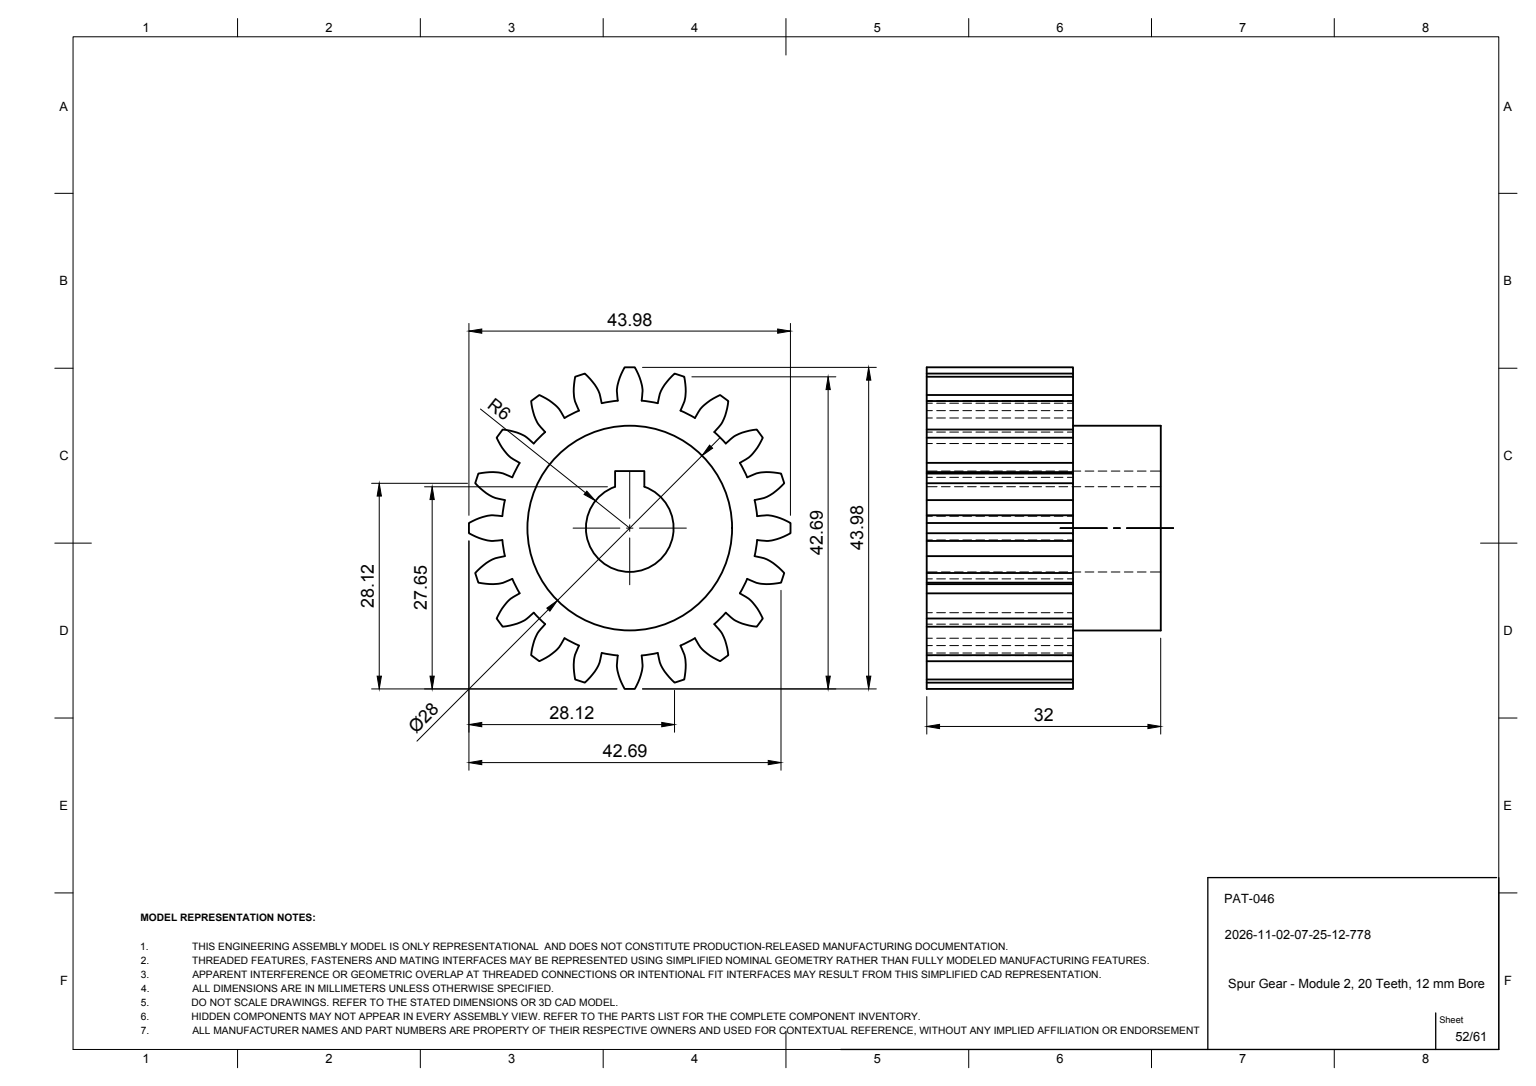
ISO-10303-21;
HEADER;
/* Generated by software containing ST-Developer
 * from STEP Tools, Inc. (www.steptools.com) 
 */

FILE_DESCRIPTION(
/* description */ ('Gear mesh backlash fixture'),
/* implementation_level */ '2;1');

FILE_NAME(
/* name */ 'Spur Gear - Module 2, 20 Teeth, 12 mm Bore.step',
/* time_stamp */ '2026-10-28T03:26:00-07:00',
/* author */ (''),
/* organization */ (''),
/* preprocessor_version */ 'ST-DEVELOPER v20.2',
/* originating_system */ 'Autodesk Translation Framework v15.17.0.0',
/* authorisation */ '');

FILE_SCHEMA (('AUTOMOTIVE_DESIGN { 1 0 10303 214 3 1 1 }'));
ENDSEC;

DATA;
#10=MECHANICAL_DESIGN_GEOMETRIC_PRESENTATION_REPRESENTATION('',(#1071),#57900);
#11=(
BOUNDED_SURFACE()
B_SPLINE_SURFACE(5,1,((#25176,#25177),(#25178,#25179),(#25180,#25181),(#25182,
#25183),(#25184,#25185),(#25186,#25187),(#25188,#25189),(#25190,#25191),
(#25192,#25193),(#25194,#25195),(#25196,#25197),(#25198,#25199),(#25200,
#25201),(#25202,#25203),(#25204,#25205),(#25206,#25207),(#25208,#25209),
(#25210,#25211),(#25212,#25213),(#25214,#25215),(#25216,#25217),(#25218,
#25219),(#25220,#25221),(#25222,#25223),(#25224,#25225),(#25226,#25227),
(#25228,#25229),(#25230,#25231),(#25232,#25233),(#25234,#25235),(#25236,
#25237),(#25238,#25239),(#25240,#25241),(#25242,#25243),(#25244,#25245),
(#25246,#25247),(#25248,#25249),(#25250,#25251),(#25252,#25253),(#25254,
#25255),(#25256,#25257),(#25258,#25259),(#25260,#25261),(#25262,#25263),
(#25264,#25265),(#25266,#25267),(#25268,#25269),(#25270,#25271),(#25272,
#25273),(#25274,#25275),(#25276,#25277),(#25278,#25279),(#25280,#25281),
(#25282,#25283),(#25284,#25285),(#25286,#25287),(#25288,#25289),(#25290,
#25291),(#25292,#25293),(#25294,#25295),(#25296,#25297),(#25298,#25299),
(#25300,#25301),(#25302,#25303),(#25304,#25305),(#25306,#25307),(#25308,
#25309),(#25310,#25311),(#25312,#25313),(#25314,#25315)),.UNSPECIFIED.,
 .F.,.F.,.F.)
B_SPLINE_SURFACE_WITH_KNOTS((6,1,1,1,1,1,1,1,1,1,1,1,1,1,1,1,1,1,1,1,1,
1,1,1,1,1,1,1,1,1,1,1,1,1,1,1,1,1,1,1,1,1,1,1,1,1,1,1,1,1,1,1,1,1,1,1,1,
1,1,1,1,1,1,1,1,6),(2,2),(-1.,-0.984615384615383,-0.969230769230768,-0.953846153846152,
-0.938461538461537,-0.923076923076922,-0.907692307692306,-0.892307692307691,
-0.876923076923076,-0.86153846153846,-0.846153846153845,-0.83076923076923,
-0.815384615384614,-0.799999999999999,-0.784615384615384,-0.769230769230768,
-0.753846153846153,-0.738461538461538,-0.723076923076922,-0.707692307692307,
-0.692307692307692,-0.676923076923076,-0.661538461538461,-0.646153846153846,
-0.63076923076923,-0.615384615384615,-0.6,-0.584615384615384,-0.569230769230769,
-0.553846153846154,-0.538461538461538,-0.523076923076923,-0.507692307692308,
-0.492307692307692,-0.476923076923077,-0.461538461538462,-0.446153846153846,
-0.430769230769231,-0.415384615384615,-0.4,-0.384615384615385,-0.369230769230769,
-0.353846153846154,-0.338461538461538,-0.323076923076923,-0.307692307692308,
-0.292307692307692,-0.276923076923077,-0.261538461538462,-0.246153846153846,
-0.230769230769231,-0.215384615384615,-0.2,-0.184615384615385,-0.169230769230769,
-0.153846153846154,-0.138461538461538,-0.123076923076923,-0.107692307692308,
-0.0923076923076923,-0.0769230769230769,-0.0615384615384615,-0.0461538461538462,
-0.0307692307692308,-0.0153846153846154,0.),(-1.,1.),.UNSPECIFIED.)
GEOMETRIC_REPRESENTATION_ITEM()
RATIONAL_B_SPLINE_SURFACE(((1.,1.),(1.,1.),(1.,1.),(1.,1.),(1.,1.),(1.,
1.),(1.,1.),(1.,1.),(1.,1.),(1.,1.),(1.,1.),(1.,1.),(1.,1.),(1.,1.),(1.,
1.),(1.,1.),(1.,1.),(1.,1.),(1.,1.),(1.,1.),(1.,1.),(1.,1.),(1.,1.),(1.,
1.),(1.,1.),(1.,1.),(1.,1.),(1.,1.),(1.,1.),(1.,1.),(1.,1.),(1.,1.),(1.,
1.),(1.,1.),(1.,1.),(1.,1.),(1.,1.),(1.,1.),(1.,1.),(1.,1.),(1.,1.),(1.,
1.),(1.,1.),(1.,1.),(1.,1.),(1.,1.),(1.,1.),(1.,1.),(1.,1.),(1.,1.),(1.,
1.),(1.,1.),(1.,1.),(1.,1.),(1.,1.),(1.,1.),(1.,1.),(1.,1.),(1.,1.),(1.,
1.),(1.,1.),(1.,1.),(1.,1.),(1.,1.),(1.,1.),(1.,1.),(1.,1.),(1.,1.),(1.,
1.),(1.,1.)))
REPRESENTATION_ITEM('')
SURFACE()
);
#12=(
BOUNDED_SURFACE()
B_SPLINE_SURFACE(5,1,((#25394,#25395),(#25396,#25397),(#25398,#25399),(#25400,
#25401),(#25402,#25403),(#25404,#25405),(#25406,#25407),(#25408,#25409),
(#25410,#25411),(#25412,#25413),(#25414,#25415),(#25416,#25417),(#25418,
#25419),(#25420,#25421),(#25422,#25423),(#25424,#25425),(#25426,#25427),
(#25428,#25429),(#25430,#25431),(#25432,#25433),(#25434,#25435),(#25436,
#25437),(#25438,#25439),(#25440,#25441),(#25442,#25443),(#25444,#25445),
(#25446,#25447),(#25448,#25449),(#25450,#25451),(#25452,#25453),(#25454,
#25455),(#25456,#25457),(#25458,#25459),(#25460,#25461),(#25462,#25463),
(#25464,#25465),(#25466,#25467),(#25468,#25469),(#25470,#25471),(#25472,
#25473),(#25474,#25475),(#25476,#25477),(#25478,#25479),(#25480,#25481),
(#25482,#25483),(#25484,#25485),(#25486,#25487),(#25488,#25489),(#25490,
#25491),(#25492,#25493),(#25494,#25495),(#25496,#25497),(#25498,#25499),
(#25500,#25501),(#25502,#25503),(#25504,#25505),(#25506,#25507),(#25508,
#25509),(#25510,#25511),(#25512,#25513),(#25514,#25515),(#25516,#25517),
(#25518,#25519),(#25520,#25521),(#25522,#25523),(#25524,#25525),(#25526,
#25527),(#25528,#25529),(#25530,#25531),(#25532,#25533)),.UNSPECIFIED.,
 .F.,.F.,.F.)
B_SPLINE_SURFACE_WITH_KNOTS((6,1,1,1,1,1,1,1,1,1,1,1,1,1,1,1,1,1,1,1,1,
1,1,1,1,1,1,1,1,1,1,1,1,1,1,1,1,1,1,1,1,1,1,1,1,1,1,1,1,1,1,1,1,1,1,1,1,
1,1,1,1,1,1,1,1,6),(2,2),(-1.,-0.984615384615383,-0.969230769230768,-0.953846153846152,
-0.938461538461537,-0.923076923076922,-0.907692307692306,-0.892307692307691,
-0.876923076923076,-0.86153846153846,-0.846153846153845,-0.83076923076923,
-0.815384615384614,-0.799999999999999,-0.784615384615384,-0.769230769230768,
-0.753846153846153,-0.738461538461538,-0.723076923076922,-0.707692307692307,
-0.692307692307692,-0.676923076923076,-0.661538461538461,-0.646153846153846,
-0.63076923076923,-0.615384615384615,-0.6,-0.584615384615384,-0.569230769230769,
-0.553846153846154,-0.538461538461538,-0.523076923076923,-0.507692307692308,
-0.492307692307692,-0.476923076923077,-0.461538461538462,-0.446153846153846,
-0.430769230769231,-0.415384615384615,-0.4,-0.384615384615385,-0.369230769230769,
-0.353846153846154,-0.338461538461538,-0.323076923076923,-0.307692307692308,
-0.292307692307692,-0.276923076923077,-0.261538461538462,-0.246153846153846,
-0.230769230769231,-0.215384615384615,-0.2,-0.184615384615385,-0.169230769230769,
-0.153846153846154,-0.138461538461538,-0.123076923076923,-0.107692307692308,
-0.0923076923076923,-0.0769230769230769,-0.0615384615384615,-0.0461538461538462,
-0.0307692307692308,-0.0153846153846154,0.),(-1.,1.),.UNSPECIFIED.)
GEOMETRIC_REPRESENTATION_ITEM()
RATIONAL_B_SPLINE_SURFACE(((1.,1.),(1.,1.),(1.,1.),(1.,1.),(1.,1.),(1.,
1.),(1.,1.),(1.,1.),(1.,1.),(1.,1.),(1.,1.),(1.,1.),(1.,1.),(1.,1.),(1.,
1.),(1.,1.),(1.,1.),(1.,1.),(1.,1.),(1.,1.),(1.,1.),(1.,1.),(1.,1.),(1.,
1.),(1.,1.),(1.,1.),(1.,1.),(1.,1.),(1.,1.),(1.,1.),(1.,1.),(1.,1.),(1.,
1.),(1.,1.),(1.,1.),(1.,1.),(1.,1.),(1.,1.),(1.,1.),(1.,1.),(1.,1.),(1.,
1.),(1.,1.),(1.,1.),(1.,1.),(1.,1.),(1.,1.),(1.,1.),(1.,1.),(1.,1.),(1.,
1.),(1.,1.),(1.,1.),(1.,1.),(1.,1.),(1.,1.),(1.,1.),(1.,1.),(1.,1.),(1.,
1.),(1.,1.),(1.,1.),(1.,1.),(1.,1.),(1.,1.),(1.,1.),(1.,1.),(1.,1.),(1.,
1.),(1.,1.)))
REPRESENTATION_ITEM('')
SURFACE()
);
#13=(
BOUNDED_SURFACE()
B_SPLINE_SURFACE(5,1,((#25610,#25611),(#25612,#25613),(#25614,#25615),(#25616,
#25617),(#25618,#25619),(#25620,#25621),(#25622,#25623),(#25624,#25625),
(#25626,#25627),(#25628,#25629),(#25630,#25631),(#25632,#25633),(#25634,
#25635),(#25636,#25637),(#25638,#25639),(#25640,#25641),(#25642,#25643),
(#25644,#25645),(#25646,#25647),(#25648,#25649),(#25650,#25651),(#25652,
#25653),(#25654,#25655),(#25656,#25657),(#25658,#25659),(#25660,#25661),
(#25662,#25663),(#25664,#25665),(#25666,#25667),(#25668,#25669),(#25670,
#25671),(#25672,#25673),(#25674,#25675),(#25676,#25677),(#25678,#25679),
(#25680,#25681),(#25682,#25683),(#25684,#25685),(#25686,#25687),(#25688,
#25689),(#25690,#25691),(#25692,#25693),(#25694,#25695),(#25696,#25697),
(#25698,#25699),(#25700,#25701),(#25702,#25703),(#25704,#25705),(#25706,
#25707),(#25708,#25709),(#25710,#25711),(#25712,#25713),(#25714,#25715),
(#25716,#25717),(#25718,#25719),(#25720,#25721),(#25722,#25723),(#25724,
#25725),(#25726,#25727),(#25728,#25729),(#25730,#25731),(#25732,#25733),
(#25734,#25735),(#25736,#25737),(#25738,#25739),(#25740,#25741),(#25742,
#25743),(#25744,#25745),(#25746,#25747),(#25748,#25749)),.UNSPECIFIED.,
 .F.,.F.,.F.)
B_SPLINE_SURFACE_WITH_KNOTS((6,1,1,1,1,1,1,1,1,1,1,1,1,1,1,1,1,1,1,1,1,
1,1,1,1,1,1,1,1,1,1,1,1,1,1,1,1,1,1,1,1,1,1,1,1,1,1,1,1,1,1,1,1,1,1,1,1,
1,1,1,1,1,1,1,1,6),(2,2),(-1.,-0.984615384615383,-0.969230769230768,-0.953846153846152,
-0.938461538461537,-0.923076923076922,-0.907692307692306,-0.892307692307691,
-0.876923076923076,-0.86153846153846,-0.846153846153845,-0.83076923076923,
-0.815384615384614,-0.799999999999999,-0.784615384615384,-0.769230769230768,
-0.753846153846153,-0.738461538461538,-0.723076923076922,-0.707692307692307,
-0.692307692307692,-0.676923076923076,-0.661538461538461,-0.646153846153846,
-0.63076923076923,-0.615384615384615,-0.6,-0.584615384615384,-0.569230769230769,
-0.553846153846154,-0.538461538461538,-0.523076923076923,-0.507692307692308,
-0.492307692307692,-0.476923076923077,-0.461538461538462,-0.446153846153846,
-0.430769230769231,-0.415384615384615,-0.4,-0.384615384615385,-0.369230769230769,
-0.353846153846154,-0.338461538461538,-0.323076923076923,-0.307692307692308,
-0.292307692307692,-0.276923076923077,-0.261538461538462,-0.246153846153846,
-0.230769230769231,-0.215384615384615,-0.2,-0.184615384615385,-0.169230769230769,
-0.153846153846154,-0.138461538461538,-0.123076923076923,-0.107692307692308,
-0.0923076923076923,-0.0769230769230769,-0.0615384615384615,-0.0461538461538462,
-0.0307692307692308,-0.0153846153846154,0.),(-1.,1.),.UNSPECIFIED.)
GEOMETRIC_REPRESENTATION_ITEM()
RATIONAL_B_SPLINE_SURFACE(((1.,1.),(1.,1.),(1.,1.),(1.,1.),(1.,1.),(1.,
1.),(1.,1.),(1.,1.),(1.,1.),(1.,1.),(1.,1.),(1.,1.),(1.,1.),(1.,1.),(1.,
1.),(1.,1.),(1.,1.),(1.,1.),(1.,1.),(1.,1.),(1.,1.),(1.,1.),(1.,1.),(1.,
1.),(1.,1.),(1.,1.),(1.,1.),(1.,1.),(1.,1.),(1.,1.),(1.,1.),(1.,1.),(1.,
1.),(1.,1.),(1.,1.),(1.,1.),(1.,1.),(1.,1.),(1.,1.),(1.,1.),(1.,1.),(1.,
1.),(1.,1.),(1.,1.),(1.,1.),(1.,1.),(1.,1.),(1.,1.),(1.,1.),(1.,1.),(1.,
1.),(1.,1.),(1.,1.),(1.,1.),(1.,1.),(1.,1.),(1.,1.),(1.,1.),(1.,1.),(1.,
1.),(1.,1.),(1.,1.),(1.,1.),(1.,1.),(1.,1.),(1.,1.),(1.,1.),(1.,1.),(1.,
1.),(1.,1.)))
REPRESENTATION_ITEM('')
SURFACE()
);
#14=(
BOUNDED_SURFACE()
B_SPLINE_SURFACE(5,1,((#25826,#25827),(#25828,#25829),(#25830,#25831),(#25832,
#25833),(#25834,#25835),(#25836,#25837),(#25838,#25839),(#25840,#25841),
(#25842,#25843),(#25844,#25845),(#25846,#25847),(#25848,#25849),(#25850,
#25851),(#25852,#25853),(#25854,#25855),(#25856,#25857),(#25858,#25859),
(#25860,#25861),(#25862,#25863),(#25864,#25865),(#25866,#25867),(#25868,
#25869),(#25870,#25871),(#25872,#25873),(#25874,#25875),(#25876,#25877),
(#25878,#25879),(#25880,#25881),(#25882,#25883),(#25884,#25885),(#25886,
#25887),(#25888,#25889),(#25890,#25891),(#25892,#25893),(#25894,#25895),
(#25896,#25897),(#25898,#25899),(#25900,#25901),(#25902,#25903),(#25904,
#25905),(#25906,#25907),(#25908,#25909),(#25910,#25911),(#25912,#25913),
(#25914,#25915),(#25916,#25917),(#25918,#25919),(#25920,#25921),(#25922,
#25923),(#25924,#25925),(#25926,#25927),(#25928,#25929),(#25930,#25931),
(#25932,#25933),(#25934,#25935),(#25936,#25937),(#25938,#25939),(#25940,
#25941),(#25942,#25943),(#25944,#25945),(#25946,#25947),(#25948,#25949),
(#25950,#25951),(#25952,#25953),(#25954,#25955),(#25956,#25957),(#25958,
#25959),(#25960,#25961),(#25962,#25963),(#25964,#25965)),.UNSPECIFIED.,
 .F.,.F.,.F.)
B_SPLINE_SURFACE_WITH_KNOTS((6,1,1,1,1,1,1,1,1,1,1,1,1,1,1,1,1,1,1,1,1,
1,1,1,1,1,1,1,1,1,1,1,1,1,1,1,1,1,1,1,1,1,1,1,1,1,1,1,1,1,1,1,1,1,1,1,1,
1,1,1,1,1,1,1,1,6),(2,2),(-1.,-0.984615384615383,-0.969230769230768,-0.953846153846152,
-0.938461538461537,-0.923076923076922,-0.907692307692306,-0.892307692307691,
-0.876923076923076,-0.86153846153846,-0.846153846153845,-0.83076923076923,
-0.815384615384614,-0.799999999999999,-0.784615384615384,-0.769230769230768,
-0.753846153846153,-0.738461538461538,-0.723076923076922,-0.707692307692307,
-0.692307692307692,-0.676923076923076,-0.661538461538461,-0.646153846153846,
-0.63076923076923,-0.615384615384615,-0.6,-0.584615384615384,-0.569230769230769,
-0.553846153846154,-0.538461538461538,-0.523076923076923,-0.507692307692308,
-0.492307692307692,-0.476923076923077,-0.461538461538462,-0.446153846153846,
-0.430769230769231,-0.415384615384615,-0.4,-0.384615384615385,-0.369230769230769,
-0.353846153846154,-0.338461538461538,-0.323076923076923,-0.307692307692308,
-0.292307692307692,-0.276923076923077,-0.261538461538462,-0.246153846153846,
-0.230769230769231,-0.215384615384615,-0.2,-0.184615384615385,-0.169230769230769,
-0.153846153846154,-0.138461538461538,-0.123076923076923,-0.107692307692308,
-0.0923076923076923,-0.0769230769230769,-0.0615384615384615,-0.0461538461538462,
-0.0307692307692308,-0.0153846153846154,0.),(-1.,1.),.UNSPECIFIED.)
GEOMETRIC_REPRESENTATION_ITEM()
RATIONAL_B_SPLINE_SURFACE(((1.,1.),(1.,1.),(1.,1.),(1.,1.),(1.,1.),(1.,
1.),(1.,1.),(1.,1.),(1.,1.),(1.,1.),(1.,1.),(1.,1.),(1.,1.),(1.,1.),(1.,
1.),(1.,1.),(1.,1.),(1.,1.),(1.,1.),(1.,1.),(1.,1.),(1.,1.),(1.,1.),(1.,
1.),(1.,1.),(1.,1.),(1.,1.),(1.,1.),(1.,1.),(1.,1.),(1.,1.),(1.,1.),(1.,
1.),(1.,1.),(1.,1.),(1.,1.),(1.,1.),(1.,1.),(1.,1.),(1.,1.),(1.,1.),(1.,
1.),(1.,1.),(1.,1.),(1.,1.),(1.,1.),(1.,1.),(1.,1.),(1.,1.),(1.,1.),(1.,
1.),(1.,1.),(1.,1.),(1.,1.),(1.,1.),(1.,1.),(1.,1.),(1.,1.),(1.,1.),(1.,
1.),(1.,1.),(1.,1.),(1.,1.),(1.,1.),(1.,1.),(1.,1.),(1.,1.),(1.,1.),(1.,
1.),(1.,1.)))
REPRESENTATION_ITEM('')
SURFACE()
);
#15=(
BOUNDED_SURFACE()
B_SPLINE_SURFACE(5,1,((#26042,#26043),(#26044,#26045),(#26046,#26047),(#26048,
#26049),(#26050,#26051),(#26052,#26053),(#26054,#26055),(#26056,#26057),
(#26058,#26059),(#26060,#26061),(#26062,#26063),(#26064,#26065),(#26066,
#26067),(#26068,#26069),(#26070,#26071),(#26072,#26073),(#26074,#26075),
(#26076,#26077),(#26078,#26079),(#26080,#26081),(#26082,#26083),(#26084,
#26085),(#26086,#26087),(#26088,#26089),(#26090,#26091),(#26092,#26093),
(#26094,#26095),(#26096,#26097),(#26098,#26099),(#26100,#26101),(#26102,
#26103),(#26104,#26105),(#26106,#26107),(#26108,#26109),(#26110,#26111),
(#26112,#26113),(#26114,#26115),(#26116,#26117),(#26118,#26119),(#26120,
#26121),(#26122,#26123),(#26124,#26125),(#26126,#26127),(#26128,#26129),
(#26130,#26131),(#26132,#26133),(#26134,#26135),(#26136,#26137),(#26138,
#26139),(#26140,#26141),(#26142,#26143),(#26144,#26145),(#26146,#26147),
(#26148,#26149),(#26150,#26151),(#26152,#26153),(#26154,#26155),(#26156,
#26157),(#26158,#26159),(#26160,#26161),(#26162,#26163),(#26164,#26165),
(#26166,#26167),(#26168,#26169),(#26170,#26171),(#26172,#26173),(#26174,
#26175),(#26176,#26177),(#26178,#26179),(#26180,#26181)),.UNSPECIFIED.,
 .F.,.F.,.F.)
B_SPLINE_SURFACE_WITH_KNOTS((6,1,1,1,1,1,1,1,1,1,1,1,1,1,1,1,1,1,1,1,1,
1,1,1,1,1,1,1,1,1,1,1,1,1,1,1,1,1,1,1,1,1,1,1,1,1,1,1,1,1,1,1,1,1,1,1,1,
1,1,1,1,1,1,1,1,6),(2,2),(-1.,-0.984615384615383,-0.969230769230768,-0.953846153846152,
-0.938461538461537,-0.923076923076922,-0.907692307692306,-0.892307692307691,
-0.876923076923076,-0.86153846153846,-0.846153846153845,-0.83076923076923,
-0.815384615384614,-0.799999999999999,-0.784615384615384,-0.769230769230768,
-0.753846153846153,-0.738461538461538,-0.723076923076922,-0.707692307692307,
-0.692307692307692,-0.676923076923076,-0.661538461538461,-0.646153846153846,
-0.63076923076923,-0.615384615384615,-0.6,-0.584615384615384,-0.569230769230769,
-0.553846153846154,-0.538461538461538,-0.523076923076923,-0.507692307692308,
-0.492307692307692,-0.476923076923077,-0.461538461538462,-0.446153846153846,
-0.430769230769231,-0.415384615384615,-0.4,-0.384615384615385,-0.369230769230769,
-0.353846153846154,-0.338461538461538,-0.323076923076923,-0.307692307692308,
-0.292307692307692,-0.276923076923077,-0.261538461538462,-0.246153846153846,
-0.230769230769231,-0.215384615384615,-0.2,-0.184615384615385,-0.169230769230769,
-0.153846153846154,-0.138461538461538,-0.123076923076923,-0.107692307692308,
-0.0923076923076923,-0.0769230769230769,-0.0615384615384615,-0.0461538461538462,
-0.0307692307692308,-0.0153846153846154,0.),(-1.,1.),.UNSPECIFIED.)
GEOMETRIC_REPRESENTATION_ITEM()
RATIONAL_B_SPLINE_SURFACE(((1.,1.),(1.,1.),(1.,1.),(1.,1.),(1.,1.),(1.,
1.),(1.,1.),(1.,1.),(1.,1.),(1.,1.),(1.,1.),(1.,1.),(1.,1.),(1.,1.),(1.,
1.),(1.,1.),(1.,1.),(1.,1.),(1.,1.),(1.,1.),(1.,1.),(1.,1.),(1.,1.),(1.,
1.),(1.,1.),(1.,1.),(1.,1.),(1.,1.),(1.,1.),(1.,1.),(1.,1.),(1.,1.),(1.,
1.),(1.,1.),(1.,1.),(1.,1.),(1.,1.),(1.,1.),(1.,1.),(1.,1.),(1.,1.),(1.,
1.),(1.,1.),(1.,1.),(1.,1.),(1.,1.),(1.,1.),(1.,1.),(1.,1.),(1.,1.),(1.,
1.),(1.,1.),(1.,1.),(1.,1.),(1.,1.),(1.,1.),(1.,1.),(1.,1.),(1.,1.),(1.,
1.),(1.,1.),(1.,1.),(1.,1.),(1.,1.),(1.,1.),(1.,1.),(1.,1.),(1.,1.),(1.,
1.),(1.,1.)))
REPRESENTATION_ITEM('')
SURFACE()
);
#16=(
BOUNDED_SURFACE()
B_SPLINE_SURFACE(5,1,((#26258,#26259),(#26260,#26261),(#26262,#26263),(#26264,
#26265),(#26266,#26267),(#26268,#26269),(#26270,#26271),(#26272,#26273),
(#26274,#26275),(#26276,#26277),(#26278,#26279),(#26280,#26281),(#26282,
#26283),(#26284,#26285),(#26286,#26287),(#26288,#26289),(#26290,#26291),
(#26292,#26293),(#26294,#26295),(#26296,#26297),(#26298,#26299),(#26300,
#26301),(#26302,#26303),(#26304,#26305),(#26306,#26307),(#26308,#26309),
(#26310,#26311),(#26312,#26313),(#26314,#26315),(#26316,#26317),(#26318,
#26319),(#26320,#26321),(#26322,#26323),(#26324,#26325),(#26326,#26327),
(#26328,#26329),(#26330,#26331),(#26332,#26333),(#26334,#26335),(#26336,
#26337),(#26338,#26339),(#26340,#26341),(#26342,#26343),(#26344,#26345),
(#26346,#26347),(#26348,#26349),(#26350,#26351),(#26352,#26353),(#26354,
#26355),(#26356,#26357),(#26358,#26359),(#26360,#26361),(#26362,#26363),
(#26364,#26365),(#26366,#26367),(#26368,#26369),(#26370,#26371),(#26372,
#26373),(#26374,#26375),(#26376,#26377),(#26378,#26379),(#26380,#26381),
(#26382,#26383),(#26384,#26385),(#26386,#26387),(#26388,#26389),(#26390,
#26391),(#26392,#26393),(#26394,#26395),(#26396,#26397)),.UNSPECIFIED.,
 .F.,.F.,.F.)
B_SPLINE_SURFACE_WITH_KNOTS((6,1,1,1,1,1,1,1,1,1,1,1,1,1,1,1,1,1,1,1,1,
1,1,1,1,1,1,1,1,1,1,1,1,1,1,1,1,1,1,1,1,1,1,1,1,1,1,1,1,1,1,1,1,1,1,1,1,
1,1,1,1,1,1,1,1,6),(2,2),(-1.,-0.984615384615383,-0.969230769230768,-0.953846153846152,
-0.938461538461537,-0.923076923076922,-0.907692307692306,-0.892307692307691,
-0.876923076923076,-0.86153846153846,-0.846153846153845,-0.83076923076923,
-0.815384615384614,-0.799999999999999,-0.784615384615384,-0.769230769230768,
-0.753846153846153,-0.738461538461538,-0.723076923076922,-0.707692307692307,
-0.692307692307692,-0.676923076923076,-0.661538461538461,-0.646153846153846,
-0.63076923076923,-0.615384615384615,-0.6,-0.584615384615384,-0.569230769230769,
-0.553846153846154,-0.538461538461538,-0.523076923076923,-0.507692307692308,
-0.492307692307692,-0.476923076923077,-0.461538461538462,-0.446153846153846,
-0.430769230769231,-0.415384615384615,-0.4,-0.384615384615385,-0.369230769230769,
-0.353846153846154,-0.338461538461538,-0.323076923076923,-0.307692307692308,
-0.292307692307692,-0.276923076923077,-0.261538461538462,-0.246153846153846,
-0.230769230769231,-0.215384615384615,-0.2,-0.184615384615385,-0.169230769230769,
-0.153846153846154,-0.138461538461538,-0.123076923076923,-0.107692307692308,
-0.0923076923076923,-0.0769230769230769,-0.0615384615384615,-0.0461538461538462,
-0.0307692307692308,-0.0153846153846154,0.),(-1.,1.),.UNSPECIFIED.)
GEOMETRIC_REPRESENTATION_ITEM()
RATIONAL_B_SPLINE_SURFACE(((1.,1.),(1.,1.),(1.,1.),(1.,1.),(1.,1.),(1.,
1.),(1.,1.),(1.,1.),(1.,1.),(1.,1.),(1.,1.),(1.,1.),(1.,1.),(1.,1.),(1.,
1.),(1.,1.),(1.,1.),(1.,1.),(1.,1.),(1.,1.),(1.,1.),(1.,1.),(1.,1.),(1.,
1.),(1.,1.),(1.,1.),(1.,1.),(1.,1.),(1.,1.),(1.,1.),(1.,1.),(1.,1.),(1.,
1.),(1.,1.),(1.,1.),(1.,1.),(1.,1.),(1.,1.),(1.,1.),(1.,1.),(1.,1.),(1.,
1.),(1.,1.),(1.,1.),(1.,1.),(1.,1.),(1.,1.),(1.,1.),(1.,1.),(1.,1.),(1.,
1.),(1.,1.),(1.,1.),(1.,1.),(1.,1.),(1.,1.),(1.,1.),(1.,1.),(1.,1.),(1.,
1.),(1.,1.),(1.,1.),(1.,1.),(1.,1.),(1.,1.),(1.,1.),(1.,1.),(1.,1.),(1.,
1.),(1.,1.)))
REPRESENTATION_ITEM('')
SURFACE()
);
#17=(
BOUNDED_SURFACE()
B_SPLINE_SURFACE(5,1,((#26474,#26475),(#26476,#26477),(#26478,#26479),(#26480,
#26481),(#26482,#26483),(#26484,#26485),(#26486,#26487),(#26488,#26489),
(#26490,#26491),(#26492,#26493),(#26494,#26495),(#26496,#26497),(#26498,
#26499),(#26500,#26501),(#26502,#26503),(#26504,#26505),(#26506,#26507),
(#26508,#26509),(#26510,#26511),(#26512,#26513),(#26514,#26515),(#26516,
#26517),(#26518,#26519),(#26520,#26521),(#26522,#26523),(#26524,#26525),
(#26526,#26527),(#26528,#26529),(#26530,#26531),(#26532,#26533),(#26534,
#26535),(#26536,#26537),(#26538,#26539),(#26540,#26541),(#26542,#26543),
(#26544,#26545),(#26546,#26547),(#26548,#26549),(#26550,#26551),(#26552,
#26553),(#26554,#26555),(#26556,#26557),(#26558,#26559),(#26560,#26561),
(#26562,#26563),(#26564,#26565),(#26566,#26567),(#26568,#26569),(#26570,
#26571),(#26572,#26573),(#26574,#26575),(#26576,#26577),(#26578,#26579),
(#26580,#26581),(#26582,#26583),(#26584,#26585),(#26586,#26587),(#26588,
#26589),(#26590,#26591),(#26592,#26593),(#26594,#26595),(#26596,#26597),
(#26598,#26599),(#26600,#26601),(#26602,#26603),(#26604,#26605),(#26606,
#26607),(#26608,#26609),(#26610,#26611),(#26612,#26613)),.UNSPECIFIED.,
 .F.,.F.,.F.)
B_SPLINE_SURFACE_WITH_KNOTS((6,1,1,1,1,1,1,1,1,1,1,1,1,1,1,1,1,1,1,1,1,
1,1,1,1,1,1,1,1,1,1,1,1,1,1,1,1,1,1,1,1,1,1,1,1,1,1,1,1,1,1,1,1,1,1,1,1,
1,1,1,1,1,1,1,1,6),(2,2),(-1.,-0.984615384615383,-0.969230769230768,-0.953846153846152,
-0.938461538461537,-0.923076923076922,-0.907692307692306,-0.892307692307691,
-0.876923076923076,-0.86153846153846,-0.846153846153845,-0.83076923076923,
-0.815384615384614,-0.799999999999999,-0.784615384615384,-0.769230769230768,
-0.753846153846153,-0.738461538461538,-0.723076923076922,-0.707692307692307,
-0.692307692307692,-0.676923076923076,-0.661538461538461,-0.646153846153846,
-0.63076923076923,-0.615384615384615,-0.6,-0.584615384615384,-0.569230769230769,
-0.553846153846154,-0.538461538461538,-0.523076923076923,-0.507692307692308,
-0.492307692307692,-0.476923076923077,-0.461538461538462,-0.446153846153846,
-0.430769230769231,-0.415384615384615,-0.4,-0.384615384615385,-0.369230769230769,
-0.353846153846154,-0.338461538461538,-0.323076923076923,-0.307692307692308,
-0.292307692307692,-0.276923076923077,-0.261538461538462,-0.246153846153846,
-0.230769230769231,-0.215384615384615,-0.2,-0.184615384615385,-0.169230769230769,
-0.153846153846154,-0.138461538461538,-0.123076923076923,-0.107692307692308,
-0.0923076923076923,-0.0769230769230769,-0.0615384615384615,-0.0461538461538462,
-0.0307692307692308,-0.0153846153846154,0.),(-1.,1.),.UNSPECIFIED.)
GEOMETRIC_REPRESENTATION_ITEM()
RATIONAL_B_SPLINE_SURFACE(((1.,1.),(1.,1.),(1.,1.),(1.,1.),(1.,1.),(1.,
1.),(1.,1.),(1.,1.),(1.,1.),(1.,1.),(1.,1.),(1.,1.),(1.,1.),(1.,1.),(1.,
1.),(1.,1.),(1.,1.),(1.,1.),(1.,1.),(1.,1.),(1.,1.),(1.,1.),(1.,1.),(1.,
1.),(1.,1.),(1.,1.),(1.,1.),(1.,1.),(1.,1.),(1.,1.),(1.,1.),(1.,1.),(1.,
1.),(1.,1.),(1.,1.),(1.,1.),(1.,1.),(1.,1.),(1.,1.),(1.,1.),(1.,1.),(1.,
1.),(1.,1.),(1.,1.),(1.,1.),(1.,1.),(1.,1.),(1.,1.),(1.,1.),(1.,1.),(1.,
1.),(1.,1.),(1.,1.),(1.,1.),(1.,1.),(1.,1.),(1.,1.),(1.,1.),(1.,1.),(1.,
1.),(1.,1.),(1.,1.),(1.,1.),(1.,1.),(1.,1.),(1.,1.),(1.,1.),(1.,1.),(1.,
1.),(1.,1.)))
REPRESENTATION_ITEM('')
SURFACE()
);
#18=(
BOUNDED_SURFACE()
B_SPLINE_SURFACE(5,1,((#26690,#26691),(#26692,#26693),(#26694,#26695),(#26696,
#26697),(#26698,#26699),(#26700,#26701),(#26702,#26703),(#26704,#26705),
(#26706,#26707),(#26708,#26709),(#26710,#26711),(#26712,#26713),(#26714,
#26715),(#26716,#26717),(#26718,#26719),(#26720,#26721),(#26722,#26723),
(#26724,#26725),(#26726,#26727),(#26728,#26729),(#26730,#26731),(#26732,
#26733),(#26734,#26735),(#26736,#26737),(#26738,#26739),(#26740,#26741),
(#26742,#26743),(#26744,#26745),(#26746,#26747),(#26748,#26749),(#26750,
#26751),(#26752,#26753),(#26754,#26755),(#26756,#26757),(#26758,#26759),
(#26760,#26761),(#26762,#26763),(#26764,#26765),(#26766,#26767),(#26768,
#26769),(#26770,#26771),(#26772,#26773),(#26774,#26775),(#26776,#26777),
(#26778,#26779),(#26780,#26781),(#26782,#26783),(#26784,#26785),(#26786,
#26787),(#26788,#26789),(#26790,#26791),(#26792,#26793),(#26794,#26795),
(#26796,#26797),(#26798,#26799),(#26800,#26801),(#26802,#26803),(#26804,
#26805),(#26806,#26807),(#26808,#26809),(#26810,#26811),(#26812,#26813),
(#26814,#26815),(#26816,#26817),(#26818,#26819),(#26820,#26821),(#26822,
#26823),(#26824,#26825),(#26826,#26827),(#26828,#26829)),.UNSPECIFIED.,
 .F.,.F.,.F.)
B_SPLINE_SURFACE_WITH_KNOTS((6,1,1,1,1,1,1,1,1,1,1,1,1,1,1,1,1,1,1,1,1,
1,1,1,1,1,1,1,1,1,1,1,1,1,1,1,1,1,1,1,1,1,1,1,1,1,1,1,1,1,1,1,1,1,1,1,1,
1,1,1,1,1,1,1,1,6),(2,2),(-1.,-0.984615384615383,-0.969230769230768,-0.953846153846152,
-0.938461538461537,-0.923076923076922,-0.907692307692306,-0.892307692307691,
-0.876923076923076,-0.86153846153846,-0.846153846153845,-0.83076923076923,
-0.815384615384614,-0.799999999999999,-0.784615384615384,-0.769230769230768,
-0.753846153846153,-0.738461538461538,-0.723076923076922,-0.707692307692307,
-0.692307692307692,-0.676923076923076,-0.661538461538461,-0.646153846153846,
-0.63076923076923,-0.615384615384615,-0.6,-0.584615384615384,-0.569230769230769,
-0.553846153846154,-0.538461538461538,-0.523076923076923,-0.507692307692308,
-0.492307692307692,-0.476923076923077,-0.461538461538462,-0.446153846153846,
-0.430769230769231,-0.415384615384615,-0.4,-0.384615384615385,-0.369230769230769,
-0.353846153846154,-0.338461538461538,-0.323076923076923,-0.307692307692308,
-0.292307692307692,-0.276923076923077,-0.261538461538462,-0.246153846153846,
-0.230769230769231,-0.215384615384615,-0.2,-0.184615384615385,-0.169230769230769,
-0.153846153846154,-0.138461538461538,-0.123076923076923,-0.107692307692308,
-0.0923076923076923,-0.0769230769230769,-0.0615384615384615,-0.0461538461538462,
-0.0307692307692308,-0.0153846153846154,0.),(-1.,1.),.UNSPECIFIED.)
GEOMETRIC_REPRESENTATION_ITEM()
RATIONAL_B_SPLINE_SURFACE(((1.,1.),(1.,1.),(1.,1.),(1.,1.),(1.,1.),(1.,
1.),(1.,1.),(1.,1.),(1.,1.),(1.,1.),(1.,1.),(1.,1.),(1.,1.),(1.,1.),(1.,
1.),(1.,1.),(1.,1.),(1.,1.),(1.,1.),(1.,1.),(1.,1.),(1.,1.),(1.,1.),(1.,
1.),(1.,1.),(1.,1.),(1.,1.),(1.,1.),(1.,1.),(1.,1.),(1.,1.),(1.,1.),(1.,
1.),(1.,1.),(1.,1.),(1.,1.),(1.,1.),(1.,1.),(1.,1.),(1.,1.),(1.,1.),(1.,
1.),(1.,1.),(1.,1.),(1.,1.),(1.,1.),(1.,1.),(1.,1.),(1.,1.),(1.,1.),(1.,
1.),(1.,1.),(1.,1.),(1.,1.),(1.,1.),(1.,1.),(1.,1.),(1.,1.),(1.,1.),(1.,
1.),(1.,1.),(1.,1.),(1.,1.),(1.,1.),(1.,1.),(1.,1.),(1.,1.),(1.,1.),(1.,
1.),(1.,1.)))
REPRESENTATION_ITEM('')
SURFACE()
);
#19=(
BOUNDED_SURFACE()
B_SPLINE_SURFACE(5,1,((#26906,#26907),(#26908,#26909),(#26910,#26911),(#26912,
#26913),(#26914,#26915),(#26916,#26917),(#26918,#26919),(#26920,#26921),
(#26922,#26923),(#26924,#26925),(#26926,#26927),(#26928,#26929),(#26930,
#26931),(#26932,#26933),(#26934,#26935),(#26936,#26937),(#26938,#26939),
(#26940,#26941),(#26942,#26943),(#26944,#26945),(#26946,#26947),(#26948,
#26949),(#26950,#26951),(#26952,#26953),(#26954,#26955),(#26956,#26957),
(#26958,#26959),(#26960,#26961),(#26962,#26963),(#26964,#26965),(#26966,
#26967),(#26968,#26969),(#26970,#26971),(#26972,#26973),(#26974,#26975),
(#26976,#26977),(#26978,#26979),(#26980,#26981),(#26982,#26983),(#26984,
#26985),(#26986,#26987),(#26988,#26989),(#26990,#26991),(#26992,#26993),
(#26994,#26995),(#26996,#26997),(#26998,#26999),(#27000,#27001),(#27002,
#27003),(#27004,#27005),(#27006,#27007),(#27008,#27009),(#27010,#27011),
(#27012,#27013),(#27014,#27015),(#27016,#27017),(#27018,#27019),(#27020,
#27021),(#27022,#27023),(#27024,#27025),(#27026,#27027),(#27028,#27029),
(#27030,#27031),(#27032,#27033),(#27034,#27035),(#27036,#27037),(#27038,
#27039),(#27040,#27041),(#27042,#27043),(#27044,#27045)),.UNSPECIFIED.,
 .F.,.F.,.F.)
B_SPLINE_SURFACE_WITH_KNOTS((6,1,1,1,1,1,1,1,1,1,1,1,1,1,1,1,1,1,1,1,1,
1,1,1,1,1,1,1,1,1,1,1,1,1,1,1,1,1,1,1,1,1,1,1,1,1,1,1,1,1,1,1,1,1,1,1,1,
1,1,1,1,1,1,1,1,6),(2,2),(-1.,-0.984615384615383,-0.969230769230768,-0.953846153846152,
-0.938461538461537,-0.923076923076922,-0.907692307692306,-0.892307692307691,
-0.876923076923076,-0.86153846153846,-0.846153846153845,-0.83076923076923,
-0.815384615384614,-0.799999999999999,-0.784615384615384,-0.769230769230768,
-0.753846153846153,-0.738461538461538,-0.723076923076922,-0.707692307692307,
-0.692307692307692,-0.676923076923076,-0.661538461538461,-0.646153846153846,
-0.63076923076923,-0.615384615384615,-0.6,-0.584615384615384,-0.569230769230769,
-0.553846153846154,-0.538461538461538,-0.523076923076923,-0.507692307692308,
-0.492307692307692,-0.476923076923077,-0.461538461538462,-0.446153846153846,
-0.430769230769231,-0.415384615384615,-0.4,-0.384615384615385,-0.369230769230769,
-0.353846153846154,-0.338461538461538,-0.323076923076923,-0.307692307692308,
-0.292307692307692,-0.276923076923077,-0.261538461538462,-0.246153846153846,
-0.230769230769231,-0.215384615384615,-0.2,-0.184615384615385,-0.169230769230769,
-0.153846153846154,-0.138461538461538,-0.123076923076923,-0.107692307692308,
-0.0923076923076923,-0.0769230769230769,-0.0615384615384615,-0.0461538461538462,
-0.0307692307692308,-0.0153846153846154,0.),(-1.,1.),.UNSPECIFIED.)
GEOMETRIC_REPRESENTATION_ITEM()
RATIONAL_B_SPLINE_SURFACE(((1.,1.),(1.,1.),(1.,1.),(1.,1.),(1.,1.),(1.,
1.),(1.,1.),(1.,1.),(1.,1.),(1.,1.),(1.,1.),(1.,1.),(1.,1.),(1.,1.),(1.,
1.),(1.,1.),(1.,1.),(1.,1.),(1.,1.),(1.,1.),(1.,1.),(1.,1.),(1.,1.),(1.,
1.),(1.,1.),(1.,1.),(1.,1.),(1.,1.),(1.,1.),(1.,1.),(1.,1.),(1.,1.),(1.,
1.),(1.,1.),(1.,1.),(1.,1.),(1.,1.),(1.,1.),(1.,1.),(1.,1.),(1.,1.),(1.,
1.),(1.,1.),(1.,1.),(1.,1.),(1.,1.),(1.,1.),(1.,1.),(1.,1.),(1.,1.),(1.,
1.),(1.,1.),(1.,1.),(1.,1.),(1.,1.),(1.,1.),(1.,1.),(1.,1.),(1.,1.),(1.,
1.),(1.,1.),(1.,1.),(1.,1.),(1.,1.),(1.,1.),(1.,1.),(1.,1.),(1.,1.),(1.,
1.),(1.,1.)))
REPRESENTATION_ITEM('')
SURFACE()
);
#20=(
BOUNDED_SURFACE()
B_SPLINE_SURFACE(5,1,((#27122,#27123),(#27124,#27125),(#27126,#27127),(#27128,
#27129),(#27130,#27131),(#27132,#27133),(#27134,#27135),(#27136,#27137),
(#27138,#27139),(#27140,#27141),(#27142,#27143),(#27144,#27145),(#27146,
#27147),(#27148,#27149),(#27150,#27151),(#27152,#27153),(#27154,#27155),
(#27156,#27157),(#27158,#27159),(#27160,#27161),(#27162,#27163),(#27164,
#27165),(#27166,#27167),(#27168,#27169),(#27170,#27171),(#27172,#27173),
(#27174,#27175),(#27176,#27177),(#27178,#27179),(#27180,#27181),(#27182,
#27183),(#27184,#27185),(#27186,#27187),(#27188,#27189),(#27190,#27191),
(#27192,#27193),(#27194,#27195),(#27196,#27197),(#27198,#27199),(#27200,
#27201),(#27202,#27203),(#27204,#27205),(#27206,#27207),(#27208,#27209),
(#27210,#27211),(#27212,#27213),(#27214,#27215),(#27216,#27217),(#27218,
#27219),(#27220,#27221),(#27222,#27223),(#27224,#27225),(#27226,#27227),
(#27228,#27229),(#27230,#27231),(#27232,#27233),(#27234,#27235),(#27236,
#27237),(#27238,#27239),(#27240,#27241),(#27242,#27243),(#27244,#27245),
(#27246,#27247),(#27248,#27249),(#27250,#27251),(#27252,#27253),(#27254,
#27255),(#27256,#27257),(#27258,#27259),(#27260,#27261)),.UNSPECIFIED.,
 .F.,.F.,.F.)
B_SPLINE_SURFACE_WITH_KNOTS((6,1,1,1,1,1,1,1,1,1,1,1,1,1,1,1,1,1,1,1,1,
1,1,1,1,1,1,1,1,1,1,1,1,1,1,1,1,1,1,1,1,1,1,1,1,1,1,1,1,1,1,1,1,1,1,1,1,
1,1,1,1,1,1,1,1,6),(2,2),(-1.,-0.984615384615383,-0.969230769230768,-0.953846153846152,
-0.938461538461537,-0.923076923076922,-0.907692307692306,-0.892307692307691,
-0.876923076923076,-0.86153846153846,-0.846153846153845,-0.83076923076923,
-0.815384615384614,-0.799999999999999,-0.784615384615384,-0.769230769230768,
-0.753846153846153,-0.738461538461538,-0.723076923076922,-0.707692307692307,
-0.692307692307692,-0.676923076923076,-0.661538461538461,-0.646153846153846,
-0.63076923076923,-0.615384615384615,-0.6,-0.584615384615384,-0.569230769230769,
-0.553846153846154,-0.538461538461538,-0.523076923076923,-0.507692307692308,
-0.492307692307692,-0.476923076923077,-0.461538461538462,-0.446153846153846,
-0.430769230769231,-0.415384615384615,-0.4,-0.384615384615385,-0.369230769230769,
-0.353846153846154,-0.338461538461538,-0.323076923076923,-0.307692307692308,
-0.292307692307692,-0.276923076923077,-0.261538461538462,-0.246153846153846,
-0.230769230769231,-0.215384615384615,-0.2,-0.184615384615385,-0.169230769230769,
-0.153846153846154,-0.138461538461538,-0.123076923076923,-0.107692307692308,
-0.0923076923076923,-0.0769230769230769,-0.0615384615384615,-0.0461538461538462,
-0.0307692307692308,-0.0153846153846154,0.),(-1.,1.),.UNSPECIFIED.)
GEOMETRIC_REPRESENTATION_ITEM()
RATIONAL_B_SPLINE_SURFACE(((1.,1.),(1.,1.),(1.,1.),(1.,1.),(1.,1.),(1.,
1.),(1.,1.),(1.,1.),(1.,1.),(1.,1.),(1.,1.),(1.,1.),(1.,1.),(1.,1.),(1.,
1.),(1.,1.),(1.,1.),(1.,1.),(1.,1.),(1.,1.),(1.,1.),(1.,1.),(1.,1.),(1.,
1.),(1.,1.),(1.,1.),(1.,1.),(1.,1.),(1.,1.),(1.,1.),(1.,1.),(1.,1.),(1.,
1.),(1.,1.),(1.,1.),(1.,1.),(1.,1.),(1.,1.),(1.,1.),(1.,1.),(1.,1.),(1.,
1.),(1.,1.),(1.,1.),(1.,1.),(1.,1.),(1.,1.),(1.,1.),(1.,1.),(1.,1.),(1.,
1.),(1.,1.),(1.,1.),(1.,1.),(1.,1.),(1.,1.),(1.,1.),(1.,1.),(1.,1.),(1.,
1.),(1.,1.),(1.,1.),(1.,1.),(1.,1.),(1.,1.),(1.,1.),(1.,1.),(1.,1.),(1.,
1.),(1.,1.)))
REPRESENTATION_ITEM('')
SURFACE()
);
#21=(
BOUNDED_SURFACE()
B_SPLINE_SURFACE(5,1,((#27338,#27339),(#27340,#27341),(#27342,#27343),(#27344,
#27345),(#27346,#27347),(#27348,#27349),(#27350,#27351),(#27352,#27353),
(#27354,#27355),(#27356,#27357),(#27358,#27359),(#27360,#27361),(#27362,
#27363),(#27364,#27365),(#27366,#27367),(#27368,#27369),(#27370,#27371),
(#27372,#27373),(#27374,#27375),(#27376,#27377),(#27378,#27379),(#27380,
#27381),(#27382,#27383),(#27384,#27385),(#27386,#27387),(#27388,#27389),
(#27390,#27391),(#27392,#27393),(#27394,#27395),(#27396,#27397),(#27398,
#27399),(#27400,#27401),(#27402,#27403),(#27404,#27405),(#27406,#27407),
(#27408,#27409),(#27410,#27411),(#27412,#27413),(#27414,#27415),(#27416,
#27417),(#27418,#27419),(#27420,#27421),(#27422,#27423),(#27424,#27425),
(#27426,#27427),(#27428,#27429),(#27430,#27431),(#27432,#27433),(#27434,
#27435),(#27436,#27437),(#27438,#27439),(#27440,#27441),(#27442,#27443),
(#27444,#27445),(#27446,#27447),(#27448,#27449),(#27450,#27451),(#27452,
#27453),(#27454,#27455),(#27456,#27457),(#27458,#27459),(#27460,#27461),
(#27462,#27463),(#27464,#27465),(#27466,#27467),(#27468,#27469),(#27470,
#27471),(#27472,#27473),(#27474,#27475),(#27476,#27477)),.UNSPECIFIED.,
 .F.,.F.,.F.)
B_SPLINE_SURFACE_WITH_KNOTS((6,1,1,1,1,1,1,1,1,1,1,1,1,1,1,1,1,1,1,1,1,
1,1,1,1,1,1,1,1,1,1,1,1,1,1,1,1,1,1,1,1,1,1,1,1,1,1,1,1,1,1,1,1,1,1,1,1,
1,1,1,1,1,1,1,1,6),(2,2),(-1.,-0.984615384615383,-0.969230769230768,-0.953846153846152,
-0.938461538461537,-0.923076923076922,-0.907692307692306,-0.892307692307691,
-0.876923076923076,-0.86153846153846,-0.846153846153845,-0.83076923076923,
-0.815384615384614,-0.799999999999999,-0.784615384615384,-0.769230769230768,
-0.753846153846153,-0.738461538461538,-0.723076923076922,-0.707692307692307,
-0.692307692307692,-0.676923076923076,-0.661538461538461,-0.646153846153846,
-0.63076923076923,-0.615384615384615,-0.6,-0.584615384615384,-0.569230769230769,
-0.553846153846154,-0.538461538461538,-0.523076923076923,-0.507692307692308,
-0.492307692307692,-0.476923076923077,-0.461538461538462,-0.446153846153846,
-0.430769230769231,-0.415384615384615,-0.4,-0.384615384615385,-0.369230769230769,
-0.353846153846154,-0.338461538461538,-0.323076923076923,-0.307692307692308,
-0.292307692307692,-0.276923076923077,-0.261538461538462,-0.246153846153846,
-0.230769230769231,-0.215384615384615,-0.2,-0.184615384615385,-0.169230769230769,
-0.153846153846154,-0.138461538461538,-0.123076923076923,-0.107692307692308,
-0.0923076923076923,-0.0769230769230769,-0.0615384615384615,-0.0461538461538462,
-0.0307692307692308,-0.0153846153846154,0.),(-1.,1.),.UNSPECIFIED.)
GEOMETRIC_REPRESENTATION_ITEM()
RATIONAL_B_SPLINE_SURFACE(((1.,1.),(1.,1.),(1.,1.),(1.,1.),(1.,1.),(1.,
1.),(1.,1.),(1.,1.),(1.,1.),(1.,1.),(1.,1.),(1.,1.),(1.,1.),(1.,1.),(1.,
1.),(1.,1.),(1.,1.),(1.,1.),(1.,1.),(1.,1.),(1.,1.),(1.,1.),(1.,1.),(1.,
1.),(1.,1.),(1.,1.),(1.,1.),(1.,1.),(1.,1.),(1.,1.),(1.,1.),(1.,1.),(1.,
1.),(1.,1.),(1.,1.),(1.,1.),(1.,1.),(1.,1.),(1.,1.),(1.,1.),(1.,1.),(1.,
1.),(1.,1.),(1.,1.),(1.,1.),(1.,1.),(1.,1.),(1.,1.),(1.,1.),(1.,1.),(1.,
1.),(1.,1.),(1.,1.),(1.,1.),(1.,1.),(1.,1.),(1.,1.),(1.,1.),(1.,1.),(1.,
1.),(1.,1.),(1.,1.),(1.,1.),(1.,1.),(1.,1.),(1.,1.),(1.,1.),(1.,1.),(1.,
1.),(1.,1.)))
REPRESENTATION_ITEM('')
SURFACE()
);
#22=(
BOUNDED_SURFACE()
B_SPLINE_SURFACE(5,1,((#27554,#27555),(#27556,#27557),(#27558,#27559),(#27560,
#27561),(#27562,#27563),(#27564,#27565),(#27566,#27567),(#27568,#27569),
(#27570,#27571),(#27572,#27573),(#27574,#27575),(#27576,#27577),(#27578,
#27579),(#27580,#27581),(#27582,#27583),(#27584,#27585),(#27586,#27587),
(#27588,#27589),(#27590,#27591),(#27592,#27593),(#27594,#27595),(#27596,
#27597),(#27598,#27599),(#27600,#27601),(#27602,#27603),(#27604,#27605),
(#27606,#27607),(#27608,#27609),(#27610,#27611),(#27612,#27613),(#27614,
#27615),(#27616,#27617),(#27618,#27619),(#27620,#27621),(#27622,#27623),
(#27624,#27625),(#27626,#27627),(#27628,#27629),(#27630,#27631),(#27632,
#27633),(#27634,#27635),(#27636,#27637),(#27638,#27639),(#27640,#27641),
(#27642,#27643),(#27644,#27645),(#27646,#27647),(#27648,#27649),(#27650,
#27651),(#27652,#27653),(#27654,#27655),(#27656,#27657),(#27658,#27659),
(#27660,#27661),(#27662,#27663),(#27664,#27665),(#27666,#27667),(#27668,
#27669),(#27670,#27671),(#27672,#27673),(#27674,#27675),(#27676,#27677),
(#27678,#27679),(#27680,#27681),(#27682,#27683),(#27684,#27685),(#27686,
#27687),(#27688,#27689),(#27690,#27691),(#27692,#27693)),.UNSPECIFIED.,
 .F.,.F.,.F.)
B_SPLINE_SURFACE_WITH_KNOTS((6,1,1,1,1,1,1,1,1,1,1,1,1,1,1,1,1,1,1,1,1,
1,1,1,1,1,1,1,1,1,1,1,1,1,1,1,1,1,1,1,1,1,1,1,1,1,1,1,1,1,1,1,1,1,1,1,1,
1,1,1,1,1,1,1,1,6),(2,2),(-1.,-0.984615384615383,-0.969230769230768,-0.953846153846152,
-0.938461538461537,-0.923076923076922,-0.907692307692306,-0.892307692307691,
-0.876923076923076,-0.86153846153846,-0.846153846153845,-0.83076923076923,
-0.815384615384614,-0.799999999999999,-0.784615384615384,-0.769230769230768,
-0.753846153846153,-0.738461538461538,-0.723076923076922,-0.707692307692307,
-0.692307692307692,-0.676923076923076,-0.661538461538461,-0.646153846153846,
-0.63076923076923,-0.615384615384615,-0.6,-0.584615384615384,-0.569230769230769,
-0.553846153846154,-0.538461538461538,-0.523076923076923,-0.507692307692308,
-0.492307692307692,-0.476923076923077,-0.461538461538462,-0.446153846153846,
-0.430769230769231,-0.415384615384615,-0.4,-0.384615384615385,-0.369230769230769,
-0.353846153846154,-0.338461538461538,-0.323076923076923,-0.307692307692308,
-0.292307692307692,-0.276923076923077,-0.261538461538462,-0.246153846153846,
-0.230769230769231,-0.215384615384615,-0.2,-0.184615384615385,-0.169230769230769,
-0.153846153846154,-0.138461538461538,-0.123076923076923,-0.107692307692308,
-0.0923076923076923,-0.0769230769230769,-0.0615384615384615,-0.0461538461538462,
-0.0307692307692308,-0.0153846153846154,0.),(-1.,1.),.UNSPECIFIED.)
GEOMETRIC_REPRESENTATION_ITEM()
RATIONAL_B_SPLINE_SURFACE(((1.,1.),(1.,1.),(1.,1.),(1.,1.),(1.,1.),(1.,
1.),(1.,1.),(1.,1.),(1.,1.),(1.,1.),(1.,1.),(1.,1.),(1.,1.),(1.,1.),(1.,
1.),(1.,1.),(1.,1.),(1.,1.),(1.,1.),(1.,1.),(1.,1.),(1.,1.),(1.,1.),(1.,
1.),(1.,1.),(1.,1.),(1.,1.),(1.,1.),(1.,1.),(1.,1.),(1.,1.),(1.,1.),(1.,
1.),(1.,1.),(1.,1.),(1.,1.),(1.,1.),(1.,1.),(1.,1.),(1.,1.),(1.,1.),(1.,
1.),(1.,1.),(1.,1.),(1.,1.),(1.,1.),(1.,1.),(1.,1.),(1.,1.),(1.,1.),(1.,
1.),(1.,1.),(1.,1.),(1.,1.),(1.,1.),(1.,1.),(1.,1.),(1.,1.),(1.,1.),(1.,
1.),(1.,1.),(1.,1.),(1.,1.),(1.,1.),(1.,1.),(1.,1.),(1.,1.),(1.,1.),(1.,
1.),(1.,1.)))
REPRESENTATION_ITEM('')
SURFACE()
);
#23=(
BOUNDED_SURFACE()
B_SPLINE_SURFACE(5,1,((#27770,#27771),(#27772,#27773),(#27774,#27775),(#27776,
#27777),(#27778,#27779),(#27780,#27781),(#27782,#27783),(#27784,#27785),
(#27786,#27787),(#27788,#27789),(#27790,#27791),(#27792,#27793),(#27794,
#27795),(#27796,#27797),(#27798,#27799),(#27800,#27801),(#27802,#27803),
(#27804,#27805),(#27806,#27807),(#27808,#27809),(#27810,#27811),(#27812,
#27813),(#27814,#27815),(#27816,#27817),(#27818,#27819),(#27820,#27821),
(#27822,#27823),(#27824,#27825),(#27826,#27827),(#27828,#27829),(#27830,
#27831),(#27832,#27833),(#27834,#27835),(#27836,#27837),(#27838,#27839),
(#27840,#27841),(#27842,#27843),(#27844,#27845),(#27846,#27847),(#27848,
#27849),(#27850,#27851),(#27852,#27853),(#27854,#27855),(#27856,#27857),
(#27858,#27859),(#27860,#27861),(#27862,#27863),(#27864,#27865),(#27866,
#27867),(#27868,#27869),(#27870,#27871),(#27872,#27873),(#27874,#27875),
(#27876,#27877),(#27878,#27879),(#27880,#27881),(#27882,#27883),(#27884,
#27885),(#27886,#27887),(#27888,#27889),(#27890,#27891),(#27892,#27893),
(#27894,#27895),(#27896,#27897),(#27898,#27899),(#27900,#27901),(#27902,
#27903),(#27904,#27905),(#27906,#27907),(#27908,#27909)),.UNSPECIFIED.,
 .F.,.F.,.F.)
B_SPLINE_SURFACE_WITH_KNOTS((6,1,1,1,1,1,1,1,1,1,1,1,1,1,1,1,1,1,1,1,1,
1,1,1,1,1,1,1,1,1,1,1,1,1,1,1,1,1,1,1,1,1,1,1,1,1,1,1,1,1,1,1,1,1,1,1,1,
1,1,1,1,1,1,1,1,6),(2,2),(-1.,-0.984615384615383,-0.969230769230768,-0.953846153846152,
-0.938461538461537,-0.923076923076922,-0.907692307692306,-0.892307692307691,
-0.876923076923076,-0.86153846153846,-0.846153846153845,-0.83076923076923,
-0.815384615384614,-0.799999999999999,-0.784615384615384,-0.769230769230768,
-0.753846153846153,-0.738461538461538,-0.723076923076922,-0.707692307692307,
-0.692307692307692,-0.676923076923076,-0.661538461538461,-0.646153846153846,
-0.63076923076923,-0.615384615384615,-0.6,-0.584615384615384,-0.569230769230769,
-0.553846153846154,-0.538461538461538,-0.523076923076923,-0.507692307692308,
-0.492307692307692,-0.476923076923077,-0.461538461538462,-0.446153846153846,
-0.430769230769231,-0.415384615384615,-0.4,-0.384615384615385,-0.369230769230769,
-0.353846153846154,-0.338461538461538,-0.323076923076923,-0.307692307692308,
-0.292307692307692,-0.276923076923077,-0.261538461538462,-0.246153846153846,
-0.230769230769231,-0.215384615384615,-0.2,-0.184615384615385,-0.169230769230769,
-0.153846153846154,-0.138461538461538,-0.123076923076923,-0.107692307692308,
-0.0923076923076923,-0.0769230769230769,-0.0615384615384615,-0.0461538461538462,
-0.0307692307692308,-0.0153846153846154,0.),(-1.,1.),.UNSPECIFIED.)
GEOMETRIC_REPRESENTATION_ITEM()
RATIONAL_B_SPLINE_SURFACE(((1.,1.),(1.,1.),(1.,1.),(1.,1.),(1.,1.),(1.,
1.),(1.,1.),(1.,1.),(1.,1.),(1.,1.),(1.,1.),(1.,1.),(1.,1.),(1.,1.),(1.,
1.),(1.,1.),(1.,1.),(1.,1.),(1.,1.),(1.,1.),(1.,1.),(1.,1.),(1.,1.),(1.,
1.),(1.,1.),(1.,1.),(1.,1.),(1.,1.),(1.,1.),(1.,1.),(1.,1.),(1.,1.),(1.,
1.),(1.,1.),(1.,1.),(1.,1.),(1.,1.),(1.,1.),(1.,1.),(1.,1.),(1.,1.),(1.,
1.),(1.,1.),(1.,1.),(1.,1.),(1.,1.),(1.,1.),(1.,1.),(1.,1.),(1.,1.),(1.,
1.),(1.,1.),(1.,1.),(1.,1.),(1.,1.),(1.,1.),(1.,1.),(1.,1.),(1.,1.),(1.,
1.),(1.,1.),(1.,1.),(1.,1.),(1.,1.),(1.,1.),(1.,1.),(1.,1.),(1.,1.),(1.,
1.),(1.,1.)))
REPRESENTATION_ITEM('')
SURFACE()
);
#24=(
BOUNDED_SURFACE()
B_SPLINE_SURFACE(5,1,((#27986,#27987),(#27988,#27989),(#27990,#27991),(#27992,
#27993),(#27994,#27995),(#27996,#27997),(#27998,#27999),(#28000,#28001),
(#28002,#28003),(#28004,#28005),(#28006,#28007),(#28008,#28009),(#28010,
#28011),(#28012,#28013),(#28014,#28015),(#28016,#28017),(#28018,#28019),
(#28020,#28021),(#28022,#28023),(#28024,#28025),(#28026,#28027),(#28028,
#28029),(#28030,#28031),(#28032,#28033),(#28034,#28035),(#28036,#28037),
(#28038,#28039),(#28040,#28041),(#28042,#28043),(#28044,#28045),(#28046,
#28047),(#28048,#28049),(#28050,#28051),(#28052,#28053),(#28054,#28055),
(#28056,#28057),(#28058,#28059),(#28060,#28061),(#28062,#28063),(#28064,
#28065),(#28066,#28067),(#28068,#28069),(#28070,#28071),(#28072,#28073),
(#28074,#28075),(#28076,#28077),(#28078,#28079),(#28080,#28081),(#28082,
#28083),(#28084,#28085),(#28086,#28087),(#28088,#28089),(#28090,#28091),
(#28092,#28093),(#28094,#28095),(#28096,#28097),(#28098,#28099),(#28100,
#28101),(#28102,#28103),(#28104,#28105),(#28106,#28107),(#28108,#28109),
(#28110,#28111),(#28112,#28113),(#28114,#28115),(#28116,#28117),(#28118,
#28119),(#28120,#28121),(#28122,#28123),(#28124,#28125)),.UNSPECIFIED.,
 .F.,.F.,.F.)
B_SPLINE_SURFACE_WITH_KNOTS((6,1,1,1,1,1,1,1,1,1,1,1,1,1,1,1,1,1,1,1,1,
1,1,1,1,1,1,1,1,1,1,1,1,1,1,1,1,1,1,1,1,1,1,1,1,1,1,1,1,1,1,1,1,1,1,1,1,
1,1,1,1,1,1,1,1,6),(2,2),(-1.,-0.984615384615383,-0.969230769230768,-0.953846153846152,
-0.938461538461537,-0.923076923076922,-0.907692307692306,-0.892307692307691,
-0.876923076923076,-0.86153846153846,-0.846153846153845,-0.83076923076923,
-0.815384615384614,-0.799999999999999,-0.784615384615384,-0.769230769230768,
-0.753846153846153,-0.738461538461538,-0.723076923076922,-0.707692307692307,
-0.692307692307692,-0.676923076923076,-0.661538461538461,-0.646153846153846,
-0.63076923076923,-0.615384615384615,-0.6,-0.584615384615384,-0.569230769230769,
-0.553846153846154,-0.538461538461538,-0.523076923076923,-0.507692307692308,
-0.492307692307692,-0.476923076923077,-0.461538461538462,-0.446153846153846,
-0.430769230769231,-0.415384615384615,-0.4,-0.384615384615385,-0.369230769230769,
-0.353846153846154,-0.338461538461538,-0.323076923076923,-0.307692307692308,
-0.292307692307692,-0.276923076923077,-0.261538461538462,-0.246153846153846,
-0.230769230769231,-0.215384615384615,-0.2,-0.184615384615385,-0.169230769230769,
-0.153846153846154,-0.138461538461538,-0.123076923076923,-0.107692307692308,
-0.0923076923076923,-0.0769230769230769,-0.0615384615384615,-0.0461538461538462,
-0.0307692307692308,-0.0153846153846154,0.),(-1.,1.),.UNSPECIFIED.)
GEOMETRIC_REPRESENTATION_ITEM()
RATIONAL_B_SPLINE_SURFACE(((1.,1.),(1.,1.),(1.,1.),(1.,1.),(1.,1.),(1.,
1.),(1.,1.),(1.,1.),(1.,1.),(1.,1.),(1.,1.),(1.,1.),(1.,1.),(1.,1.),(1.,
1.),(1.,1.),(1.,1.),(1.,1.),(1.,1.),(1.,1.),(1.,1.),(1.,1.),(1.,1.),(1.,
1.),(1.,1.),(1.,1.),(1.,1.),(1.,1.),(1.,1.),(1.,1.),(1.,1.),(1.,1.),(1.,
1.),(1.,1.),(1.,1.),(1.,1.),(1.,1.),(1.,1.),(1.,1.),(1.,1.),(1.,1.),(1.,
1.),(1.,1.),(1.,1.),(1.,1.),(1.,1.),(1.,1.),(1.,1.),(1.,1.),(1.,1.),(1.,
1.),(1.,1.),(1.,1.),(1.,1.),(1.,1.),(1.,1.),(1.,1.),(1.,1.),(1.,1.),(1.,
1.),(1.,1.),(1.,1.),(1.,1.),(1.,1.),(1.,1.),(1.,1.),(1.,1.),(1.,1.),(1.,
1.),(1.,1.)))
REPRESENTATION_ITEM('')
SURFACE()
);
#25=(
BOUNDED_SURFACE()
B_SPLINE_SURFACE(5,1,((#28202,#28203),(#28204,#28205),(#28206,#28207),(#28208,
#28209),(#28210,#28211),(#28212,#28213),(#28214,#28215),(#28216,#28217),
(#28218,#28219),(#28220,#28221),(#28222,#28223),(#28224,#28225),(#28226,
#28227),(#28228,#28229),(#28230,#28231),(#28232,#28233),(#28234,#28235),
(#28236,#28237),(#28238,#28239),(#28240,#28241),(#28242,#28243),(#28244,
#28245),(#28246,#28247),(#28248,#28249),(#28250,#28251),(#28252,#28253),
(#28254,#28255),(#28256,#28257),(#28258,#28259),(#28260,#28261),(#28262,
#28263),(#28264,#28265),(#28266,#28267),(#28268,#28269),(#28270,#28271),
(#28272,#28273),(#28274,#28275),(#28276,#28277),(#28278,#28279),(#28280,
#28281),(#28282,#28283),(#28284,#28285),(#28286,#28287),(#28288,#28289),
(#28290,#28291),(#28292,#28293),(#28294,#28295),(#28296,#28297),(#28298,
#28299),(#28300,#28301),(#28302,#28303),(#28304,#28305),(#28306,#28307),
(#28308,#28309),(#28310,#28311),(#28312,#28313),(#28314,#28315),(#28316,
#28317),(#28318,#28319),(#28320,#28321),(#28322,#28323),(#28324,#28325),
(#28326,#28327),(#28328,#28329),(#28330,#28331),(#28332,#28333),(#28334,
#28335),(#28336,#28337),(#28338,#28339),(#28340,#28341)),.UNSPECIFIED.,
 .F.,.F.,.F.)
B_SPLINE_SURFACE_WITH_KNOTS((6,1,1,1,1,1,1,1,1,1,1,1,1,1,1,1,1,1,1,1,1,
1,1,1,1,1,1,1,1,1,1,1,1,1,1,1,1,1,1,1,1,1,1,1,1,1,1,1,1,1,1,1,1,1,1,1,1,
1,1,1,1,1,1,1,1,6),(2,2),(-1.,-0.984615384615383,-0.969230769230768,-0.953846153846152,
-0.938461538461537,-0.923076923076922,-0.907692307692306,-0.892307692307691,
-0.876923076923076,-0.86153846153846,-0.846153846153845,-0.83076923076923,
-0.815384615384614,-0.799999999999999,-0.784615384615384,-0.769230769230768,
-0.753846153846153,-0.738461538461538,-0.723076923076922,-0.707692307692307,
-0.692307692307692,-0.676923076923076,-0.661538461538461,-0.646153846153846,
-0.63076923076923,-0.615384615384615,-0.6,-0.584615384615384,-0.569230769230769,
-0.553846153846154,-0.538461538461538,-0.523076923076923,-0.507692307692308,
-0.492307692307692,-0.476923076923077,-0.461538461538462,-0.446153846153846,
-0.430769230769231,-0.415384615384615,-0.4,-0.384615384615385,-0.369230769230769,
-0.353846153846154,-0.338461538461538,-0.323076923076923,-0.307692307692308,
-0.292307692307692,-0.276923076923077,-0.261538461538462,-0.246153846153846,
-0.230769230769231,-0.215384615384615,-0.2,-0.184615384615385,-0.169230769230769,
-0.153846153846154,-0.138461538461538,-0.123076923076923,-0.107692307692308,
-0.0923076923076923,-0.0769230769230769,-0.0615384615384615,-0.0461538461538462,
-0.0307692307692308,-0.0153846153846154,0.),(-1.,1.),.UNSPECIFIED.)
GEOMETRIC_REPRESENTATION_ITEM()
RATIONAL_B_SPLINE_SURFACE(((1.,1.),(1.,1.),(1.,1.),(1.,1.),(1.,1.),(1.,
1.),(1.,1.),(1.,1.),(1.,1.),(1.,1.),(1.,1.),(1.,1.),(1.,1.),(1.,1.),(1.,
1.),(1.,1.),(1.,1.),(1.,1.),(1.,1.),(1.,1.),(1.,1.),(1.,1.),(1.,1.),(1.,
1.),(1.,1.),(1.,1.),(1.,1.),(1.,1.),(1.,1.),(1.,1.),(1.,1.),(1.,1.),(1.,
1.),(1.,1.),(1.,1.),(1.,1.),(1.,1.),(1.,1.),(1.,1.),(1.,1.),(1.,1.),(1.,
1.),(1.,1.),(1.,1.),(1.,1.),(1.,1.),(1.,1.),(1.,1.),(1.,1.),(1.,1.),(1.,
1.),(1.,1.),(1.,1.),(1.,1.),(1.,1.),(1.,1.),(1.,1.),(1.,1.),(1.,1.),(1.,
1.),(1.,1.),(1.,1.),(1.,1.),(1.,1.),(1.,1.),(1.,1.),(1.,1.),(1.,1.),(1.,
1.),(1.,1.)))
REPRESENTATION_ITEM('')
SURFACE()
);
#26=(
BOUNDED_SURFACE()
B_SPLINE_SURFACE(5,1,((#28418,#28419),(#28420,#28421),(#28422,#28423),(#28424,
#28425),(#28426,#28427),(#28428,#28429),(#28430,#28431),(#28432,#28433),
(#28434,#28435),(#28436,#28437),(#28438,#28439),(#28440,#28441),(#28442,
#28443),(#28444,#28445),(#28446,#28447),(#28448,#28449),(#28450,#28451),
(#28452,#28453),(#28454,#28455),(#28456,#28457),(#28458,#28459),(#28460,
#28461),(#28462,#28463),(#28464,#28465),(#28466,#28467),(#28468,#28469),
(#28470,#28471),(#28472,#28473),(#28474,#28475),(#28476,#28477),(#28478,
#28479),(#28480,#28481),(#28482,#28483),(#28484,#28485),(#28486,#28487),
(#28488,#28489),(#28490,#28491),(#28492,#28493),(#28494,#28495),(#28496,
#28497),(#28498,#28499),(#28500,#28501),(#28502,#28503),(#28504,#28505),
(#28506,#28507),(#28508,#28509),(#28510,#28511),(#28512,#28513),(#28514,
#28515),(#28516,#28517),(#28518,#28519),(#28520,#28521),(#28522,#28523),
(#28524,#28525),(#28526,#28527),(#28528,#28529),(#28530,#28531),(#28532,
#28533),(#28534,#28535),(#28536,#28537),(#28538,#28539),(#28540,#28541),
(#28542,#28543),(#28544,#28545),(#28546,#28547),(#28548,#28549),(#28550,
#28551),(#28552,#28553),(#28554,#28555),(#28556,#28557)),.UNSPECIFIED.,
 .F.,.F.,.F.)
B_SPLINE_SURFACE_WITH_KNOTS((6,1,1,1,1,1,1,1,1,1,1,1,1,1,1,1,1,1,1,1,1,
1,1,1,1,1,1,1,1,1,1,1,1,1,1,1,1,1,1,1,1,1,1,1,1,1,1,1,1,1,1,1,1,1,1,1,1,
1,1,1,1,1,1,1,1,6),(2,2),(-1.,-0.984615384615383,-0.969230769230768,-0.953846153846152,
-0.938461538461537,-0.923076923076922,-0.907692307692306,-0.892307692307691,
-0.876923076923076,-0.86153846153846,-0.846153846153845,-0.83076923076923,
-0.815384615384614,-0.799999999999999,-0.784615384615384,-0.769230769230768,
-0.753846153846153,-0.738461538461538,-0.723076923076922,-0.707692307692307,
-0.692307692307692,-0.676923076923076,-0.661538461538461,-0.646153846153846,
-0.63076923076923,-0.615384615384615,-0.6,-0.584615384615384,-0.569230769230769,
-0.553846153846154,-0.538461538461538,-0.523076923076923,-0.507692307692308,
-0.492307692307692,-0.476923076923077,-0.461538461538462,-0.446153846153846,
-0.430769230769231,-0.415384615384615,-0.4,-0.384615384615385,-0.369230769230769,
-0.353846153846154,-0.338461538461538,-0.323076923076923,-0.307692307692308,
-0.292307692307692,-0.276923076923077,-0.261538461538462,-0.246153846153846,
-0.230769230769231,-0.215384615384615,-0.2,-0.184615384615385,-0.169230769230769,
-0.153846153846154,-0.138461538461538,-0.123076923076923,-0.107692307692308,
-0.0923076923076923,-0.0769230769230769,-0.0615384615384615,-0.0461538461538462,
-0.0307692307692308,-0.0153846153846154,0.),(-1.,1.),.UNSPECIFIED.)
GEOMETRIC_REPRESENTATION_ITEM()
RATIONAL_B_SPLINE_SURFACE(((1.,1.),(1.,1.),(1.,1.),(1.,1.),(1.,1.),(1.,
1.),(1.,1.),(1.,1.),(1.,1.),(1.,1.),(1.,1.),(1.,1.),(1.,1.),(1.,1.),(1.,
1.),(1.,1.),(1.,1.),(1.,1.),(1.,1.),(1.,1.),(1.,1.),(1.,1.),(1.,1.),(1.,
1.),(1.,1.),(1.,1.),(1.,1.),(1.,1.),(1.,1.),(1.,1.),(1.,1.),(1.,1.),(1.,
1.),(1.,1.),(1.,1.),(1.,1.),(1.,1.),(1.,1.),(1.,1.),(1.,1.),(1.,1.),(1.,
1.),(1.,1.),(1.,1.),(1.,1.),(1.,1.),(1.,1.),(1.,1.),(1.,1.),(1.,1.),(1.,
1.),(1.,1.),(1.,1.),(1.,1.),(1.,1.),(1.,1.),(1.,1.),(1.,1.),(1.,1.),(1.,
1.),(1.,1.),(1.,1.),(1.,1.),(1.,1.),(1.,1.),(1.,1.),(1.,1.),(1.,1.),(1.,
1.),(1.,1.)))
REPRESENTATION_ITEM('')
SURFACE()
);
#27=(
BOUNDED_SURFACE()
B_SPLINE_SURFACE(5,1,((#28634,#28635),(#28636,#28637),(#28638,#28639),(#28640,
#28641),(#28642,#28643),(#28644,#28645),(#28646,#28647),(#28648,#28649),
(#28650,#28651),(#28652,#28653),(#28654,#28655),(#28656,#28657),(#28658,
#28659),(#28660,#28661),(#28662,#28663),(#28664,#28665),(#28666,#28667),
(#28668,#28669),(#28670,#28671),(#28672,#28673),(#28674,#28675),(#28676,
#28677),(#28678,#28679),(#28680,#28681),(#28682,#28683),(#28684,#28685),
(#28686,#28687),(#28688,#28689),(#28690,#28691),(#28692,#28693),(#28694,
#28695),(#28696,#28697),(#28698,#28699),(#28700,#28701),(#28702,#28703),
(#28704,#28705),(#28706,#28707),(#28708,#28709),(#28710,#28711),(#28712,
#28713),(#28714,#28715),(#28716,#28717),(#28718,#28719),(#28720,#28721),
(#28722,#28723),(#28724,#28725),(#28726,#28727),(#28728,#28729),(#28730,
#28731),(#28732,#28733),(#28734,#28735),(#28736,#28737),(#28738,#28739),
(#28740,#28741),(#28742,#28743),(#28744,#28745),(#28746,#28747),(#28748,
#28749),(#28750,#28751),(#28752,#28753),(#28754,#28755),(#28756,#28757),
(#28758,#28759),(#28760,#28761),(#28762,#28763),(#28764,#28765),(#28766,
#28767),(#28768,#28769),(#28770,#28771),(#28772,#28773)),.UNSPECIFIED.,
 .F.,.F.,.F.)
B_SPLINE_SURFACE_WITH_KNOTS((6,1,1,1,1,1,1,1,1,1,1,1,1,1,1,1,1,1,1,1,1,
1,1,1,1,1,1,1,1,1,1,1,1,1,1,1,1,1,1,1,1,1,1,1,1,1,1,1,1,1,1,1,1,1,1,1,1,
1,1,1,1,1,1,1,1,6),(2,2),(-1.,-0.984615384615383,-0.969230769230768,-0.953846153846152,
-0.938461538461537,-0.923076923076922,-0.907692307692306,-0.892307692307691,
-0.876923076923076,-0.86153846153846,-0.846153846153845,-0.83076923076923,
-0.815384615384614,-0.799999999999999,-0.784615384615384,-0.769230769230768,
-0.753846153846153,-0.738461538461538,-0.723076923076922,-0.707692307692307,
-0.692307692307692,-0.676923076923076,-0.661538461538461,-0.646153846153846,
-0.63076923076923,-0.615384615384615,-0.6,-0.584615384615384,-0.569230769230769,
-0.553846153846154,-0.538461538461538,-0.523076923076923,-0.507692307692308,
-0.492307692307692,-0.476923076923077,-0.461538461538462,-0.446153846153846,
-0.430769230769231,-0.415384615384615,-0.4,-0.384615384615385,-0.369230769230769,
-0.353846153846154,-0.338461538461538,-0.323076923076923,-0.307692307692308,
-0.292307692307692,-0.276923076923077,-0.261538461538462,-0.246153846153846,
-0.230769230769231,-0.215384615384615,-0.2,-0.184615384615385,-0.169230769230769,
-0.153846153846154,-0.138461538461538,-0.123076923076923,-0.107692307692308,
-0.0923076923076923,-0.0769230769230769,-0.0615384615384615,-0.0461538461538462,
-0.0307692307692308,-0.0153846153846154,0.),(-1.,1.),.UNSPECIFIED.)
GEOMETRIC_REPRESENTATION_ITEM()
RATIONAL_B_SPLINE_SURFACE(((1.,1.),(1.,1.),(1.,1.),(1.,1.),(1.,1.),(1.,
1.),(1.,1.),(1.,1.),(1.,1.),(1.,1.),(1.,1.),(1.,1.),(1.,1.),(1.,1.),(1.,
1.),(1.,1.),(1.,1.),(1.,1.),(1.,1.),(1.,1.),(1.,1.),(1.,1.),(1.,1.),(1.,
1.),(1.,1.),(1.,1.),(1.,1.),(1.,1.),(1.,1.),(1.,1.),(1.,1.),(1.,1.),(1.,
1.),(1.,1.),(1.,1.),(1.,1.),(1.,1.),(1.,1.),(1.,1.),(1.,1.),(1.,1.),(1.,
1.),(1.,1.),(1.,1.),(1.,1.),(1.,1.),(1.,1.),(1.,1.),(1.,1.),(1.,1.),(1.,
1.),(1.,1.),(1.,1.),(1.,1.),(1.,1.),(1.,1.),(1.,1.),(1.,1.),(1.,1.),(1.,
1.),(1.,1.),(1.,1.),(1.,1.),(1.,1.),(1.,1.),(1.,1.),(1.,1.),(1.,1.),(1.,
1.),(1.,1.)))
REPRESENTATION_ITEM('')
SURFACE()
);
#28=(
BOUNDED_SURFACE()
B_SPLINE_SURFACE(5,1,((#28850,#28851),(#28852,#28853),(#28854,#28855),(#28856,
#28857),(#28858,#28859),(#28860,#28861),(#28862,#28863),(#28864,#28865),
(#28866,#28867),(#28868,#28869),(#28870,#28871),(#28872,#28873),(#28874,
#28875),(#28876,#28877),(#28878,#28879),(#28880,#28881),(#28882,#28883),
(#28884,#28885),(#28886,#28887),(#28888,#28889),(#28890,#28891),(#28892,
#28893),(#28894,#28895),(#28896,#28897),(#28898,#28899),(#28900,#28901),
(#28902,#28903),(#28904,#28905),(#28906,#28907),(#28908,#28909),(#28910,
#28911),(#28912,#28913),(#28914,#28915),(#28916,#28917),(#28918,#28919),
(#28920,#28921),(#28922,#28923),(#28924,#28925),(#28926,#28927),(#28928,
#28929),(#28930,#28931),(#28932,#28933),(#28934,#28935),(#28936,#28937),
(#28938,#28939),(#28940,#28941),(#28942,#28943),(#28944,#28945),(#28946,
#28947),(#28948,#28949),(#28950,#28951),(#28952,#28953),(#28954,#28955),
(#28956,#28957),(#28958,#28959),(#28960,#28961),(#28962,#28963),(#28964,
#28965),(#28966,#28967),(#28968,#28969),(#28970,#28971),(#28972,#28973),
(#28974,#28975),(#28976,#28977),(#28978,#28979),(#28980,#28981),(#28982,
#28983),(#28984,#28985),(#28986,#28987),(#28988,#28989)),.UNSPECIFIED.,
 .F.,.F.,.F.)
B_SPLINE_SURFACE_WITH_KNOTS((6,1,1,1,1,1,1,1,1,1,1,1,1,1,1,1,1,1,1,1,1,
1,1,1,1,1,1,1,1,1,1,1,1,1,1,1,1,1,1,1,1,1,1,1,1,1,1,1,1,1,1,1,1,1,1,1,1,
1,1,1,1,1,1,1,1,6),(2,2),(-1.,-0.984615384615383,-0.969230769230768,-0.953846153846152,
-0.938461538461537,-0.923076923076922,-0.907692307692306,-0.892307692307691,
-0.876923076923076,-0.86153846153846,-0.846153846153845,-0.83076923076923,
-0.815384615384614,-0.799999999999999,-0.784615384615384,-0.769230769230768,
-0.753846153846153,-0.738461538461538,-0.723076923076922,-0.707692307692307,
-0.692307692307692,-0.676923076923076,-0.661538461538461,-0.646153846153846,
-0.63076923076923,-0.615384615384615,-0.6,-0.584615384615384,-0.569230769230769,
-0.553846153846154,-0.538461538461538,-0.523076923076923,-0.507692307692308,
-0.492307692307692,-0.476923076923077,-0.461538461538462,-0.446153846153846,
-0.430769230769231,-0.415384615384615,-0.4,-0.384615384615385,-0.369230769230769,
-0.353846153846154,-0.338461538461538,-0.323076923076923,-0.307692307692308,
-0.292307692307692,-0.276923076923077,-0.261538461538462,-0.246153846153846,
-0.230769230769231,-0.215384615384615,-0.2,-0.184615384615385,-0.169230769230769,
-0.153846153846154,-0.138461538461538,-0.123076923076923,-0.107692307692308,
-0.0923076923076923,-0.0769230769230769,-0.0615384615384615,-0.0461538461538462,
-0.0307692307692308,-0.0153846153846154,0.),(-1.,1.),.UNSPECIFIED.)
GEOMETRIC_REPRESENTATION_ITEM()
RATIONAL_B_SPLINE_SURFACE(((1.,1.),(1.,1.),(1.,1.),(1.,1.),(1.,1.),(1.,
1.),(1.,1.),(1.,1.),(1.,1.),(1.,1.),(1.,1.),(1.,1.),(1.,1.),(1.,1.),(1.,
1.),(1.,1.),(1.,1.),(1.,1.),(1.,1.),(1.,1.),(1.,1.),(1.,1.),(1.,1.),(1.,
1.),(1.,1.),(1.,1.),(1.,1.),(1.,1.),(1.,1.),(1.,1.),(1.,1.),(1.,1.),(1.,
1.),(1.,1.),(1.,1.),(1.,1.),(1.,1.),(1.,1.),(1.,1.),(1.,1.),(1.,1.),(1.,
1.),(1.,1.),(1.,1.),(1.,1.),(1.,1.),(1.,1.),(1.,1.),(1.,1.),(1.,1.),(1.,
1.),(1.,1.),(1.,1.),(1.,1.),(1.,1.),(1.,1.),(1.,1.),(1.,1.),(1.,1.),(1.,
1.),(1.,1.),(1.,1.),(1.,1.),(1.,1.),(1.,1.),(1.,1.),(1.,1.),(1.,1.),(1.,
1.),(1.,1.)))
REPRESENTATION_ITEM('')
SURFACE()
);
#29=(
BOUNDED_SURFACE()
B_SPLINE_SURFACE(5,1,((#29066,#29067),(#29068,#29069),(#29070,#29071),(#29072,
#29073),(#29074,#29075),(#29076,#29077),(#29078,#29079),(#29080,#29081),
(#29082,#29083),(#29084,#29085),(#29086,#29087),(#29088,#29089),(#29090,
#29091),(#29092,#29093),(#29094,#29095),(#29096,#29097),(#29098,#29099),
(#29100,#29101),(#29102,#29103),(#29104,#29105),(#29106,#29107),(#29108,
#29109),(#29110,#29111),(#29112,#29113),(#29114,#29115),(#29116,#29117),
(#29118,#29119),(#29120,#29121),(#29122,#29123),(#29124,#29125),(#29126,
#29127),(#29128,#29129),(#29130,#29131),(#29132,#29133),(#29134,#29135),
(#29136,#29137),(#29138,#29139),(#29140,#29141),(#29142,#29143),(#29144,
#29145),(#29146,#29147),(#29148,#29149),(#29150,#29151),(#29152,#29153),
(#29154,#29155),(#29156,#29157),(#29158,#29159),(#29160,#29161),(#29162,
#29163),(#29164,#29165),(#29166,#29167),(#29168,#29169),(#29170,#29171),
(#29172,#29173),(#29174,#29175),(#29176,#29177),(#29178,#29179),(#29180,
#29181),(#29182,#29183),(#29184,#29185),(#29186,#29187),(#29188,#29189),
(#29190,#29191),(#29192,#29193),(#29194,#29195),(#29196,#29197),(#29198,
#29199),(#29200,#29201),(#29202,#29203),(#29204,#29205)),.UNSPECIFIED.,
 .F.,.F.,.F.)
B_SPLINE_SURFACE_WITH_KNOTS((6,1,1,1,1,1,1,1,1,1,1,1,1,1,1,1,1,1,1,1,1,
1,1,1,1,1,1,1,1,1,1,1,1,1,1,1,1,1,1,1,1,1,1,1,1,1,1,1,1,1,1,1,1,1,1,1,1,
1,1,1,1,1,1,1,1,6),(2,2),(-1.,-0.984615384615383,-0.969230769230768,-0.953846153846152,
-0.938461538461537,-0.923076923076922,-0.907692307692306,-0.892307692307691,
-0.876923076923076,-0.86153846153846,-0.846153846153845,-0.83076923076923,
-0.815384615384614,-0.799999999999999,-0.784615384615384,-0.769230769230768,
-0.753846153846153,-0.738461538461538,-0.723076923076922,-0.707692307692307,
-0.692307692307692,-0.676923076923076,-0.661538461538461,-0.646153846153846,
-0.63076923076923,-0.615384615384615,-0.6,-0.584615384615384,-0.569230769230769,
-0.553846153846154,-0.538461538461538,-0.523076923076923,-0.507692307692308,
-0.492307692307692,-0.476923076923077,-0.461538461538462,-0.446153846153846,
-0.430769230769231,-0.415384615384615,-0.4,-0.384615384615385,-0.369230769230769,
-0.353846153846154,-0.338461538461538,-0.323076923076923,-0.307692307692308,
-0.292307692307692,-0.276923076923077,-0.261538461538462,-0.246153846153846,
-0.230769230769231,-0.215384615384615,-0.2,-0.184615384615385,-0.169230769230769,
-0.153846153846154,-0.138461538461538,-0.123076923076923,-0.107692307692308,
-0.0923076923076923,-0.0769230769230769,-0.0615384615384615,-0.0461538461538462,
-0.0307692307692308,-0.0153846153846154,0.),(-1.,1.),.UNSPECIFIED.)
GEOMETRIC_REPRESENTATION_ITEM()
RATIONAL_B_SPLINE_SURFACE(((1.,1.),(1.,1.),(1.,1.),(1.,1.),(1.,1.),(1.,
1.),(1.,1.),(1.,1.),(1.,1.),(1.,1.),(1.,1.),(1.,1.),(1.,1.),(1.,1.),(1.,
1.),(1.,1.),(1.,1.),(1.,1.),(1.,1.),(1.,1.),(1.,1.),(1.,1.),(1.,1.),(1.,
1.),(1.,1.),(1.,1.),(1.,1.),(1.,1.),(1.,1.),(1.,1.),(1.,1.),(1.,1.),(1.,
1.),(1.,1.),(1.,1.),(1.,1.),(1.,1.),(1.,1.),(1.,1.),(1.,1.),(1.,1.),(1.,
1.),(1.,1.),(1.,1.),(1.,1.),(1.,1.),(1.,1.),(1.,1.),(1.,1.),(1.,1.),(1.,
1.),(1.,1.),(1.,1.),(1.,1.),(1.,1.),(1.,1.),(1.,1.),(1.,1.),(1.,1.),(1.,
1.),(1.,1.),(1.,1.),(1.,1.),(1.,1.),(1.,1.),(1.,1.),(1.,1.),(1.,1.),(1.,
1.),(1.,1.)))
REPRESENTATION_ITEM('')
SURFACE()
);
#30=(
BOUNDED_SURFACE()
B_SPLINE_SURFACE(5,1,((#29282,#29283),(#29284,#29285),(#29286,#29287),(#29288,
#29289),(#29290,#29291),(#29292,#29293),(#29294,#29295),(#29296,#29297),
(#29298,#29299),(#29300,#29301),(#29302,#29303),(#29304,#29305),(#29306,
#29307),(#29308,#29309),(#29310,#29311),(#29312,#29313),(#29314,#29315),
(#29316,#29317),(#29318,#29319),(#29320,#29321),(#29322,#29323),(#29324,
#29325),(#29326,#29327),(#29328,#29329),(#29330,#29331),(#29332,#29333),
(#29334,#29335),(#29336,#29337),(#29338,#29339),(#29340,#29341),(#29342,
#29343),(#29344,#29345),(#29346,#29347),(#29348,#29349),(#29350,#29351),
(#29352,#29353),(#29354,#29355),(#29356,#29357),(#29358,#29359),(#29360,
#29361),(#29362,#29363),(#29364,#29365),(#29366,#29367),(#29368,#29369),
(#29370,#29371),(#29372,#29373),(#29374,#29375),(#29376,#29377),(#29378,
#29379),(#29380,#29381),(#29382,#29383),(#29384,#29385),(#29386,#29387),
(#29388,#29389),(#29390,#29391),(#29392,#29393),(#29394,#29395),(#29396,
#29397),(#29398,#29399),(#29400,#29401),(#29402,#29403),(#29404,#29405),
(#29406,#29407),(#29408,#29409),(#29410,#29411),(#29412,#29413),(#29414,
#29415),(#29416,#29417),(#29418,#29419),(#29420,#29421)),.UNSPECIFIED.,
 .F.,.F.,.F.)
B_SPLINE_SURFACE_WITH_KNOTS((6,1,1,1,1,1,1,1,1,1,1,1,1,1,1,1,1,1,1,1,1,
1,1,1,1,1,1,1,1,1,1,1,1,1,1,1,1,1,1,1,1,1,1,1,1,1,1,1,1,1,1,1,1,1,1,1,1,
1,1,1,1,1,1,1,1,6),(2,2),(-1.,-0.984615384615383,-0.969230769230768,-0.953846153846152,
-0.938461538461537,-0.923076923076922,-0.907692307692306,-0.892307692307691,
-0.876923076923076,-0.86153846153846,-0.846153846153845,-0.83076923076923,
-0.815384615384614,-0.799999999999999,-0.784615384615384,-0.769230769230768,
-0.753846153846153,-0.738461538461538,-0.723076923076922,-0.707692307692307,
-0.692307692307692,-0.676923076923076,-0.661538461538461,-0.646153846153846,
-0.63076923076923,-0.615384615384615,-0.6,-0.584615384615384,-0.569230769230769,
-0.553846153846154,-0.538461538461538,-0.523076923076923,-0.507692307692308,
-0.492307692307692,-0.476923076923077,-0.461538461538462,-0.446153846153846,
-0.430769230769231,-0.415384615384615,-0.4,-0.384615384615385,-0.369230769230769,
-0.353846153846154,-0.338461538461538,-0.323076923076923,-0.307692307692308,
-0.292307692307692,-0.276923076923077,-0.261538461538462,-0.246153846153846,
-0.230769230769231,-0.215384615384615,-0.2,-0.184615384615385,-0.169230769230769,
-0.153846153846154,-0.138461538461538,-0.123076923076923,-0.107692307692308,
-0.0923076923076923,-0.0769230769230769,-0.0615384615384615,-0.0461538461538462,
-0.0307692307692308,-0.0153846153846154,0.),(-1.,1.),.UNSPECIFIED.)
GEOMETRIC_REPRESENTATION_ITEM()
RATIONAL_B_SPLINE_SURFACE(((1.,1.),(1.,1.),(1.,1.),(1.,1.),(1.,1.),(1.,
1.),(1.,1.),(1.,1.),(1.,1.),(1.,1.),(1.,1.),(1.,1.),(1.,1.),(1.,1.),(1.,
1.),(1.,1.),(1.,1.),(1.,1.),(1.,1.),(1.,1.),(1.,1.),(1.,1.),(1.,1.),(1.,
1.),(1.,1.),(1.,1.),(1.,1.),(1.,1.),(1.,1.),(1.,1.),(1.,1.),(1.,1.),(1.,
1.),(1.,1.),(1.,1.),(1.,1.),(1.,1.),(1.,1.),(1.,1.),(1.,1.),(1.,1.),(1.,
1.),(1.,1.),(1.,1.),(1.,1.),(1.,1.),(1.,1.),(1.,1.),(1.,1.),(1.,1.),(1.,
1.),(1.,1.),(1.,1.),(1.,1.),(1.,1.),(1.,1.),(1.,1.),(1.,1.),(1.,1.),(1.,
1.),(1.,1.),(1.,1.),(1.,1.),(1.,1.),(1.,1.),(1.,1.),(1.,1.),(1.,1.),(1.,
1.),(1.,1.)))
REPRESENTATION_ITEM('')
SURFACE()
);
#31=(
BOUNDED_SURFACE()
B_SPLINE_SURFACE(5,1,((#29498,#29499),(#29500,#29501),(#29502,#29503),(#29504,
#29505),(#29506,#29507),(#29508,#29509),(#29510,#29511),(#29512,#29513),
(#29514,#29515),(#29516,#29517),(#29518,#29519),(#29520,#29521),(#29522,
#29523),(#29524,#29525),(#29526,#29527),(#29528,#29529),(#29530,#29531),
(#29532,#29533),(#29534,#29535),(#29536,#29537),(#29538,#29539),(#29540,
#29541),(#29542,#29543),(#29544,#29545),(#29546,#29547),(#29548,#29549),
(#29550,#29551),(#29552,#29553),(#29554,#29555),(#29556,#29557),(#29558,
#29559),(#29560,#29561),(#29562,#29563),(#29564,#29565),(#29566,#29567),
(#29568,#29569),(#29570,#29571),(#29572,#29573),(#29574,#29575),(#29576,
#29577),(#29578,#29579),(#29580,#29581),(#29582,#29583),(#29584,#29585),
(#29586,#29587),(#29588,#29589),(#29590,#29591),(#29592,#29593),(#29594,
#29595),(#29596,#29597),(#29598,#29599),(#29600,#29601),(#29602,#29603),
(#29604,#29605),(#29606,#29607),(#29608,#29609),(#29610,#29611),(#29612,
#29613),(#29614,#29615),(#29616,#29617),(#29618,#29619),(#29620,#29621),
(#29622,#29623),(#29624,#29625),(#29626,#29627),(#29628,#29629),(#29630,
#29631),(#29632,#29633),(#29634,#29635),(#29636,#29637)),.UNSPECIFIED.,
 .F.,.F.,.F.)
B_SPLINE_SURFACE_WITH_KNOTS((6,1,1,1,1,1,1,1,1,1,1,1,1,1,1,1,1,1,1,1,1,
1,1,1,1,1,1,1,1,1,1,1,1,1,1,1,1,1,1,1,1,1,1,1,1,1,1,1,1,1,1,1,1,1,1,1,1,
1,1,1,1,1,1,1,1,6),(2,2),(-1.,-0.984615384615383,-0.969230769230768,-0.953846153846152,
-0.938461538461537,-0.923076923076922,-0.907692307692306,-0.892307692307691,
-0.876923076923076,-0.86153846153846,-0.846153846153845,-0.83076923076923,
-0.815384615384614,-0.799999999999999,-0.784615384615384,-0.769230769230768,
-0.753846153846153,-0.738461538461538,-0.723076923076922,-0.707692307692307,
-0.692307692307692,-0.676923076923076,-0.661538461538461,-0.646153846153846,
-0.63076923076923,-0.615384615384615,-0.6,-0.584615384615384,-0.569230769230769,
-0.553846153846154,-0.538461538461538,-0.523076923076923,-0.507692307692308,
-0.492307692307692,-0.476923076923077,-0.461538461538462,-0.446153846153846,
-0.430769230769231,-0.415384615384615,-0.4,-0.384615384615385,-0.369230769230769,
-0.353846153846154,-0.338461538461538,-0.323076923076923,-0.307692307692308,
-0.292307692307692,-0.276923076923077,-0.261538461538462,-0.246153846153846,
-0.230769230769231,-0.215384615384615,-0.2,-0.184615384615385,-0.169230769230769,
-0.153846153846154,-0.138461538461538,-0.123076923076923,-0.107692307692308,
-0.0923076923076923,-0.0769230769230769,-0.0615384615384615,-0.0461538461538462,
-0.0307692307692308,-0.0153846153846154,0.),(-1.,1.),.UNSPECIFIED.)
GEOMETRIC_REPRESENTATION_ITEM()
RATIONAL_B_SPLINE_SURFACE(((1.,1.),(1.,1.),(1.,1.),(1.,1.),(1.,1.),(1.,
1.),(1.,1.),(1.,1.),(1.,1.),(1.,1.),(1.,1.),(1.,1.),(1.,1.),(1.,1.),(1.,
1.),(1.,1.),(1.,1.),(1.,1.),(1.,1.),(1.,1.),(1.,1.),(1.,1.),(1.,1.),(1.,
1.),(1.,1.),(1.,1.),(1.,1.),(1.,1.),(1.,1.),(1.,1.),(1.,1.),(1.,1.),(1.,
1.),(1.,1.),(1.,1.),(1.,1.),(1.,1.),(1.,1.),(1.,1.),(1.,1.),(1.,1.),(1.,
1.),(1.,1.),(1.,1.),(1.,1.),(1.,1.),(1.,1.),(1.,1.),(1.,1.),(1.,1.),(1.,
1.),(1.,1.),(1.,1.),(1.,1.),(1.,1.),(1.,1.),(1.,1.),(1.,1.),(1.,1.),(1.,
1.),(1.,1.),(1.,1.),(1.,1.),(1.,1.),(1.,1.),(1.,1.),(1.,1.),(1.,1.),(1.,
1.),(1.,1.)))
REPRESENTATION_ITEM('')
SURFACE()
);
#32=(
BOUNDED_SURFACE()
B_SPLINE_SURFACE(5,1,((#29714,#29715),(#29716,#29717),(#29718,#29719),(#29720,
#29721),(#29722,#29723),(#29724,#29725),(#29726,#29727),(#29728,#29729),
(#29730,#29731),(#29732,#29733),(#29734,#29735),(#29736,#29737),(#29738,
#29739),(#29740,#29741),(#29742,#29743),(#29744,#29745),(#29746,#29747),
(#29748,#29749),(#29750,#29751),(#29752,#29753),(#29754,#29755),(#29756,
#29757),(#29758,#29759),(#29760,#29761),(#29762,#29763),(#29764,#29765),
(#29766,#29767),(#29768,#29769),(#29770,#29771),(#29772,#29773),(#29774,
#29775),(#29776,#29777),(#29778,#29779),(#29780,#29781),(#29782,#29783),
(#29784,#29785),(#29786,#29787),(#29788,#29789),(#29790,#29791),(#29792,
#29793),(#29794,#29795),(#29796,#29797),(#29798,#29799),(#29800,#29801),
(#29802,#29803),(#29804,#29805),(#29806,#29807),(#29808,#29809),(#29810,
#29811),(#29812,#29813),(#29814,#29815),(#29816,#29817),(#29818,#29819),
(#29820,#29821),(#29822,#29823),(#29824,#29825),(#29826,#29827),(#29828,
#29829),(#29830,#29831),(#29832,#29833),(#29834,#29835),(#29836,#29837),
(#29838,#29839),(#29840,#29841),(#29842,#29843),(#29844,#29845),(#29846,
#29847),(#29848,#29849),(#29850,#29851),(#29852,#29853)),.UNSPECIFIED.,
 .F.,.F.,.F.)
B_SPLINE_SURFACE_WITH_KNOTS((6,1,1,1,1,1,1,1,1,1,1,1,1,1,1,1,1,1,1,1,1,
1,1,1,1,1,1,1,1,1,1,1,1,1,1,1,1,1,1,1,1,1,1,1,1,1,1,1,1,1,1,1,1,1,1,1,1,
1,1,1,1,1,1,1,1,6),(2,2),(-1.,-0.984615384615383,-0.969230769230768,-0.953846153846152,
-0.938461538461537,-0.923076923076922,-0.907692307692306,-0.892307692307691,
-0.876923076923076,-0.86153846153846,-0.846153846153845,-0.83076923076923,
-0.815384615384614,-0.799999999999999,-0.784615384615384,-0.769230769230768,
-0.753846153846153,-0.738461538461538,-0.723076923076922,-0.707692307692307,
-0.692307692307692,-0.676923076923076,-0.661538461538461,-0.646153846153846,
-0.63076923076923,-0.615384615384615,-0.6,-0.584615384615384,-0.569230769230769,
-0.553846153846154,-0.538461538461538,-0.523076923076923,-0.507692307692308,
-0.492307692307692,-0.476923076923077,-0.461538461538462,-0.446153846153846,
-0.430769230769231,-0.415384615384615,-0.4,-0.384615384615385,-0.369230769230769,
-0.353846153846154,-0.338461538461538,-0.323076923076923,-0.307692307692308,
-0.292307692307692,-0.276923076923077,-0.261538461538462,-0.246153846153846,
-0.230769230769231,-0.215384615384615,-0.2,-0.184615384615385,-0.169230769230769,
-0.153846153846154,-0.138461538461538,-0.123076923076923,-0.107692307692308,
-0.0923076923076923,-0.0769230769230769,-0.0615384615384615,-0.0461538461538462,
-0.0307692307692308,-0.0153846153846154,0.),(-1.,1.),.UNSPECIFIED.)
GEOMETRIC_REPRESENTATION_ITEM()
RATIONAL_B_SPLINE_SURFACE(((1.,1.),(1.,1.),(1.,1.),(1.,1.),(1.,1.),(1.,
1.),(1.,1.),(1.,1.),(1.,1.),(1.,1.),(1.,1.),(1.,1.),(1.,1.),(1.,1.),(1.,
1.),(1.,1.),(1.,1.),(1.,1.),(1.,1.),(1.,1.),(1.,1.),(1.,1.),(1.,1.),(1.,
1.),(1.,1.),(1.,1.),(1.,1.),(1.,1.),(1.,1.),(1.,1.),(1.,1.),(1.,1.),(1.,
1.),(1.,1.),(1.,1.),(1.,1.),(1.,1.),(1.,1.),(1.,1.),(1.,1.),(1.,1.),(1.,
1.),(1.,1.),(1.,1.),(1.,1.),(1.,1.),(1.,1.),(1.,1.),(1.,1.),(1.,1.),(1.,
1.),(1.,1.),(1.,1.),(1.,1.),(1.,1.),(1.,1.),(1.,1.),(1.,1.),(1.,1.),(1.,
1.),(1.,1.),(1.,1.),(1.,1.),(1.,1.),(1.,1.),(1.,1.),(1.,1.),(1.,1.),(1.,
1.),(1.,1.)))
REPRESENTATION_ITEM('')
SURFACE()
);
#33=(
BOUNDED_SURFACE()
B_SPLINE_SURFACE(5,1,((#29930,#29931),(#29932,#29933),(#29934,#29935),(#29936,
#29937),(#29938,#29939),(#29940,#29941),(#29942,#29943),(#29944,#29945),
(#29946,#29947),(#29948,#29949),(#29950,#29951),(#29952,#29953),(#29954,
#29955),(#29956,#29957),(#29958,#29959),(#29960,#29961),(#29962,#29963),
(#29964,#29965),(#29966,#29967),(#29968,#29969),(#29970,#29971),(#29972,
#29973),(#29974,#29975),(#29976,#29977),(#29978,#29979),(#29980,#29981),
(#29982,#29983),(#29984,#29985),(#29986,#29987),(#29988,#29989),(#29990,
#29991),(#29992,#29993),(#29994,#29995),(#29996,#29997),(#29998,#29999),
(#30000,#30001),(#30002,#30003),(#30004,#30005),(#30006,#30007),(#30008,
#30009),(#30010,#30011),(#30012,#30013),(#30014,#30015),(#30016,#30017),
(#30018,#30019),(#30020,#30021),(#30022,#30023),(#30024,#30025),(#30026,
#30027),(#30028,#30029),(#30030,#30031),(#30032,#30033),(#30034,#30035),
(#30036,#30037),(#30038,#30039),(#30040,#30041),(#30042,#30043),(#30044,
#30045),(#30046,#30047),(#30048,#30049),(#30050,#30051),(#30052,#30053),
(#30054,#30055),(#30056,#30057),(#30058,#30059),(#30060,#30061),(#30062,
#30063),(#30064,#30065),(#30066,#30067),(#30068,#30069)),.UNSPECIFIED.,
 .F.,.F.,.F.)
B_SPLINE_SURFACE_WITH_KNOTS((6,1,1,1,1,1,1,1,1,1,1,1,1,1,1,1,1,1,1,1,1,
1,1,1,1,1,1,1,1,1,1,1,1,1,1,1,1,1,1,1,1,1,1,1,1,1,1,1,1,1,1,1,1,1,1,1,1,
1,1,1,1,1,1,1,1,6),(2,2),(-1.,-0.984615384615383,-0.969230769230768,-0.953846153846152,
-0.938461538461537,-0.923076923076922,-0.907692307692306,-0.892307692307691,
-0.876923076923076,-0.86153846153846,-0.846153846153845,-0.83076923076923,
-0.815384615384614,-0.799999999999999,-0.784615384615384,-0.769230769230768,
-0.753846153846153,-0.738461538461538,-0.723076923076922,-0.707692307692307,
-0.692307692307692,-0.676923076923076,-0.661538461538461,-0.646153846153846,
-0.63076923076923,-0.615384615384615,-0.6,-0.584615384615384,-0.569230769230769,
-0.553846153846154,-0.538461538461538,-0.523076923076923,-0.507692307692308,
-0.492307692307692,-0.476923076923077,-0.461538461538462,-0.446153846153846,
-0.430769230769231,-0.415384615384615,-0.4,-0.384615384615385,-0.369230769230769,
-0.353846153846154,-0.338461538461538,-0.323076923076923,-0.307692307692308,
-0.292307692307692,-0.276923076923077,-0.261538461538462,-0.246153846153846,
-0.230769230769231,-0.215384615384615,-0.2,-0.184615384615385,-0.169230769230769,
-0.153846153846154,-0.138461538461538,-0.123076923076923,-0.107692307692308,
-0.0923076923076923,-0.0769230769230769,-0.0615384615384615,-0.0461538461538462,
-0.0307692307692308,-0.0153846153846154,0.),(-1.,1.),.UNSPECIFIED.)
GEOMETRIC_REPRESENTATION_ITEM()
RATIONAL_B_SPLINE_SURFACE(((1.,1.),(1.,1.),(1.,1.),(1.,1.),(1.,1.),(1.,
1.),(1.,1.),(1.,1.),(1.,1.),(1.,1.),(1.,1.),(1.,1.),(1.,1.),(1.,1.),(1.,
1.),(1.,1.),(1.,1.),(1.,1.),(1.,1.),(1.,1.),(1.,1.),(1.,1.),(1.,1.),(1.,
1.),(1.,1.),(1.,1.),(1.,1.),(1.,1.),(1.,1.),(1.,1.),(1.,1.),(1.,1.),(1.,
1.),(1.,1.),(1.,1.),(1.,1.),(1.,1.),(1.,1.),(1.,1.),(1.,1.),(1.,1.),(1.,
1.),(1.,1.),(1.,1.),(1.,1.),(1.,1.),(1.,1.),(1.,1.),(1.,1.),(1.,1.),(1.,
1.),(1.,1.),(1.,1.),(1.,1.),(1.,1.),(1.,1.),(1.,1.),(1.,1.),(1.,1.),(1.,
1.),(1.,1.),(1.,1.),(1.,1.),(1.,1.),(1.,1.),(1.,1.),(1.,1.),(1.,1.),(1.,
1.),(1.,1.)))
REPRESENTATION_ITEM('')
SURFACE()
);
#34=(
BOUNDED_SURFACE()
B_SPLINE_SURFACE(5,1,((#30146,#30147),(#30148,#30149),(#30150,#30151),(#30152,
#30153),(#30154,#30155),(#30156,#30157),(#30158,#30159),(#30160,#30161),
(#30162,#30163),(#30164,#30165),(#30166,#30167),(#30168,#30169),(#30170,
#30171),(#30172,#30173),(#30174,#30175),(#30176,#30177),(#30178,#30179),
(#30180,#30181),(#30182,#30183),(#30184,#30185),(#30186,#30187),(#30188,
#30189),(#30190,#30191),(#30192,#30193),(#30194,#30195),(#30196,#30197),
(#30198,#30199),(#30200,#30201),(#30202,#30203),(#30204,#30205),(#30206,
#30207),(#30208,#30209),(#30210,#30211),(#30212,#30213),(#30214,#30215),
(#30216,#30217),(#30218,#30219),(#30220,#30221),(#30222,#30223),(#30224,
#30225),(#30226,#30227),(#30228,#30229),(#30230,#30231),(#30232,#30233),
(#30234,#30235),(#30236,#30237),(#30238,#30239),(#30240,#30241),(#30242,
#30243),(#30244,#30245),(#30246,#30247),(#30248,#30249),(#30250,#30251),
(#30252,#30253),(#30254,#30255),(#30256,#30257),(#30258,#30259),(#30260,
#30261),(#30262,#30263),(#30264,#30265),(#30266,#30267),(#30268,#30269),
(#30270,#30271),(#30272,#30273),(#30274,#30275),(#30276,#30277),(#30278,
#30279),(#30280,#30281),(#30282,#30283),(#30284,#30285)),.UNSPECIFIED.,
 .F.,.F.,.F.)
B_SPLINE_SURFACE_WITH_KNOTS((6,1,1,1,1,1,1,1,1,1,1,1,1,1,1,1,1,1,1,1,1,
1,1,1,1,1,1,1,1,1,1,1,1,1,1,1,1,1,1,1,1,1,1,1,1,1,1,1,1,1,1,1,1,1,1,1,1,
1,1,1,1,1,1,1,1,6),(2,2),(-1.,-0.984615384615383,-0.969230769230768,-0.953846153846152,
-0.938461538461537,-0.923076923076922,-0.907692307692306,-0.892307692307691,
-0.876923076923076,-0.86153846153846,-0.846153846153845,-0.83076923076923,
-0.815384615384614,-0.799999999999999,-0.784615384615384,-0.769230769230768,
-0.753846153846153,-0.738461538461538,-0.723076923076922,-0.707692307692307,
-0.692307692307692,-0.676923076923076,-0.661538461538461,-0.646153846153846,
-0.63076923076923,-0.615384615384615,-0.6,-0.584615384615384,-0.569230769230769,
-0.553846153846154,-0.538461538461538,-0.523076923076923,-0.507692307692308,
-0.492307692307692,-0.476923076923077,-0.461538461538462,-0.446153846153846,
-0.430769230769231,-0.415384615384615,-0.4,-0.384615384615385,-0.369230769230769,
-0.353846153846154,-0.338461538461538,-0.323076923076923,-0.307692307692308,
-0.292307692307692,-0.276923076923077,-0.261538461538462,-0.246153846153846,
-0.230769230769231,-0.215384615384615,-0.2,-0.184615384615385,-0.169230769230769,
-0.153846153846154,-0.138461538461538,-0.123076923076923,-0.107692307692308,
-0.0923076923076923,-0.0769230769230769,-0.0615384615384615,-0.0461538461538462,
-0.0307692307692308,-0.0153846153846154,0.),(-1.,1.),.UNSPECIFIED.)
GEOMETRIC_REPRESENTATION_ITEM()
RATIONAL_B_SPLINE_SURFACE(((1.,1.),(1.,1.),(1.,1.),(1.,1.),(1.,1.),(1.,
1.),(1.,1.),(1.,1.),(1.,1.),(1.,1.),(1.,1.),(1.,1.),(1.,1.),(1.,1.),(1.,
1.),(1.,1.),(1.,1.),(1.,1.),(1.,1.),(1.,1.),(1.,1.),(1.,1.),(1.,1.),(1.,
1.),(1.,1.),(1.,1.),(1.,1.),(1.,1.),(1.,1.),(1.,1.),(1.,1.),(1.,1.),(1.,
1.),(1.,1.),(1.,1.),(1.,1.),(1.,1.),(1.,1.),(1.,1.),(1.,1.),(1.,1.),(1.,
1.),(1.,1.),(1.,1.),(1.,1.),(1.,1.),(1.,1.),(1.,1.),(1.,1.),(1.,1.),(1.,
1.),(1.,1.),(1.,1.),(1.,1.),(1.,1.),(1.,1.),(1.,1.),(1.,1.),(1.,1.),(1.,
1.),(1.,1.),(1.,1.),(1.,1.),(1.,1.),(1.,1.),(1.,1.),(1.,1.),(1.,1.),(1.,
1.),(1.,1.)))
REPRESENTATION_ITEM('')
SURFACE()
);
#35=(
BOUNDED_SURFACE()
B_SPLINE_SURFACE(5,1,((#30362,#30363),(#30364,#30365),(#30366,#30367),(#30368,
#30369),(#30370,#30371),(#30372,#30373),(#30374,#30375),(#30376,#30377),
(#30378,#30379),(#30380,#30381),(#30382,#30383),(#30384,#30385),(#30386,
#30387),(#30388,#30389),(#30390,#30391),(#30392,#30393),(#30394,#30395),
(#30396,#30397),(#30398,#30399),(#30400,#30401),(#30402,#30403),(#30404,
#30405),(#30406,#30407),(#30408,#30409),(#30410,#30411),(#30412,#30413),
(#30414,#30415),(#30416,#30417),(#30418,#30419),(#30420,#30421),(#30422,
#30423),(#30424,#30425),(#30426,#30427),(#30428,#30429),(#30430,#30431),
(#30432,#30433),(#30434,#30435),(#30436,#30437),(#30438,#30439),(#30440,
#30441),(#30442,#30443),(#30444,#30445),(#30446,#30447),(#30448,#30449),
(#30450,#30451),(#30452,#30453),(#30454,#30455),(#30456,#30457),(#30458,
#30459),(#30460,#30461),(#30462,#30463),(#30464,#30465),(#30466,#30467),
(#30468,#30469),(#30470,#30471),(#30472,#30473),(#30474,#30475),(#30476,
#30477),(#30478,#30479),(#30480,#30481),(#30482,#30483),(#30484,#30485),
(#30486,#30487),(#30488,#30489),(#30490,#30491),(#30492,#30493),(#30494,
#30495),(#30496,#30497),(#30498,#30499),(#30500,#30501)),.UNSPECIFIED.,
 .F.,.F.,.F.)
B_SPLINE_SURFACE_WITH_KNOTS((6,1,1,1,1,1,1,1,1,1,1,1,1,1,1,1,1,1,1,1,1,
1,1,1,1,1,1,1,1,1,1,1,1,1,1,1,1,1,1,1,1,1,1,1,1,1,1,1,1,1,1,1,1,1,1,1,1,
1,1,1,1,1,1,1,1,6),(2,2),(-1.,-0.984615384615383,-0.969230769230768,-0.953846153846152,
-0.938461538461537,-0.923076923076922,-0.907692307692306,-0.892307692307691,
-0.876923076923076,-0.86153846153846,-0.846153846153845,-0.83076923076923,
-0.815384615384614,-0.799999999999999,-0.784615384615384,-0.769230769230768,
-0.753846153846153,-0.738461538461538,-0.723076923076922,-0.707692307692307,
-0.692307692307692,-0.676923076923076,-0.661538461538461,-0.646153846153846,
-0.63076923076923,-0.615384615384615,-0.6,-0.584615384615384,-0.569230769230769,
-0.553846153846154,-0.538461538461538,-0.523076923076923,-0.507692307692308,
-0.492307692307692,-0.476923076923077,-0.461538461538462,-0.446153846153846,
-0.430769230769231,-0.415384615384615,-0.4,-0.384615384615385,-0.369230769230769,
-0.353846153846154,-0.338461538461538,-0.323076923076923,-0.307692307692308,
-0.292307692307692,-0.276923076923077,-0.261538461538462,-0.246153846153846,
-0.230769230769231,-0.215384615384615,-0.2,-0.184615384615385,-0.169230769230769,
-0.153846153846154,-0.138461538461538,-0.123076923076923,-0.107692307692308,
-0.0923076923076923,-0.0769230769230769,-0.0615384615384615,-0.0461538461538462,
-0.0307692307692308,-0.0153846153846154,0.),(-1.,1.),.UNSPECIFIED.)
GEOMETRIC_REPRESENTATION_ITEM()
RATIONAL_B_SPLINE_SURFACE(((1.,1.),(1.,1.),(1.,1.),(1.,1.),(1.,1.),(1.,
1.),(1.,1.),(1.,1.),(1.,1.),(1.,1.),(1.,1.),(1.,1.),(1.,1.),(1.,1.),(1.,
1.),(1.,1.),(1.,1.),(1.,1.),(1.,1.),(1.,1.),(1.,1.),(1.,1.),(1.,1.),(1.,
1.),(1.,1.),(1.,1.),(1.,1.),(1.,1.),(1.,1.),(1.,1.),(1.,1.),(1.,1.),(1.,
1.),(1.,1.),(1.,1.),(1.,1.),(1.,1.),(1.,1.),(1.,1.),(1.,1.),(1.,1.),(1.,
1.),(1.,1.),(1.,1.),(1.,1.),(1.,1.),(1.,1.),(1.,1.),(1.,1.),(1.,1.),(1.,
1.),(1.,1.),(1.,1.),(1.,1.),(1.,1.),(1.,1.),(1.,1.),(1.,1.),(1.,1.),(1.,
1.),(1.,1.),(1.,1.),(1.,1.),(1.,1.),(1.,1.),(1.,1.),(1.,1.),(1.,1.),(1.,
1.),(1.,1.)))
REPRESENTATION_ITEM('')
SURFACE()
);
#36=(
BOUNDED_SURFACE()
B_SPLINE_SURFACE(5,1,((#30578,#30579),(#30580,#30581),(#30582,#30583),(#30584,
#30585),(#30586,#30587),(#30588,#30589),(#30590,#30591),(#30592,#30593),
(#30594,#30595),(#30596,#30597),(#30598,#30599),(#30600,#30601),(#30602,
#30603),(#30604,#30605),(#30606,#30607),(#30608,#30609),(#30610,#30611),
(#30612,#30613),(#30614,#30615),(#30616,#30617),(#30618,#30619),(#30620,
#30621),(#30622,#30623),(#30624,#30625),(#30626,#30627),(#30628,#30629),
(#30630,#30631),(#30632,#30633),(#30634,#30635),(#30636,#30637),(#30638,
#30639),(#30640,#30641),(#30642,#30643),(#30644,#30645),(#30646,#30647),
(#30648,#30649),(#30650,#30651),(#30652,#30653),(#30654,#30655),(#30656,
#30657),(#30658,#30659),(#30660,#30661),(#30662,#30663),(#30664,#30665),
(#30666,#30667),(#30668,#30669),(#30670,#30671),(#30672,#30673),(#30674,
#30675),(#30676,#30677),(#30678,#30679),(#30680,#30681),(#30682,#30683),
(#30684,#30685),(#30686,#30687),(#30688,#30689),(#30690,#30691),(#30692,
#30693),(#30694,#30695),(#30696,#30697),(#30698,#30699),(#30700,#30701),
(#30702,#30703),(#30704,#30705),(#30706,#30707),(#30708,#30709),(#30710,
#30711),(#30712,#30713),(#30714,#30715),(#30716,#30717)),.UNSPECIFIED.,
 .F.,.F.,.F.)
B_SPLINE_SURFACE_WITH_KNOTS((6,1,1,1,1,1,1,1,1,1,1,1,1,1,1,1,1,1,1,1,1,
1,1,1,1,1,1,1,1,1,1,1,1,1,1,1,1,1,1,1,1,1,1,1,1,1,1,1,1,1,1,1,1,1,1,1,1,
1,1,1,1,1,1,1,1,6),(2,2),(-1.,-0.984615384615383,-0.969230769230768,-0.953846153846152,
-0.938461538461537,-0.923076923076922,-0.907692307692306,-0.892307692307691,
-0.876923076923076,-0.86153846153846,-0.846153846153845,-0.83076923076923,
-0.815384615384614,-0.799999999999999,-0.784615384615384,-0.769230769230768,
-0.753846153846153,-0.738461538461538,-0.723076923076922,-0.707692307692307,
-0.692307692307692,-0.676923076923076,-0.661538461538461,-0.646153846153846,
-0.63076923076923,-0.615384615384615,-0.6,-0.584615384615384,-0.569230769230769,
-0.553846153846154,-0.538461538461538,-0.523076923076923,-0.507692307692308,
-0.492307692307692,-0.476923076923077,-0.461538461538462,-0.446153846153846,
-0.430769230769231,-0.415384615384615,-0.4,-0.384615384615385,-0.369230769230769,
-0.353846153846154,-0.338461538461538,-0.323076923076923,-0.307692307692308,
-0.292307692307692,-0.276923076923077,-0.261538461538462,-0.246153846153846,
-0.230769230769231,-0.215384615384615,-0.2,-0.184615384615385,-0.169230769230769,
-0.153846153846154,-0.138461538461538,-0.123076923076923,-0.107692307692308,
-0.0923076923076923,-0.0769230769230769,-0.0615384615384615,-0.0461538461538462,
-0.0307692307692308,-0.0153846153846154,0.),(-1.,1.),.UNSPECIFIED.)
GEOMETRIC_REPRESENTATION_ITEM()
RATIONAL_B_SPLINE_SURFACE(((1.,1.),(1.,1.),(1.,1.),(1.,1.),(1.,1.),(1.,
1.),(1.,1.),(1.,1.),(1.,1.),(1.,1.),(1.,1.),(1.,1.),(1.,1.),(1.,1.),(1.,
1.),(1.,1.),(1.,1.),(1.,1.),(1.,1.),(1.,1.),(1.,1.),(1.,1.),(1.,1.),(1.,
1.),(1.,1.),(1.,1.),(1.,1.),(1.,1.),(1.,1.),(1.,1.),(1.,1.),(1.,1.),(1.,
1.),(1.,1.),(1.,1.),(1.,1.),(1.,1.),(1.,1.),(1.,1.),(1.,1.),(1.,1.),(1.,
1.),(1.,1.),(1.,1.),(1.,1.),(1.,1.),(1.,1.),(1.,1.),(1.,1.),(1.,1.),(1.,
1.),(1.,1.),(1.,1.),(1.,1.),(1.,1.),(1.,1.),(1.,1.),(1.,1.),(1.,1.),(1.,
1.),(1.,1.),(1.,1.),(1.,1.),(1.,1.),(1.,1.),(1.,1.),(1.,1.),(1.,1.),(1.,
1.),(1.,1.)))
REPRESENTATION_ITEM('')
SURFACE()
);
#37=(
BOUNDED_SURFACE()
B_SPLINE_SURFACE(5,1,((#30794,#30795),(#30796,#30797),(#30798,#30799),(#30800,
#30801),(#30802,#30803),(#30804,#30805),(#30806,#30807),(#30808,#30809),
(#30810,#30811),(#30812,#30813),(#30814,#30815),(#30816,#30817),(#30818,
#30819),(#30820,#30821),(#30822,#30823),(#30824,#30825),(#30826,#30827),
(#30828,#30829),(#30830,#30831),(#30832,#30833),(#30834,#30835),(#30836,
#30837),(#30838,#30839),(#30840,#30841),(#30842,#30843),(#30844,#30845),
(#30846,#30847),(#30848,#30849),(#30850,#30851),(#30852,#30853),(#30854,
#30855),(#30856,#30857),(#30858,#30859),(#30860,#30861),(#30862,#30863),
(#30864,#30865),(#30866,#30867),(#30868,#30869),(#30870,#30871),(#30872,
#30873),(#30874,#30875),(#30876,#30877),(#30878,#30879),(#30880,#30881),
(#30882,#30883),(#30884,#30885),(#30886,#30887),(#30888,#30889),(#30890,
#30891),(#30892,#30893),(#30894,#30895),(#30896,#30897),(#30898,#30899),
(#30900,#30901),(#30902,#30903),(#30904,#30905),(#30906,#30907),(#30908,
#30909),(#30910,#30911),(#30912,#30913),(#30914,#30915),(#30916,#30917),
(#30918,#30919),(#30920,#30921),(#30922,#30923),(#30924,#30925),(#30926,
#30927),(#30928,#30929),(#30930,#30931),(#30932,#30933)),.UNSPECIFIED.,
 .F.,.F.,.F.)
B_SPLINE_SURFACE_WITH_KNOTS((6,1,1,1,1,1,1,1,1,1,1,1,1,1,1,1,1,1,1,1,1,
1,1,1,1,1,1,1,1,1,1,1,1,1,1,1,1,1,1,1,1,1,1,1,1,1,1,1,1,1,1,1,1,1,1,1,1,
1,1,1,1,1,1,1,1,6),(2,2),(-1.,-0.984615384615383,-0.969230769230768,-0.953846153846152,
-0.938461538461537,-0.923076923076922,-0.907692307692306,-0.892307692307691,
-0.876923076923076,-0.86153846153846,-0.846153846153845,-0.83076923076923,
-0.815384615384614,-0.799999999999999,-0.784615384615384,-0.769230769230768,
-0.753846153846153,-0.738461538461538,-0.723076923076922,-0.707692307692307,
-0.692307692307692,-0.676923076923076,-0.661538461538461,-0.646153846153846,
-0.63076923076923,-0.615384615384615,-0.6,-0.584615384615384,-0.569230769230769,
-0.553846153846154,-0.538461538461538,-0.523076923076923,-0.507692307692308,
-0.492307692307692,-0.476923076923077,-0.461538461538462,-0.446153846153846,
-0.430769230769231,-0.415384615384615,-0.4,-0.384615384615385,-0.369230769230769,
-0.353846153846154,-0.338461538461538,-0.323076923076923,-0.307692307692308,
-0.292307692307692,-0.276923076923077,-0.261538461538462,-0.246153846153846,
-0.230769230769231,-0.215384615384615,-0.2,-0.184615384615385,-0.169230769230769,
-0.153846153846154,-0.138461538461538,-0.123076923076923,-0.107692307692308,
-0.0923076923076923,-0.0769230769230769,-0.0615384615384615,-0.0461538461538462,
-0.0307692307692308,-0.0153846153846154,0.),(-1.,1.),.UNSPECIFIED.)
GEOMETRIC_REPRESENTATION_ITEM()
RATIONAL_B_SPLINE_SURFACE(((1.,1.),(1.,1.),(1.,1.),(1.,1.),(1.,1.),(1.,
1.),(1.,1.),(1.,1.),(1.,1.),(1.,1.),(1.,1.),(1.,1.),(1.,1.),(1.,1.),(1.,
1.),(1.,1.),(1.,1.),(1.,1.),(1.,1.),(1.,1.),(1.,1.),(1.,1.),(1.,1.),(1.,
1.),(1.,1.),(1.,1.),(1.,1.),(1.,1.),(1.,1.),(1.,1.),(1.,1.),(1.,1.),(1.,
1.),(1.,1.),(1.,1.),(1.,1.),(1.,1.),(1.,1.),(1.,1.),(1.,1.),(1.,1.),(1.,
1.),(1.,1.),(1.,1.),(1.,1.),(1.,1.),(1.,1.),(1.,1.),(1.,1.),(1.,1.),(1.,
1.),(1.,1.),(1.,1.),(1.,1.),(1.,1.),(1.,1.),(1.,1.),(1.,1.),(1.,1.),(1.,
1.),(1.,1.),(1.,1.),(1.,1.),(1.,1.),(1.,1.),(1.,1.),(1.,1.),(1.,1.),(1.,
1.),(1.,1.)))
REPRESENTATION_ITEM('')
SURFACE()
);
#38=(
BOUNDED_SURFACE()
B_SPLINE_SURFACE(5,1,((#31010,#31011),(#31012,#31013),(#31014,#31015),(#31016,
#31017),(#31018,#31019),(#31020,#31021),(#31022,#31023),(#31024,#31025),
(#31026,#31027),(#31028,#31029),(#31030,#31031),(#31032,#31033),(#31034,
#31035),(#31036,#31037),(#31038,#31039),(#31040,#31041),(#31042,#31043),
(#31044,#31045),(#31046,#31047),(#31048,#31049),(#31050,#31051),(#31052,
#31053),(#31054,#31055),(#31056,#31057),(#31058,#31059),(#31060,#31061),
(#31062,#31063),(#31064,#31065),(#31066,#31067),(#31068,#31069),(#31070,
#31071),(#31072,#31073),(#31074,#31075),(#31076,#31077),(#31078,#31079),
(#31080,#31081),(#31082,#31083),(#31084,#31085),(#31086,#31087),(#31088,
#31089),(#31090,#31091),(#31092,#31093),(#31094,#31095),(#31096,#31097),
(#31098,#31099),(#31100,#31101),(#31102,#31103),(#31104,#31105),(#31106,
#31107),(#31108,#31109),(#31110,#31111),(#31112,#31113),(#31114,#31115),
(#31116,#31117),(#31118,#31119),(#31120,#31121),(#31122,#31123),(#31124,
#31125),(#31126,#31127),(#31128,#31129),(#31130,#31131),(#31132,#31133),
(#31134,#31135),(#31136,#31137),(#31138,#31139),(#31140,#31141),(#31142,
#31143),(#31144,#31145),(#31146,#31147),(#31148,#31149)),.UNSPECIFIED.,
 .F.,.F.,.F.)
B_SPLINE_SURFACE_WITH_KNOTS((6,1,1,1,1,1,1,1,1,1,1,1,1,1,1,1,1,1,1,1,1,
1,1,1,1,1,1,1,1,1,1,1,1,1,1,1,1,1,1,1,1,1,1,1,1,1,1,1,1,1,1,1,1,1,1,1,1,
1,1,1,1,1,1,1,1,6),(2,2),(-1.,-0.984615384615383,-0.969230769230768,-0.953846153846152,
-0.938461538461537,-0.923076923076922,-0.907692307692306,-0.892307692307691,
-0.876923076923076,-0.86153846153846,-0.846153846153845,-0.83076923076923,
-0.815384615384614,-0.799999999999999,-0.784615384615384,-0.769230769230768,
-0.753846153846153,-0.738461538461538,-0.723076923076922,-0.707692307692307,
-0.692307692307692,-0.676923076923076,-0.661538461538461,-0.646153846153846,
-0.63076923076923,-0.615384615384615,-0.6,-0.584615384615384,-0.569230769230769,
-0.553846153846154,-0.538461538461538,-0.523076923076923,-0.507692307692308,
-0.492307692307692,-0.476923076923077,-0.461538461538462,-0.446153846153846,
-0.430769230769231,-0.415384615384615,-0.4,-0.384615384615385,-0.369230769230769,
-0.353846153846154,-0.338461538461538,-0.323076923076923,-0.307692307692308,
-0.292307692307692,-0.276923076923077,-0.261538461538462,-0.246153846153846,
-0.230769230769231,-0.215384615384615,-0.2,-0.184615384615385,-0.169230769230769,
-0.153846153846154,-0.138461538461538,-0.123076923076923,-0.107692307692308,
-0.0923076923076923,-0.0769230769230769,-0.0615384615384615,-0.0461538461538462,
-0.0307692307692308,-0.0153846153846154,0.),(-1.,1.),.UNSPECIFIED.)
GEOMETRIC_REPRESENTATION_ITEM()
RATIONAL_B_SPLINE_SURFACE(((1.,1.),(1.,1.),(1.,1.),(1.,1.),(1.,1.),(1.,
1.),(1.,1.),(1.,1.),(1.,1.),(1.,1.),(1.,1.),(1.,1.),(1.,1.),(1.,1.),(1.,
1.),(1.,1.),(1.,1.),(1.,1.),(1.,1.),(1.,1.),(1.,1.),(1.,1.),(1.,1.),(1.,
1.),(1.,1.),(1.,1.),(1.,1.),(1.,1.),(1.,1.),(1.,1.),(1.,1.),(1.,1.),(1.,
1.),(1.,1.),(1.,1.),(1.,1.),(1.,1.),(1.,1.),(1.,1.),(1.,1.),(1.,1.),(1.,
1.),(1.,1.),(1.,1.),(1.,1.),(1.,1.),(1.,1.),(1.,1.),(1.,1.),(1.,1.),(1.,
1.),(1.,1.),(1.,1.),(1.,1.),(1.,1.),(1.,1.),(1.,1.),(1.,1.),(1.,1.),(1.,
1.),(1.,1.),(1.,1.),(1.,1.),(1.,1.),(1.,1.),(1.,1.),(1.,1.),(1.,1.),(1.,
1.),(1.,1.)))
REPRESENTATION_ITEM('')
SURFACE()
);
#39=(
BOUNDED_SURFACE()
B_SPLINE_SURFACE(5,1,((#31226,#31227),(#31228,#31229),(#31230,#31231),(#31232,
#31233),(#31234,#31235),(#31236,#31237),(#31238,#31239),(#31240,#31241),
(#31242,#31243),(#31244,#31245),(#31246,#31247),(#31248,#31249),(#31250,
#31251),(#31252,#31253),(#31254,#31255),(#31256,#31257),(#31258,#31259),
(#31260,#31261),(#31262,#31263),(#31264,#31265),(#31266,#31267),(#31268,
#31269),(#31270,#31271),(#31272,#31273),(#31274,#31275),(#31276,#31277),
(#31278,#31279),(#31280,#31281),(#31282,#31283),(#31284,#31285),(#31286,
#31287),(#31288,#31289),(#31290,#31291),(#31292,#31293),(#31294,#31295),
(#31296,#31297),(#31298,#31299),(#31300,#31301),(#31302,#31303),(#31304,
#31305),(#31306,#31307),(#31308,#31309),(#31310,#31311),(#31312,#31313),
(#31314,#31315),(#31316,#31317),(#31318,#31319),(#31320,#31321),(#31322,
#31323),(#31324,#31325),(#31326,#31327),(#31328,#31329),(#31330,#31331),
(#31332,#31333),(#31334,#31335),(#31336,#31337),(#31338,#31339),(#31340,
#31341),(#31342,#31343),(#31344,#31345),(#31346,#31347),(#31348,#31349),
(#31350,#31351),(#31352,#31353),(#31354,#31355),(#31356,#31357),(#31358,
#31359),(#31360,#31361),(#31362,#31363),(#31364,#31365)),.UNSPECIFIED.,
 .F.,.F.,.F.)
B_SPLINE_SURFACE_WITH_KNOTS((6,1,1,1,1,1,1,1,1,1,1,1,1,1,1,1,1,1,1,1,1,
1,1,1,1,1,1,1,1,1,1,1,1,1,1,1,1,1,1,1,1,1,1,1,1,1,1,1,1,1,1,1,1,1,1,1,1,
1,1,1,1,1,1,1,1,6),(2,2),(-1.,-0.984615384615383,-0.969230769230768,-0.953846153846152,
-0.938461538461537,-0.923076923076922,-0.907692307692306,-0.892307692307691,
-0.876923076923076,-0.86153846153846,-0.846153846153845,-0.83076923076923,
-0.815384615384614,-0.799999999999999,-0.784615384615384,-0.769230769230768,
-0.753846153846153,-0.738461538461538,-0.723076923076922,-0.707692307692307,
-0.692307692307692,-0.676923076923076,-0.661538461538461,-0.646153846153846,
-0.63076923076923,-0.615384615384615,-0.6,-0.584615384615384,-0.569230769230769,
-0.553846153846154,-0.538461538461538,-0.523076923076923,-0.507692307692308,
-0.492307692307692,-0.476923076923077,-0.461538461538462,-0.446153846153846,
-0.430769230769231,-0.415384615384615,-0.4,-0.384615384615385,-0.369230769230769,
-0.353846153846154,-0.338461538461538,-0.323076923076923,-0.307692307692308,
-0.292307692307692,-0.276923076923077,-0.261538461538462,-0.246153846153846,
-0.230769230769231,-0.215384615384615,-0.2,-0.184615384615385,-0.169230769230769,
-0.153846153846154,-0.138461538461538,-0.123076923076923,-0.107692307692308,
-0.0923076923076923,-0.0769230769230769,-0.0615384615384615,-0.0461538461538462,
-0.0307692307692308,-0.0153846153846154,0.),(-1.,1.),.UNSPECIFIED.)
GEOMETRIC_REPRESENTATION_ITEM()
RATIONAL_B_SPLINE_SURFACE(((1.,1.),(1.,1.),(1.,1.),(1.,1.),(1.,1.),(1.,
1.),(1.,1.),(1.,1.),(1.,1.),(1.,1.),(1.,1.),(1.,1.),(1.,1.),(1.,1.),(1.,
1.),(1.,1.),(1.,1.),(1.,1.),(1.,1.),(1.,1.),(1.,1.),(1.,1.),(1.,1.),(1.,
1.),(1.,1.),(1.,1.),(1.,1.),(1.,1.),(1.,1.),(1.,1.),(1.,1.),(1.,1.),(1.,
1.),(1.,1.),(1.,1.),(1.,1.),(1.,1.),(1.,1.),(1.,1.),(1.,1.),(1.,1.),(1.,
1.),(1.,1.),(1.,1.),(1.,1.),(1.,1.),(1.,1.),(1.,1.),(1.,1.),(1.,1.),(1.,
1.),(1.,1.),(1.,1.),(1.,1.),(1.,1.),(1.,1.),(1.,1.),(1.,1.),(1.,1.),(1.,
1.),(1.,1.),(1.,1.),(1.,1.),(1.,1.),(1.,1.),(1.,1.),(1.,1.),(1.,1.),(1.,
1.),(1.,1.)))
REPRESENTATION_ITEM('')
SURFACE()
);
#40=(
BOUNDED_SURFACE()
B_SPLINE_SURFACE(5,1,((#31442,#31443),(#31444,#31445),(#31446,#31447),(#31448,
#31449),(#31450,#31451),(#31452,#31453),(#31454,#31455),(#31456,#31457),
(#31458,#31459),(#31460,#31461),(#31462,#31463),(#31464,#31465),(#31466,
#31467),(#31468,#31469),(#31470,#31471),(#31472,#31473),(#31474,#31475),
(#31476,#31477),(#31478,#31479),(#31480,#31481),(#31482,#31483),(#31484,
#31485),(#31486,#31487),(#31488,#31489),(#31490,#31491),(#31492,#31493),
(#31494,#31495),(#31496,#31497),(#31498,#31499),(#31500,#31501),(#31502,
#31503),(#31504,#31505),(#31506,#31507),(#31508,#31509),(#31510,#31511),
(#31512,#31513),(#31514,#31515),(#31516,#31517),(#31518,#31519),(#31520,
#31521),(#31522,#31523),(#31524,#31525),(#31526,#31527),(#31528,#31529),
(#31530,#31531),(#31532,#31533),(#31534,#31535),(#31536,#31537),(#31538,
#31539),(#31540,#31541),(#31542,#31543),(#31544,#31545),(#31546,#31547),
(#31548,#31549),(#31550,#31551),(#31552,#31553),(#31554,#31555),(#31556,
#31557),(#31558,#31559),(#31560,#31561),(#31562,#31563),(#31564,#31565),
(#31566,#31567),(#31568,#31569),(#31570,#31571),(#31572,#31573),(#31574,
#31575),(#31576,#31577),(#31578,#31579),(#31580,#31581)),.UNSPECIFIED.,
 .F.,.F.,.F.)
B_SPLINE_SURFACE_WITH_KNOTS((6,1,1,1,1,1,1,1,1,1,1,1,1,1,1,1,1,1,1,1,1,
1,1,1,1,1,1,1,1,1,1,1,1,1,1,1,1,1,1,1,1,1,1,1,1,1,1,1,1,1,1,1,1,1,1,1,1,
1,1,1,1,1,1,1,1,6),(2,2),(-1.,-0.984615384615383,-0.969230769230768,-0.953846153846152,
-0.938461538461537,-0.923076923076922,-0.907692307692306,-0.892307692307691,
-0.876923076923076,-0.86153846153846,-0.846153846153845,-0.83076923076923,
-0.815384615384614,-0.799999999999999,-0.784615384615384,-0.769230769230768,
-0.753846153846153,-0.738461538461538,-0.723076923076922,-0.707692307692307,
-0.692307692307692,-0.676923076923076,-0.661538461538461,-0.646153846153846,
-0.63076923076923,-0.615384615384615,-0.6,-0.584615384615384,-0.569230769230769,
-0.553846153846154,-0.538461538461538,-0.523076923076923,-0.507692307692308,
-0.492307692307692,-0.476923076923077,-0.461538461538462,-0.446153846153846,
-0.430769230769231,-0.415384615384615,-0.4,-0.384615384615385,-0.369230769230769,
-0.353846153846154,-0.338461538461538,-0.323076923076923,-0.307692307692308,
-0.292307692307692,-0.276923076923077,-0.261538461538462,-0.246153846153846,
-0.230769230769231,-0.215384615384615,-0.2,-0.184615384615385,-0.169230769230769,
-0.153846153846154,-0.138461538461538,-0.123076923076923,-0.107692307692308,
-0.0923076923076923,-0.0769230769230769,-0.0615384615384615,-0.0461538461538462,
-0.0307692307692308,-0.0153846153846154,0.),(-1.,1.),.UNSPECIFIED.)
GEOMETRIC_REPRESENTATION_ITEM()
RATIONAL_B_SPLINE_SURFACE(((1.,1.),(1.,1.),(1.,1.),(1.,1.),(1.,1.),(1.,
1.),(1.,1.),(1.,1.),(1.,1.),(1.,1.),(1.,1.),(1.,1.),(1.,1.),(1.,1.),(1.,
1.),(1.,1.),(1.,1.),(1.,1.),(1.,1.),(1.,1.),(1.,1.),(1.,1.),(1.,1.),(1.,
1.),(1.,1.),(1.,1.),(1.,1.),(1.,1.),(1.,1.),(1.,1.),(1.,1.),(1.,1.),(1.,
1.),(1.,1.),(1.,1.),(1.,1.),(1.,1.),(1.,1.),(1.,1.),(1.,1.),(1.,1.),(1.,
1.),(1.,1.),(1.,1.),(1.,1.),(1.,1.),(1.,1.),(1.,1.),(1.,1.),(1.,1.),(1.,
1.),(1.,1.),(1.,1.),(1.,1.),(1.,1.),(1.,1.),(1.,1.),(1.,1.),(1.,1.),(1.,
1.),(1.,1.),(1.,1.),(1.,1.),(1.,1.),(1.,1.),(1.,1.),(1.,1.),(1.,1.),(1.,
1.),(1.,1.)))
REPRESENTATION_ITEM('')
SURFACE()
);
#41=(
BOUNDED_SURFACE()
B_SPLINE_SURFACE(5,1,((#31658,#31659),(#31660,#31661),(#31662,#31663),(#31664,
#31665),(#31666,#31667),(#31668,#31669),(#31670,#31671),(#31672,#31673),
(#31674,#31675),(#31676,#31677),(#31678,#31679),(#31680,#31681),(#31682,
#31683),(#31684,#31685),(#31686,#31687),(#31688,#31689),(#31690,#31691),
(#31692,#31693),(#31694,#31695),(#31696,#31697),(#31698,#31699),(#31700,
#31701),(#31702,#31703),(#31704,#31705),(#31706,#31707),(#31708,#31709),
(#31710,#31711),(#31712,#31713),(#31714,#31715),(#31716,#31717),(#31718,
#31719),(#31720,#31721),(#31722,#31723),(#31724,#31725),(#31726,#31727),
(#31728,#31729),(#31730,#31731),(#31732,#31733),(#31734,#31735),(#31736,
#31737),(#31738,#31739),(#31740,#31741),(#31742,#31743),(#31744,#31745),
(#31746,#31747),(#31748,#31749),(#31750,#31751),(#31752,#31753),(#31754,
#31755),(#31756,#31757),(#31758,#31759),(#31760,#31761),(#31762,#31763),
(#31764,#31765),(#31766,#31767),(#31768,#31769),(#31770,#31771),(#31772,
#31773),(#31774,#31775),(#31776,#31777),(#31778,#31779),(#31780,#31781),
(#31782,#31783),(#31784,#31785),(#31786,#31787),(#31788,#31789),(#31790,
#31791),(#31792,#31793),(#31794,#31795),(#31796,#31797)),.UNSPECIFIED.,
 .F.,.F.,.F.)
B_SPLINE_SURFACE_WITH_KNOTS((6,1,1,1,1,1,1,1,1,1,1,1,1,1,1,1,1,1,1,1,1,
1,1,1,1,1,1,1,1,1,1,1,1,1,1,1,1,1,1,1,1,1,1,1,1,1,1,1,1,1,1,1,1,1,1,1,1,
1,1,1,1,1,1,1,1,6),(2,2),(-1.,-0.984615384615383,-0.969230769230768,-0.953846153846152,
-0.938461538461537,-0.923076923076922,-0.907692307692306,-0.892307692307691,
-0.876923076923076,-0.86153846153846,-0.846153846153845,-0.83076923076923,
-0.815384615384614,-0.799999999999999,-0.784615384615384,-0.769230769230768,
-0.753846153846153,-0.738461538461538,-0.723076923076922,-0.707692307692307,
-0.692307692307692,-0.676923076923076,-0.661538461538461,-0.646153846153846,
-0.63076923076923,-0.615384615384615,-0.6,-0.584615384615384,-0.569230769230769,
-0.553846153846154,-0.538461538461538,-0.523076923076923,-0.507692307692308,
-0.492307692307692,-0.476923076923077,-0.461538461538462,-0.446153846153846,
-0.430769230769231,-0.415384615384615,-0.4,-0.384615384615385,-0.369230769230769,
-0.353846153846154,-0.338461538461538,-0.323076923076923,-0.307692307692308,
-0.292307692307692,-0.276923076923077,-0.261538461538462,-0.246153846153846,
-0.230769230769231,-0.215384615384615,-0.2,-0.184615384615385,-0.169230769230769,
-0.153846153846154,-0.138461538461538,-0.123076923076923,-0.107692307692308,
-0.0923076923076923,-0.0769230769230769,-0.0615384615384615,-0.0461538461538462,
-0.0307692307692308,-0.0153846153846154,0.),(-1.,1.),.UNSPECIFIED.)
GEOMETRIC_REPRESENTATION_ITEM()
RATIONAL_B_SPLINE_SURFACE(((1.,1.),(1.,1.),(1.,1.),(1.,1.),(1.,1.),(1.,
1.),(1.,1.),(1.,1.),(1.,1.),(1.,1.),(1.,1.),(1.,1.),(1.,1.),(1.,1.),(1.,
1.),(1.,1.),(1.,1.),(1.,1.),(1.,1.),(1.,1.),(1.,1.),(1.,1.),(1.,1.),(1.,
1.),(1.,1.),(1.,1.),(1.,1.),(1.,1.),(1.,1.),(1.,1.),(1.,1.),(1.,1.),(1.,
1.),(1.,1.),(1.,1.),(1.,1.),(1.,1.),(1.,1.),(1.,1.),(1.,1.),(1.,1.),(1.,
1.),(1.,1.),(1.,1.),(1.,1.),(1.,1.),(1.,1.),(1.,1.),(1.,1.),(1.,1.),(1.,
1.),(1.,1.),(1.,1.),(1.,1.),(1.,1.),(1.,1.),(1.,1.),(1.,1.),(1.,1.),(1.,
1.),(1.,1.),(1.,1.),(1.,1.),(1.,1.),(1.,1.),(1.,1.),(1.,1.),(1.,1.),(1.,
1.),(1.,1.)))
REPRESENTATION_ITEM('')
SURFACE()
);
#42=(
BOUNDED_SURFACE()
B_SPLINE_SURFACE(5,1,((#31874,#31875),(#31876,#31877),(#31878,#31879),(#31880,
#31881),(#31882,#31883),(#31884,#31885),(#31886,#31887),(#31888,#31889),
(#31890,#31891),(#31892,#31893),(#31894,#31895),(#31896,#31897),(#31898,
#31899),(#31900,#31901),(#31902,#31903),(#31904,#31905),(#31906,#31907),
(#31908,#31909),(#31910,#31911),(#31912,#31913),(#31914,#31915),(#31916,
#31917),(#31918,#31919),(#31920,#31921),(#31922,#31923),(#31924,#31925),
(#31926,#31927),(#31928,#31929),(#31930,#31931),(#31932,#31933),(#31934,
#31935),(#31936,#31937),(#31938,#31939),(#31940,#31941),(#31942,#31943),
(#31944,#31945),(#31946,#31947),(#31948,#31949),(#31950,#31951),(#31952,
#31953),(#31954,#31955),(#31956,#31957),(#31958,#31959),(#31960,#31961),
(#31962,#31963),(#31964,#31965),(#31966,#31967),(#31968,#31969),(#31970,
#31971),(#31972,#31973),(#31974,#31975),(#31976,#31977),(#31978,#31979),
(#31980,#31981),(#31982,#31983),(#31984,#31985),(#31986,#31987),(#31988,
#31989),(#31990,#31991),(#31992,#31993),(#31994,#31995),(#31996,#31997),
(#31998,#31999),(#32000,#32001),(#32002,#32003),(#32004,#32005),(#32006,
#32007),(#32008,#32009),(#32010,#32011),(#32012,#32013)),.UNSPECIFIED.,
 .F.,.F.,.F.)
B_SPLINE_SURFACE_WITH_KNOTS((6,1,1,1,1,1,1,1,1,1,1,1,1,1,1,1,1,1,1,1,1,
1,1,1,1,1,1,1,1,1,1,1,1,1,1,1,1,1,1,1,1,1,1,1,1,1,1,1,1,1,1,1,1,1,1,1,1,
1,1,1,1,1,1,1,1,6),(2,2),(-1.,-0.984615384615383,-0.969230769230768,-0.953846153846152,
-0.938461538461537,-0.923076923076922,-0.907692307692306,-0.892307692307691,
-0.876923076923076,-0.86153846153846,-0.846153846153845,-0.83076923076923,
-0.815384615384614,-0.799999999999999,-0.784615384615384,-0.769230769230768,
-0.753846153846153,-0.738461538461538,-0.723076923076922,-0.707692307692307,
-0.692307692307692,-0.676923076923076,-0.661538461538461,-0.646153846153846,
-0.63076923076923,-0.615384615384615,-0.6,-0.584615384615384,-0.569230769230769,
-0.553846153846154,-0.538461538461538,-0.523076923076923,-0.507692307692308,
-0.492307692307692,-0.476923076923077,-0.461538461538462,-0.446153846153846,
-0.430769230769231,-0.415384615384615,-0.4,-0.384615384615385,-0.369230769230769,
-0.353846153846154,-0.338461538461538,-0.323076923076923,-0.307692307692308,
-0.292307692307692,-0.276923076923077,-0.261538461538462,-0.246153846153846,
-0.230769230769231,-0.215384615384615,-0.2,-0.184615384615385,-0.169230769230769,
-0.153846153846154,-0.138461538461538,-0.123076923076923,-0.107692307692308,
-0.0923076923076923,-0.0769230769230769,-0.0615384615384615,-0.0461538461538462,
-0.0307692307692308,-0.0153846153846154,0.),(-1.,1.),.UNSPECIFIED.)
GEOMETRIC_REPRESENTATION_ITEM()
RATIONAL_B_SPLINE_SURFACE(((1.,1.),(1.,1.),(1.,1.),(1.,1.),(1.,1.),(1.,
1.),(1.,1.),(1.,1.),(1.,1.),(1.,1.),(1.,1.),(1.,1.),(1.,1.),(1.,1.),(1.,
1.),(1.,1.),(1.,1.),(1.,1.),(1.,1.),(1.,1.),(1.,1.),(1.,1.),(1.,1.),(1.,
1.),(1.,1.),(1.,1.),(1.,1.),(1.,1.),(1.,1.),(1.,1.),(1.,1.),(1.,1.),(1.,
1.),(1.,1.),(1.,1.),(1.,1.),(1.,1.),(1.,1.),(1.,1.),(1.,1.),(1.,1.),(1.,
1.),(1.,1.),(1.,1.),(1.,1.),(1.,1.),(1.,1.),(1.,1.),(1.,1.),(1.,1.),(1.,
1.),(1.,1.),(1.,1.),(1.,1.),(1.,1.),(1.,1.),(1.,1.),(1.,1.),(1.,1.),(1.,
1.),(1.,1.),(1.,1.),(1.,1.),(1.,1.),(1.,1.),(1.,1.),(1.,1.),(1.,1.),(1.,
1.),(1.,1.)))
REPRESENTATION_ITEM('')
SURFACE()
);
#43=(
BOUNDED_SURFACE()
B_SPLINE_SURFACE(5,1,((#32090,#32091),(#32092,#32093),(#32094,#32095),(#32096,
#32097),(#32098,#32099),(#32100,#32101),(#32102,#32103),(#32104,#32105),
(#32106,#32107),(#32108,#32109),(#32110,#32111),(#32112,#32113),(#32114,
#32115),(#32116,#32117),(#32118,#32119),(#32120,#32121),(#32122,#32123),
(#32124,#32125),(#32126,#32127),(#32128,#32129),(#32130,#32131),(#32132,
#32133),(#32134,#32135),(#32136,#32137),(#32138,#32139),(#32140,#32141),
(#32142,#32143),(#32144,#32145),(#32146,#32147),(#32148,#32149),(#32150,
#32151),(#32152,#32153),(#32154,#32155),(#32156,#32157),(#32158,#32159),
(#32160,#32161),(#32162,#32163),(#32164,#32165),(#32166,#32167),(#32168,
#32169),(#32170,#32171),(#32172,#32173),(#32174,#32175),(#32176,#32177),
(#32178,#32179),(#32180,#32181),(#32182,#32183),(#32184,#32185),(#32186,
#32187),(#32188,#32189),(#32190,#32191),(#32192,#32193),(#32194,#32195),
(#32196,#32197),(#32198,#32199),(#32200,#32201),(#32202,#32203),(#32204,
#32205),(#32206,#32207),(#32208,#32209),(#32210,#32211),(#32212,#32213),
(#32214,#32215),(#32216,#32217),(#32218,#32219),(#32220,#32221),(#32222,
#32223),(#32224,#32225),(#32226,#32227),(#32228,#32229)),.UNSPECIFIED.,
 .F.,.F.,.F.)
B_SPLINE_SURFACE_WITH_KNOTS((6,1,1,1,1,1,1,1,1,1,1,1,1,1,1,1,1,1,1,1,1,
1,1,1,1,1,1,1,1,1,1,1,1,1,1,1,1,1,1,1,1,1,1,1,1,1,1,1,1,1,1,1,1,1,1,1,1,
1,1,1,1,1,1,1,1,6),(2,2),(-1.,-0.984615384615383,-0.969230769230768,-0.953846153846152,
-0.938461538461537,-0.923076923076922,-0.907692307692306,-0.892307692307691,
-0.876923076923076,-0.86153846153846,-0.846153846153845,-0.83076923076923,
-0.815384615384614,-0.799999999999999,-0.784615384615384,-0.769230769230768,
-0.753846153846153,-0.738461538461538,-0.723076923076922,-0.707692307692307,
-0.692307692307692,-0.676923076923076,-0.661538461538461,-0.646153846153846,
-0.63076923076923,-0.615384615384615,-0.6,-0.584615384615384,-0.569230769230769,
-0.553846153846154,-0.538461538461538,-0.523076923076923,-0.507692307692308,
-0.492307692307692,-0.476923076923077,-0.461538461538462,-0.446153846153846,
-0.430769230769231,-0.415384615384615,-0.4,-0.384615384615385,-0.369230769230769,
-0.353846153846154,-0.338461538461538,-0.323076923076923,-0.307692307692308,
-0.292307692307692,-0.276923076923077,-0.261538461538462,-0.246153846153846,
-0.230769230769231,-0.215384615384615,-0.2,-0.184615384615385,-0.169230769230769,
-0.153846153846154,-0.138461538461538,-0.123076923076923,-0.107692307692308,
-0.0923076923076923,-0.0769230769230769,-0.0615384615384615,-0.0461538461538462,
-0.0307692307692308,-0.0153846153846154,0.),(-1.,1.),.UNSPECIFIED.)
GEOMETRIC_REPRESENTATION_ITEM()
RATIONAL_B_SPLINE_SURFACE(((1.,1.),(1.,1.),(1.,1.),(1.,1.),(1.,1.),(1.,
1.),(1.,1.),(1.,1.),(1.,1.),(1.,1.),(1.,1.),(1.,1.),(1.,1.),(1.,1.),(1.,
1.),(1.,1.),(1.,1.),(1.,1.),(1.,1.),(1.,1.),(1.,1.),(1.,1.),(1.,1.),(1.,
1.),(1.,1.),(1.,1.),(1.,1.),(1.,1.),(1.,1.),(1.,1.),(1.,1.),(1.,1.),(1.,
1.),(1.,1.),(1.,1.),(1.,1.),(1.,1.),(1.,1.),(1.,1.),(1.,1.),(1.,1.),(1.,
1.),(1.,1.),(1.,1.),(1.,1.),(1.,1.),(1.,1.),(1.,1.),(1.,1.),(1.,1.),(1.,
1.),(1.,1.),(1.,1.),(1.,1.),(1.,1.),(1.,1.),(1.,1.),(1.,1.),(1.,1.),(1.,
1.),(1.,1.),(1.,1.),(1.,1.),(1.,1.),(1.,1.),(1.,1.),(1.,1.),(1.,1.),(1.,
1.),(1.,1.)))
REPRESENTATION_ITEM('')
SURFACE()
);
#44=(
BOUNDED_SURFACE()
B_SPLINE_SURFACE(5,1,((#32306,#32307),(#32308,#32309),(#32310,#32311),(#32312,
#32313),(#32314,#32315),(#32316,#32317),(#32318,#32319),(#32320,#32321),
(#32322,#32323),(#32324,#32325),(#32326,#32327),(#32328,#32329),(#32330,
#32331),(#32332,#32333),(#32334,#32335),(#32336,#32337),(#32338,#32339),
(#32340,#32341),(#32342,#32343),(#32344,#32345),(#32346,#32347),(#32348,
#32349),(#32350,#32351),(#32352,#32353),(#32354,#32355),(#32356,#32357),
(#32358,#32359),(#32360,#32361),(#32362,#32363),(#32364,#32365),(#32366,
#32367),(#32368,#32369),(#32370,#32371),(#32372,#32373),(#32374,#32375),
(#32376,#32377),(#32378,#32379),(#32380,#32381),(#32382,#32383),(#32384,
#32385),(#32386,#32387),(#32388,#32389),(#32390,#32391),(#32392,#32393),
(#32394,#32395),(#32396,#32397),(#32398,#32399),(#32400,#32401),(#32402,
#32403),(#32404,#32405),(#32406,#32407),(#32408,#32409),(#32410,#32411),
(#32412,#32413),(#32414,#32415),(#32416,#32417),(#32418,#32419),(#32420,
#32421),(#32422,#32423),(#32424,#32425),(#32426,#32427),(#32428,#32429),
(#32430,#32431),(#32432,#32433),(#32434,#32435),(#32436,#32437),(#32438,
#32439),(#32440,#32441),(#32442,#32443),(#32444,#32445)),.UNSPECIFIED.,
 .F.,.F.,.F.)
B_SPLINE_SURFACE_WITH_KNOTS((6,1,1,1,1,1,1,1,1,1,1,1,1,1,1,1,1,1,1,1,1,
1,1,1,1,1,1,1,1,1,1,1,1,1,1,1,1,1,1,1,1,1,1,1,1,1,1,1,1,1,1,1,1,1,1,1,1,
1,1,1,1,1,1,1,1,6),(2,2),(-1.,-0.984615384615383,-0.969230769230768,-0.953846153846152,
-0.938461538461537,-0.923076923076922,-0.907692307692306,-0.892307692307691,
-0.876923076923076,-0.86153846153846,-0.846153846153845,-0.83076923076923,
-0.815384615384614,-0.799999999999999,-0.784615384615384,-0.769230769230768,
-0.753846153846153,-0.738461538461538,-0.723076923076922,-0.707692307692307,
-0.692307692307692,-0.676923076923076,-0.661538461538461,-0.646153846153846,
-0.63076923076923,-0.615384615384615,-0.6,-0.584615384615384,-0.569230769230769,
-0.553846153846154,-0.538461538461538,-0.523076923076923,-0.507692307692308,
-0.492307692307692,-0.476923076923077,-0.461538461538462,-0.446153846153846,
-0.430769230769231,-0.415384615384615,-0.4,-0.384615384615385,-0.369230769230769,
-0.353846153846154,-0.338461538461538,-0.323076923076923,-0.307692307692308,
-0.292307692307692,-0.276923076923077,-0.261538461538462,-0.246153846153846,
-0.230769230769231,-0.215384615384615,-0.2,-0.184615384615385,-0.169230769230769,
-0.153846153846154,-0.138461538461538,-0.123076923076923,-0.107692307692308,
-0.0923076923076923,-0.0769230769230769,-0.0615384615384615,-0.0461538461538462,
-0.0307692307692308,-0.0153846153846154,0.),(-1.,1.),.UNSPECIFIED.)
GEOMETRIC_REPRESENTATION_ITEM()
RATIONAL_B_SPLINE_SURFACE(((1.,1.),(1.,1.),(1.,1.),(1.,1.),(1.,1.),(1.,
1.),(1.,1.),(1.,1.),(1.,1.),(1.,1.),(1.,1.),(1.,1.),(1.,1.),(1.,1.),(1.,
1.),(1.,1.),(1.,1.),(1.,1.),(1.,1.),(1.,1.),(1.,1.),(1.,1.),(1.,1.),(1.,
1.),(1.,1.),(1.,1.),(1.,1.),(1.,1.),(1.,1.),(1.,1.),(1.,1.),(1.,1.),(1.,
1.),(1.,1.),(1.,1.),(1.,1.),(1.,1.),(1.,1.),(1.,1.),(1.,1.),(1.,1.),(1.,
1.),(1.,1.),(1.,1.),(1.,1.),(1.,1.),(1.,1.),(1.,1.),(1.,1.),(1.,1.),(1.,
1.),(1.,1.),(1.,1.),(1.,1.),(1.,1.),(1.,1.),(1.,1.),(1.,1.),(1.,1.),(1.,
1.),(1.,1.),(1.,1.),(1.,1.),(1.,1.),(1.,1.),(1.,1.),(1.,1.),(1.,1.),(1.,
1.),(1.,1.)))
REPRESENTATION_ITEM('')
SURFACE()
);
#45=(
BOUNDED_SURFACE()
B_SPLINE_SURFACE(5,1,((#32522,#32523),(#32524,#32525),(#32526,#32527),(#32528,
#32529),(#32530,#32531),(#32532,#32533),(#32534,#32535),(#32536,#32537),
(#32538,#32539),(#32540,#32541),(#32542,#32543),(#32544,#32545),(#32546,
#32547),(#32548,#32549),(#32550,#32551),(#32552,#32553),(#32554,#32555),
(#32556,#32557),(#32558,#32559),(#32560,#32561),(#32562,#32563),(#32564,
#32565),(#32566,#32567),(#32568,#32569),(#32570,#32571),(#32572,#32573),
(#32574,#32575),(#32576,#32577),(#32578,#32579),(#32580,#32581),(#32582,
#32583),(#32584,#32585),(#32586,#32587),(#32588,#32589),(#32590,#32591),
(#32592,#32593),(#32594,#32595),(#32596,#32597),(#32598,#32599),(#32600,
#32601),(#32602,#32603),(#32604,#32605),(#32606,#32607),(#32608,#32609),
(#32610,#32611),(#32612,#32613),(#32614,#32615),(#32616,#32617),(#32618,
#32619),(#32620,#32621),(#32622,#32623),(#32624,#32625),(#32626,#32627),
(#32628,#32629),(#32630,#32631),(#32632,#32633),(#32634,#32635),(#32636,
#32637),(#32638,#32639),(#32640,#32641),(#32642,#32643),(#32644,#32645),
(#32646,#32647),(#32648,#32649),(#32650,#32651),(#32652,#32653),(#32654,
#32655),(#32656,#32657),(#32658,#32659),(#32660,#32661)),.UNSPECIFIED.,
 .F.,.F.,.F.)
B_SPLINE_SURFACE_WITH_KNOTS((6,1,1,1,1,1,1,1,1,1,1,1,1,1,1,1,1,1,1,1,1,
1,1,1,1,1,1,1,1,1,1,1,1,1,1,1,1,1,1,1,1,1,1,1,1,1,1,1,1,1,1,1,1,1,1,1,1,
1,1,1,1,1,1,1,1,6),(2,2),(-1.,-0.984615384615383,-0.969230769230768,-0.953846153846152,
-0.938461538461537,-0.923076923076922,-0.907692307692306,-0.892307692307691,
-0.876923076923076,-0.86153846153846,-0.846153846153845,-0.83076923076923,
-0.815384615384614,-0.799999999999999,-0.784615384615384,-0.769230769230768,
-0.753846153846153,-0.738461538461538,-0.723076923076922,-0.707692307692307,
-0.692307692307692,-0.676923076923076,-0.661538461538461,-0.646153846153846,
-0.63076923076923,-0.615384615384615,-0.6,-0.584615384615384,-0.569230769230769,
-0.553846153846154,-0.538461538461538,-0.523076923076923,-0.507692307692308,
-0.492307692307692,-0.476923076923077,-0.461538461538462,-0.446153846153846,
-0.430769230769231,-0.415384615384615,-0.4,-0.384615384615385,-0.369230769230769,
-0.353846153846154,-0.338461538461538,-0.323076923076923,-0.307692307692308,
-0.292307692307692,-0.276923076923077,-0.261538461538462,-0.246153846153846,
-0.230769230769231,-0.215384615384615,-0.2,-0.184615384615385,-0.169230769230769,
-0.153846153846154,-0.138461538461538,-0.123076923076923,-0.107692307692308,
-0.0923076923076923,-0.0769230769230769,-0.0615384615384615,-0.0461538461538462,
-0.0307692307692308,-0.0153846153846154,0.),(-1.,1.),.UNSPECIFIED.)
GEOMETRIC_REPRESENTATION_ITEM()
RATIONAL_B_SPLINE_SURFACE(((1.,1.),(1.,1.),(1.,1.),(1.,1.),(1.,1.),(1.,
1.),(1.,1.),(1.,1.),(1.,1.),(1.,1.),(1.,1.),(1.,1.),(1.,1.),(1.,1.),(1.,
1.),(1.,1.),(1.,1.),(1.,1.),(1.,1.),(1.,1.),(1.,1.),(1.,1.),(1.,1.),(1.,
1.),(1.,1.),(1.,1.),(1.,1.),(1.,1.),(1.,1.),(1.,1.),(1.,1.),(1.,1.),(1.,
1.),(1.,1.),(1.,1.),(1.,1.),(1.,1.),(1.,1.),(1.,1.),(1.,1.),(1.,1.),(1.,
1.),(1.,1.),(1.,1.),(1.,1.),(1.,1.),(1.,1.),(1.,1.),(1.,1.),(1.,1.),(1.,
1.),(1.,1.),(1.,1.),(1.,1.),(1.,1.),(1.,1.),(1.,1.),(1.,1.),(1.,1.),(1.,
1.),(1.,1.),(1.,1.),(1.,1.),(1.,1.),(1.,1.),(1.,1.),(1.,1.),(1.,1.),(1.,
1.),(1.,1.)))
REPRESENTATION_ITEM('')
SURFACE()
);
#46=(
BOUNDED_SURFACE()
B_SPLINE_SURFACE(5,1,((#32738,#32739),(#32740,#32741),(#32742,#32743),(#32744,
#32745),(#32746,#32747),(#32748,#32749),(#32750,#32751),(#32752,#32753),
(#32754,#32755),(#32756,#32757),(#32758,#32759),(#32760,#32761),(#32762,
#32763),(#32764,#32765),(#32766,#32767),(#32768,#32769),(#32770,#32771),
(#32772,#32773),(#32774,#32775),(#32776,#32777),(#32778,#32779),(#32780,
#32781),(#32782,#32783),(#32784,#32785),(#32786,#32787),(#32788,#32789),
(#32790,#32791),(#32792,#32793),(#32794,#32795),(#32796,#32797),(#32798,
#32799),(#32800,#32801),(#32802,#32803),(#32804,#32805),(#32806,#32807),
(#32808,#32809),(#32810,#32811),(#32812,#32813),(#32814,#32815),(#32816,
#32817),(#32818,#32819),(#32820,#32821),(#32822,#32823),(#32824,#32825),
(#32826,#32827),(#32828,#32829),(#32830,#32831),(#32832,#32833),(#32834,
#32835),(#32836,#32837),(#32838,#32839),(#32840,#32841),(#32842,#32843),
(#32844,#32845),(#32846,#32847),(#32848,#32849),(#32850,#32851),(#32852,
#32853),(#32854,#32855),(#32856,#32857),(#32858,#32859),(#32860,#32861),
(#32862,#32863),(#32864,#32865),(#32866,#32867),(#32868,#32869),(#32870,
#32871),(#32872,#32873),(#32874,#32875),(#32876,#32877)),.UNSPECIFIED.,
 .F.,.F.,.F.)
B_SPLINE_SURFACE_WITH_KNOTS((6,1,1,1,1,1,1,1,1,1,1,1,1,1,1,1,1,1,1,1,1,
1,1,1,1,1,1,1,1,1,1,1,1,1,1,1,1,1,1,1,1,1,1,1,1,1,1,1,1,1,1,1,1,1,1,1,1,
1,1,1,1,1,1,1,1,6),(2,2),(-1.,-0.984615384615383,-0.969230769230768,-0.953846153846152,
-0.938461538461537,-0.923076923076922,-0.907692307692306,-0.892307692307691,
-0.876923076923076,-0.86153846153846,-0.846153846153845,-0.83076923076923,
-0.815384615384614,-0.799999999999999,-0.784615384615384,-0.769230769230768,
-0.753846153846153,-0.738461538461538,-0.723076923076922,-0.707692307692307,
-0.692307692307692,-0.676923076923076,-0.661538461538461,-0.646153846153846,
-0.63076923076923,-0.615384615384615,-0.6,-0.584615384615384,-0.569230769230769,
-0.553846153846154,-0.538461538461538,-0.523076923076923,-0.507692307692308,
-0.492307692307692,-0.476923076923077,-0.461538461538462,-0.446153846153846,
-0.430769230769231,-0.415384615384615,-0.4,-0.384615384615385,-0.369230769230769,
-0.353846153846154,-0.338461538461538,-0.323076923076923,-0.307692307692308,
-0.292307692307692,-0.276923076923077,-0.261538461538462,-0.246153846153846,
-0.230769230769231,-0.215384615384615,-0.2,-0.184615384615385,-0.169230769230769,
-0.153846153846154,-0.138461538461538,-0.123076923076923,-0.107692307692308,
-0.0923076923076923,-0.0769230769230769,-0.0615384615384615,-0.0461538461538462,
-0.0307692307692308,-0.0153846153846154,0.),(-1.,1.),.UNSPECIFIED.)
GEOMETRIC_REPRESENTATION_ITEM()
RATIONAL_B_SPLINE_SURFACE(((1.,1.),(1.,1.),(1.,1.),(1.,1.),(1.,1.),(1.,
1.),(1.,1.),(1.,1.),(1.,1.),(1.,1.),(1.,1.),(1.,1.),(1.,1.),(1.,1.),(1.,
1.),(1.,1.),(1.,1.),(1.,1.),(1.,1.),(1.,1.),(1.,1.),(1.,1.),(1.,1.),(1.,
1.),(1.,1.),(1.,1.),(1.,1.),(1.,1.),(1.,1.),(1.,1.),(1.,1.),(1.,1.),(1.,
1.),(1.,1.),(1.,1.),(1.,1.),(1.,1.),(1.,1.),(1.,1.),(1.,1.),(1.,1.),(1.,
1.),(1.,1.),(1.,1.),(1.,1.),(1.,1.),(1.,1.),(1.,1.),(1.,1.),(1.,1.),(1.,
1.),(1.,1.),(1.,1.),(1.,1.),(1.,1.),(1.,1.),(1.,1.),(1.,1.),(1.,1.),(1.,
1.),(1.,1.),(1.,1.),(1.,1.),(1.,1.),(1.,1.),(1.,1.),(1.,1.),(1.,1.),(1.,
1.),(1.,1.)))
REPRESENTATION_ITEM('')
SURFACE()
);
#47=(
BOUNDED_SURFACE()
B_SPLINE_SURFACE(5,1,((#32954,#32955),(#32956,#32957),(#32958,#32959),(#32960,
#32961),(#32962,#32963),(#32964,#32965),(#32966,#32967),(#32968,#32969),
(#32970,#32971),(#32972,#32973),(#32974,#32975),(#32976,#32977),(#32978,
#32979),(#32980,#32981),(#32982,#32983),(#32984,#32985),(#32986,#32987),
(#32988,#32989),(#32990,#32991),(#32992,#32993),(#32994,#32995),(#32996,
#32997),(#32998,#32999),(#33000,#33001),(#33002,#33003),(#33004,#33005),
(#33006,#33007),(#33008,#33009),(#33010,#33011),(#33012,#33013),(#33014,
#33015),(#33016,#33017),(#33018,#33019),(#33020,#33021),(#33022,#33023),
(#33024,#33025),(#33026,#33027),(#33028,#33029),(#33030,#33031),(#33032,
#33033),(#33034,#33035),(#33036,#33037),(#33038,#33039),(#33040,#33041),
(#33042,#33043),(#33044,#33045),(#33046,#33047),(#33048,#33049),(#33050,
#33051),(#33052,#33053),(#33054,#33055),(#33056,#33057),(#33058,#33059),
(#33060,#33061),(#33062,#33063),(#33064,#33065),(#33066,#33067),(#33068,
#33069),(#33070,#33071),(#33072,#33073),(#33074,#33075),(#33076,#33077),
(#33078,#33079),(#33080,#33081),(#33082,#33083),(#33084,#33085),(#33086,
#33087),(#33088,#33089),(#33090,#33091),(#33092,#33093)),.UNSPECIFIED.,
 .F.,.F.,.F.)
B_SPLINE_SURFACE_WITH_KNOTS((6,1,1,1,1,1,1,1,1,1,1,1,1,1,1,1,1,1,1,1,1,
1,1,1,1,1,1,1,1,1,1,1,1,1,1,1,1,1,1,1,1,1,1,1,1,1,1,1,1,1,1,1,1,1,1,1,1,
1,1,1,1,1,1,1,1,6),(2,2),(-1.,-0.984615384615383,-0.969230769230768,-0.953846153846152,
-0.938461538461537,-0.923076923076922,-0.907692307692306,-0.892307692307691,
-0.876923076923076,-0.86153846153846,-0.846153846153845,-0.83076923076923,
-0.815384615384614,-0.799999999999999,-0.784615384615384,-0.769230769230768,
-0.753846153846153,-0.738461538461538,-0.723076923076922,-0.707692307692307,
-0.692307692307692,-0.676923076923076,-0.661538461538461,-0.646153846153846,
-0.63076923076923,-0.615384615384615,-0.6,-0.584615384615384,-0.569230769230769,
-0.553846153846154,-0.538461538461538,-0.523076923076923,-0.507692307692308,
-0.492307692307692,-0.476923076923077,-0.461538461538462,-0.446153846153846,
-0.430769230769231,-0.415384615384615,-0.4,-0.384615384615385,-0.369230769230769,
-0.353846153846154,-0.338461538461538,-0.323076923076923,-0.307692307692308,
-0.292307692307692,-0.276923076923077,-0.261538461538462,-0.246153846153846,
-0.230769230769231,-0.215384615384615,-0.2,-0.184615384615385,-0.169230769230769,
-0.153846153846154,-0.138461538461538,-0.123076923076923,-0.107692307692308,
-0.0923076923076923,-0.0769230769230769,-0.0615384615384615,-0.0461538461538462,
-0.0307692307692308,-0.0153846153846154,0.),(-1.,1.),.UNSPECIFIED.)
GEOMETRIC_REPRESENTATION_ITEM()
RATIONAL_B_SPLINE_SURFACE(((1.,1.),(1.,1.),(1.,1.),(1.,1.),(1.,1.),(1.,
1.),(1.,1.),(1.,1.),(1.,1.),(1.,1.),(1.,1.),(1.,1.),(1.,1.),(1.,1.),(1.,
1.),(1.,1.),(1.,1.),(1.,1.),(1.,1.),(1.,1.),(1.,1.),(1.,1.),(1.,1.),(1.,
1.),(1.,1.),(1.,1.),(1.,1.),(1.,1.),(1.,1.),(1.,1.),(1.,1.),(1.,1.),(1.,
1.),(1.,1.),(1.,1.),(1.,1.),(1.,1.),(1.,1.),(1.,1.),(1.,1.),(1.,1.),(1.,
1.),(1.,1.),(1.,1.),(1.,1.),(1.,1.),(1.,1.),(1.,1.),(1.,1.),(1.,1.),(1.,
1.),(1.,1.),(1.,1.),(1.,1.),(1.,1.),(1.,1.),(1.,1.),(1.,1.),(1.,1.),(1.,
1.),(1.,1.),(1.,1.),(1.,1.),(1.,1.),(1.,1.),(1.,1.),(1.,1.),(1.,1.),(1.,
1.),(1.,1.)))
REPRESENTATION_ITEM('')
SURFACE()
);
#48=(
BOUNDED_SURFACE()
B_SPLINE_SURFACE(5,1,((#33170,#33171),(#33172,#33173),(#33174,#33175),(#33176,
#33177),(#33178,#33179),(#33180,#33181),(#33182,#33183),(#33184,#33185),
(#33186,#33187),(#33188,#33189),(#33190,#33191),(#33192,#33193),(#33194,
#33195),(#33196,#33197),(#33198,#33199),(#33200,#33201),(#33202,#33203),
(#33204,#33205),(#33206,#33207),(#33208,#33209),(#33210,#33211),(#33212,
#33213),(#33214,#33215),(#33216,#33217),(#33218,#33219),(#33220,#33221),
(#33222,#33223),(#33224,#33225),(#33226,#33227),(#33228,#33229),(#33230,
#33231),(#33232,#33233),(#33234,#33235),(#33236,#33237),(#33238,#33239),
(#33240,#33241),(#33242,#33243),(#33244,#33245),(#33246,#33247),(#33248,
#33249),(#33250,#33251),(#33252,#33253),(#33254,#33255),(#33256,#33257),
(#33258,#33259),(#33260,#33261),(#33262,#33263),(#33264,#33265),(#33266,
#33267),(#33268,#33269),(#33270,#33271),(#33272,#33273),(#33274,#33275),
(#33276,#33277),(#33278,#33279),(#33280,#33281),(#33282,#33283),(#33284,
#33285),(#33286,#33287),(#33288,#33289),(#33290,#33291),(#33292,#33293),
(#33294,#33295),(#33296,#33297),(#33298,#33299),(#33300,#33301),(#33302,
#33303),(#33304,#33305),(#33306,#33307),(#33308,#33309)),.UNSPECIFIED.,
 .F.,.F.,.F.)
B_SPLINE_SURFACE_WITH_KNOTS((6,1,1,1,1,1,1,1,1,1,1,1,1,1,1,1,1,1,1,1,1,
1,1,1,1,1,1,1,1,1,1,1,1,1,1,1,1,1,1,1,1,1,1,1,1,1,1,1,1,1,1,1,1,1,1,1,1,
1,1,1,1,1,1,1,1,6),(2,2),(-1.,-0.984615384615383,-0.969230769230768,-0.953846153846152,
-0.938461538461537,-0.923076923076922,-0.907692307692306,-0.892307692307691,
-0.876923076923076,-0.86153846153846,-0.846153846153845,-0.83076923076923,
-0.815384615384614,-0.799999999999999,-0.784615384615384,-0.769230769230768,
-0.753846153846153,-0.738461538461538,-0.723076923076922,-0.707692307692307,
-0.692307692307692,-0.676923076923076,-0.661538461538461,-0.646153846153846,
-0.63076923076923,-0.615384615384615,-0.6,-0.584615384615384,-0.569230769230769,
-0.553846153846154,-0.538461538461538,-0.523076923076923,-0.507692307692308,
-0.492307692307692,-0.476923076923077,-0.461538461538462,-0.446153846153846,
-0.430769230769231,-0.415384615384615,-0.4,-0.384615384615385,-0.369230769230769,
-0.353846153846154,-0.338461538461538,-0.323076923076923,-0.307692307692308,
-0.292307692307692,-0.276923076923077,-0.261538461538462,-0.246153846153846,
-0.230769230769231,-0.215384615384615,-0.2,-0.184615384615385,-0.169230769230769,
-0.153846153846154,-0.138461538461538,-0.123076923076923,-0.107692307692308,
-0.0923076923076923,-0.0769230769230769,-0.0615384615384615,-0.0461538461538462,
-0.0307692307692308,-0.0153846153846154,0.),(-1.,1.),.UNSPECIFIED.)
GEOMETRIC_REPRESENTATION_ITEM()
RATIONAL_B_SPLINE_SURFACE(((1.,1.),(1.,1.),(1.,1.),(1.,1.),(1.,1.),(1.,
1.),(1.,1.),(1.,1.),(1.,1.),(1.,1.),(1.,1.),(1.,1.),(1.,1.),(1.,1.),(1.,
1.),(1.,1.),(1.,1.),(1.,1.),(1.,1.),(1.,1.),(1.,1.),(1.,1.),(1.,1.),(1.,
1.),(1.,1.),(1.,1.),(1.,1.),(1.,1.),(1.,1.),(1.,1.),(1.,1.),(1.,1.),(1.,
1.),(1.,1.),(1.,1.),(1.,1.),(1.,1.),(1.,1.),(1.,1.),(1.,1.),(1.,1.),(1.,
1.),(1.,1.),(1.,1.),(1.,1.),(1.,1.),(1.,1.),(1.,1.),(1.,1.),(1.,1.),(1.,
1.),(1.,1.),(1.,1.),(1.,1.),(1.,1.),(1.,1.),(1.,1.),(1.,1.),(1.,1.),(1.,
1.),(1.,1.),(1.,1.),(1.,1.),(1.,1.),(1.,1.),(1.,1.),(1.,1.),(1.,1.),(1.,
1.),(1.,1.)))
REPRESENTATION_ITEM('')
SURFACE()
);
#49=(
BOUNDED_SURFACE()
B_SPLINE_SURFACE(5,1,((#33386,#33387),(#33388,#33389),(#33390,#33391),(#33392,
#33393),(#33394,#33395),(#33396,#33397),(#33398,#33399),(#33400,#33401),
(#33402,#33403),(#33404,#33405),(#33406,#33407),(#33408,#33409),(#33410,
#33411),(#33412,#33413),(#33414,#33415),(#33416,#33417),(#33418,#33419),
(#33420,#33421),(#33422,#33423),(#33424,#33425),(#33426,#33427),(#33428,
#33429),(#33430,#33431),(#33432,#33433),(#33434,#33435),(#33436,#33437),
(#33438,#33439),(#33440,#33441),(#33442,#33443),(#33444,#33445),(#33446,
#33447),(#33448,#33449),(#33450,#33451),(#33452,#33453),(#33454,#33455),
(#33456,#33457),(#33458,#33459),(#33460,#33461),(#33462,#33463),(#33464,
#33465),(#33466,#33467),(#33468,#33469),(#33470,#33471),(#33472,#33473),
(#33474,#33475),(#33476,#33477),(#33478,#33479),(#33480,#33481),(#33482,
#33483),(#33484,#33485),(#33486,#33487),(#33488,#33489),(#33490,#33491),
(#33492,#33493),(#33494,#33495),(#33496,#33497),(#33498,#33499),(#33500,
#33501),(#33502,#33503),(#33504,#33505),(#33506,#33507),(#33508,#33509),
(#33510,#33511),(#33512,#33513),(#33514,#33515),(#33516,#33517),(#33518,
#33519),(#33520,#33521),(#33522,#33523),(#33524,#33525)),.UNSPECIFIED.,
 .F.,.F.,.F.)
B_SPLINE_SURFACE_WITH_KNOTS((6,1,1,1,1,1,1,1,1,1,1,1,1,1,1,1,1,1,1,1,1,
1,1,1,1,1,1,1,1,1,1,1,1,1,1,1,1,1,1,1,1,1,1,1,1,1,1,1,1,1,1,1,1,1,1,1,1,
1,1,1,1,1,1,1,1,6),(2,2),(-1.,-0.984615384615383,-0.969230769230768,-0.953846153846152,
-0.938461538461537,-0.923076923076922,-0.907692307692306,-0.892307692307691,
-0.876923076923076,-0.86153846153846,-0.846153846153845,-0.83076923076923,
-0.815384615384614,-0.799999999999999,-0.784615384615384,-0.769230769230768,
-0.753846153846153,-0.738461538461538,-0.723076923076922,-0.707692307692307,
-0.692307692307692,-0.676923076923076,-0.661538461538461,-0.646153846153846,
-0.63076923076923,-0.615384615384615,-0.6,-0.584615384615384,-0.569230769230769,
-0.553846153846154,-0.538461538461538,-0.523076923076923,-0.507692307692308,
-0.492307692307692,-0.476923076923077,-0.461538461538462,-0.446153846153846,
-0.430769230769231,-0.415384615384615,-0.4,-0.384615384615385,-0.369230769230769,
-0.353846153846154,-0.338461538461538,-0.323076923076923,-0.307692307692308,
-0.292307692307692,-0.276923076923077,-0.261538461538462,-0.246153846153846,
-0.230769230769231,-0.215384615384615,-0.2,-0.184615384615385,-0.169230769230769,
-0.153846153846154,-0.138461538461538,-0.123076923076923,-0.107692307692308,
-0.0923076923076923,-0.0769230769230769,-0.0615384615384615,-0.0461538461538462,
-0.0307692307692308,-0.0153846153846154,0.),(-1.,1.),.UNSPECIFIED.)
GEOMETRIC_REPRESENTATION_ITEM()
RATIONAL_B_SPLINE_SURFACE(((1.,1.),(1.,1.),(1.,1.),(1.,1.),(1.,1.),(1.,
1.),(1.,1.),(1.,1.),(1.,1.),(1.,1.),(1.,1.),(1.,1.),(1.,1.),(1.,1.),(1.,
1.),(1.,1.),(1.,1.),(1.,1.),(1.,1.),(1.,1.),(1.,1.),(1.,1.),(1.,1.),(1.,
1.),(1.,1.),(1.,1.),(1.,1.),(1.,1.),(1.,1.),(1.,1.),(1.,1.),(1.,1.),(1.,
1.),(1.,1.),(1.,1.),(1.,1.),(1.,1.),(1.,1.),(1.,1.),(1.,1.),(1.,1.),(1.,
1.),(1.,1.),(1.,1.),(1.,1.),(1.,1.),(1.,1.),(1.,1.),(1.,1.),(1.,1.),(1.,
1.),(1.,1.),(1.,1.),(1.,1.),(1.,1.),(1.,1.),(1.,1.),(1.,1.),(1.,1.),(1.,
1.),(1.,1.),(1.,1.),(1.,1.),(1.,1.),(1.,1.),(1.,1.),(1.,1.),(1.,1.),(1.,
1.),(1.,1.)))
REPRESENTATION_ITEM('')
SURFACE()
);
#50=(
BOUNDED_SURFACE()
B_SPLINE_SURFACE(5,1,((#33602,#33603),(#33604,#33605),(#33606,#33607),(#33608,
#33609),(#33610,#33611),(#33612,#33613),(#33614,#33615),(#33616,#33617),
(#33618,#33619),(#33620,#33621),(#33622,#33623),(#33624,#33625),(#33626,
#33627),(#33628,#33629),(#33630,#33631),(#33632,#33633),(#33634,#33635),
(#33636,#33637),(#33638,#33639),(#33640,#33641),(#33642,#33643),(#33644,
#33645),(#33646,#33647),(#33648,#33649),(#33650,#33651),(#33652,#33653),
(#33654,#33655),(#33656,#33657),(#33658,#33659),(#33660,#33661),(#33662,
#33663),(#33664,#33665),(#33666,#33667),(#33668,#33669),(#33670,#33671),
(#33672,#33673),(#33674,#33675),(#33676,#33677),(#33678,#33679),(#33680,
#33681),(#33682,#33683),(#33684,#33685),(#33686,#33687),(#33688,#33689),
(#33690,#33691),(#33692,#33693),(#33694,#33695),(#33696,#33697),(#33698,
#33699),(#33700,#33701),(#33702,#33703),(#33704,#33705),(#33706,#33707),
(#33708,#33709),(#33710,#33711),(#33712,#33713),(#33714,#33715),(#33716,
#33717),(#33718,#33719),(#33720,#33721),(#33722,#33723),(#33724,#33725),
(#33726,#33727),(#33728,#33729),(#33730,#33731),(#33732,#33733),(#33734,
#33735),(#33736,#33737),(#33738,#33739),(#33740,#33741)),.UNSPECIFIED.,
 .F.,.F.,.F.)
B_SPLINE_SURFACE_WITH_KNOTS((6,1,1,1,1,1,1,1,1,1,1,1,1,1,1,1,1,1,1,1,1,
1,1,1,1,1,1,1,1,1,1,1,1,1,1,1,1,1,1,1,1,1,1,1,1,1,1,1,1,1,1,1,1,1,1,1,1,
1,1,1,1,1,1,1,1,6),(2,2),(-1.,-0.984615384615383,-0.969230769230768,-0.953846153846152,
-0.938461538461537,-0.923076923076922,-0.907692307692306,-0.892307692307691,
-0.876923076923076,-0.86153846153846,-0.846153846153845,-0.83076923076923,
-0.815384615384614,-0.799999999999999,-0.784615384615384,-0.769230769230768,
-0.753846153846153,-0.738461538461538,-0.723076923076922,-0.707692307692307,
-0.692307692307692,-0.676923076923076,-0.661538461538461,-0.646153846153846,
-0.63076923076923,-0.615384615384615,-0.6,-0.584615384615384,-0.569230769230769,
-0.553846153846154,-0.538461538461538,-0.523076923076923,-0.507692307692308,
-0.492307692307692,-0.476923076923077,-0.461538461538462,-0.446153846153846,
-0.430769230769231,-0.415384615384615,-0.4,-0.384615384615385,-0.369230769230769,
-0.353846153846154,-0.338461538461538,-0.323076923076923,-0.307692307692308,
-0.292307692307692,-0.276923076923077,-0.261538461538462,-0.246153846153846,
-0.230769230769231,-0.215384615384615,-0.2,-0.184615384615385,-0.169230769230769,
-0.153846153846154,-0.138461538461538,-0.123076923076923,-0.107692307692308,
-0.0923076923076923,-0.0769230769230769,-0.0615384615384615,-0.0461538461538462,
-0.0307692307692308,-0.0153846153846154,0.),(-1.,1.),.UNSPECIFIED.)
GEOMETRIC_REPRESENTATION_ITEM()
RATIONAL_B_SPLINE_SURFACE(((1.,1.),(1.,1.),(1.,1.),(1.,1.),(1.,1.),(1.,
1.),(1.,1.),(1.,1.),(1.,1.),(1.,1.),(1.,1.),(1.,1.),(1.,1.),(1.,1.),(1.,
1.),(1.,1.),(1.,1.),(1.,1.),(1.,1.),(1.,1.),(1.,1.),(1.,1.),(1.,1.),(1.,
1.),(1.,1.),(1.,1.),(1.,1.),(1.,1.),(1.,1.),(1.,1.),(1.,1.),(1.,1.),(1.,
1.),(1.,1.),(1.,1.),(1.,1.),(1.,1.),(1.,1.),(1.,1.),(1.,1.),(1.,1.),(1.,
1.),(1.,1.),(1.,1.),(1.,1.),(1.,1.),(1.,1.),(1.,1.),(1.,1.),(1.,1.),(1.,
1.),(1.,1.),(1.,1.),(1.,1.),(1.,1.),(1.,1.),(1.,1.),(1.,1.),(1.,1.),(1.,
1.),(1.,1.),(1.,1.),(1.,1.),(1.,1.),(1.,1.),(1.,1.),(1.,1.),(1.,1.),(1.,
1.),(1.,1.)))
REPRESENTATION_ITEM('')
SURFACE()
);
#131=(
BOUNDED_CURVE()
B_SPLINE_CURVE(5,(#22250,#22251,#22252,#22253,#22254,#22255,#22256,#22257,
#22258,#22259,#22260,#22261,#22262,#22263,#22264,#22265,#22266,#22267,#22268,
#22269,#22270,#22271,#22272,#22273,#22274,#22275,#22276,#22277,#22278,#22279,
#22280,#22281,#22282,#22283,#22284,#22285,#22286,#22287,#22288,#22289,#22290,
#22291,#22292,#22293,#22294,#22295,#22296,#22297,#22298,#22299,#22300,#22301,
#22302,#22303,#22304,#22305,#22306,#22307,#22308,#22309,#22310,#22311,#22312,
#22313,#22314,#22315,#22316,#22317,#22318,#22319),.UNSPECIFIED.,.F.,.F.)
B_SPLINE_CURVE_WITH_KNOTS((6,1,1,1,1,1,1,1,1,1,1,1,1,1,1,1,1,1,1,1,1,1,
1,1,1,1,1,1,1,1,1,1,1,1,1,1,1,1,1,1,1,1,1,1,1,1,1,1,1,1,1,1,1,1,1,1,1,1,
1,1,1,1,1,1,1,6),(0.,0.0153846153846154,0.0307692307692308,0.0461538461538462,
0.0615384615384615,0.0769230769230769,0.0923076923076923,0.107692307692308,
0.123076923076923,0.138461538461538,0.153846153846154,0.169230769230769,
0.184615384615385,0.2,0.215384615384615,0.230769230769231,0.246153846153846,
0.261538461538462,0.276923076923077,0.292307692307692,0.307692307692308,
0.323076923076923,0.338461538461538,0.353846153846154,0.369230769230769,
0.384615384615385,0.4,0.415384615384615,0.430769230769231,0.446153846153846,
0.461538461538462,0.476923076923077,0.492307692307692,0.507692307692308,
0.523076923076923,0.538461538461538,0.553846153846154,0.569230769230769,
0.584615384615384,0.6,0.615384615384615,0.63076923076923,0.646153846153846,
0.661538461538461,0.676923076923076,0.692307692307692,0.707692307692307,
0.723076923076922,0.738461538461538,0.753846153846153,0.769230769230768,
0.784615384615384,0.799999999999999,0.815384615384614,0.83076923076923,
0.846153846153845,0.86153846153846,0.876923076923076,0.892307692307691,
0.907692307692306,0.923076923076922,0.938461538461537,0.953846153846152,
0.969230769230768,0.984615384615383,1.),.UNSPECIFIED.)
CURVE()
GEOMETRIC_REPRESENTATION_ITEM()
RATIONAL_B_SPLINE_CURVE((1.,1.,1.,1.,1.,1.,1.,1.,1.,1.,1.,1.,1.,1.,1.,1.,
1.,1.,1.,1.,1.,1.,1.,1.,1.,1.,1.,1.,1.,1.,1.,1.,1.,1.,1.,1.,1.,1.,1.,1.,
1.,1.,1.,1.,1.,1.,1.,1.,1.,1.,1.,1.,1.,1.,1.,1.,1.,1.,1.,1.,1.,1.,1.,1.,
1.,1.,1.,1.,1.,1.))
REPRESENTATION_ITEM('')
);
#132=(
BOUNDED_CURVE()
B_SPLINE_CURVE(5,(#22323,#22324,#22325,#22326,#22327,#22328,#22329,#22330,
#22331,#22332,#22333,#22334,#22335,#22336,#22337,#22338,#22339,#22340,#22341,
#22342,#22343,#22344,#22345,#22346,#22347,#22348,#22349,#22350,#22351,#22352,
#22353,#22354,#22355,#22356,#22357,#22358,#22359,#22360,#22361,#22362,#22363,
#22364,#22365,#22366,#22367,#22368,#22369,#22370,#22371,#22372,#22373,#22374,
#22375,#22376,#22377,#22378,#22379,#22380,#22381,#22382,#22383,#22384,#22385,
#22386,#22387,#22388,#22389,#22390,#22391,#22392),.UNSPECIFIED.,.F.,.F.)
B_SPLINE_CURVE_WITH_KNOTS((6,1,1,1,1,1,1,1,1,1,1,1,1,1,1,1,1,1,1,1,1,1,
1,1,1,1,1,1,1,1,1,1,1,1,1,1,1,1,1,1,1,1,1,1,1,1,1,1,1,1,1,1,1,1,1,1,1,1,
1,1,1,1,1,1,1,6),(0.,0.0153846153846154,0.0307692307692308,0.0461538461538462,
0.0615384615384615,0.0769230769230769,0.0923076923076923,0.107692307692308,
0.123076923076923,0.138461538461538,0.153846153846154,0.169230769230769,
0.184615384615385,0.2,0.215384615384615,0.230769230769231,0.246153846153846,
0.261538461538462,0.276923076923077,0.292307692307692,0.307692307692308,
0.323076923076923,0.338461538461538,0.353846153846154,0.369230769230769,
0.384615384615385,0.4,0.415384615384615,0.430769230769231,0.446153846153846,
0.461538461538462,0.476923076923077,0.492307692307692,0.507692307692308,
0.523076923076923,0.538461538461538,0.553846153846154,0.569230769230769,
0.584615384615384,0.6,0.615384615384615,0.63076923076923,0.646153846153846,
0.661538461538461,0.676923076923076,0.692307692307692,0.707692307692307,
0.723076923076922,0.738461538461538,0.753846153846153,0.769230769230768,
0.784615384615384,0.799999999999999,0.815384615384614,0.83076923076923,
0.846153846153845,0.86153846153846,0.876923076923076,0.892307692307691,
0.907692307692306,0.923076923076922,0.938461538461537,0.953846153846152,
0.969230769230768,0.984615384615383,1.),.UNSPECIFIED.)
CURVE()
GEOMETRIC_REPRESENTATION_ITEM()
RATIONAL_B_SPLINE_CURVE((1.,1.,1.,1.,1.,1.,1.,1.,1.,1.,1.,1.,1.,1.,1.,1.,
1.,1.,1.,1.,1.,1.,1.,1.,1.,1.,1.,1.,1.,1.,1.,1.,1.,1.,1.,1.,1.,1.,1.,1.,
1.,1.,1.,1.,1.,1.,1.,1.,1.,1.,1.,1.,1.,1.,1.,1.,1.,1.,1.,1.,1.,1.,1.,1.,
1.,1.,1.,1.,1.,1.))
REPRESENTATION_ITEM('')
);
#133=(
BOUNDED_CURVE()
B_SPLINE_CURVE(5,(#22396,#22397,#22398,#22399,#22400,#22401,#22402,#22403,
#22404,#22405,#22406,#22407,#22408,#22409,#22410,#22411,#22412,#22413,#22414,
#22415,#22416,#22417,#22418,#22419,#22420,#22421,#22422,#22423,#22424,#22425,
#22426,#22427,#22428,#22429,#22430,#22431,#22432,#22433,#22434,#22435,#22436,
#22437,#22438,#22439,#22440,#22441,#22442,#22443,#22444,#22445,#22446,#22447,
#22448,#22449,#22450,#22451,#22452,#22453,#22454,#22455,#22456,#22457,#22458,
#22459,#22460,#22461,#22462,#22463,#22464,#22465),.UNSPECIFIED.,.F.,.F.)
B_SPLINE_CURVE_WITH_KNOTS((6,1,1,1,1,1,1,1,1,1,1,1,1,1,1,1,1,1,1,1,1,1,
1,1,1,1,1,1,1,1,1,1,1,1,1,1,1,1,1,1,1,1,1,1,1,1,1,1,1,1,1,1,1,1,1,1,1,1,
1,1,1,1,1,1,1,6),(0.,0.0153846153846154,0.0307692307692308,0.0461538461538462,
0.0615384615384615,0.0769230769230769,0.0923076923076923,0.107692307692308,
0.123076923076923,0.138461538461538,0.153846153846154,0.169230769230769,
0.184615384615385,0.2,0.215384615384615,0.230769230769231,0.246153846153846,
0.261538461538462,0.276923076923077,0.292307692307692,0.307692307692308,
0.323076923076923,0.338461538461538,0.353846153846154,0.369230769230769,
0.384615384615385,0.4,0.415384615384615,0.430769230769231,0.446153846153846,
0.461538461538462,0.476923076923077,0.492307692307692,0.507692307692308,
0.523076923076923,0.538461538461538,0.553846153846154,0.569230769230769,
0.584615384615384,0.6,0.615384615384615,0.63076923076923,0.646153846153846,
0.661538461538461,0.676923076923076,0.692307692307692,0.707692307692307,
0.723076923076922,0.738461538461538,0.753846153846153,0.769230769230768,
0.784615384615384,0.799999999999999,0.815384615384614,0.83076923076923,
0.846153846153845,0.86153846153846,0.876923076923076,0.892307692307691,
0.907692307692306,0.923076923076922,0.938461538461537,0.953846153846152,
0.969230769230768,0.984615384615383,1.),.UNSPECIFIED.)
CURVE()
GEOMETRIC_REPRESENTATION_ITEM()
RATIONAL_B_SPLINE_CURVE((1.,1.,1.,1.,1.,1.,1.,1.,1.,1.,1.,1.,1.,1.,1.,1.,
1.,1.,1.,1.,1.,1.,1.,1.,1.,1.,1.,1.,1.,1.,1.,1.,1.,1.,1.,1.,1.,1.,1.,1.,
1.,1.,1.,1.,1.,1.,1.,1.,1.,1.,1.,1.,1.,1.,1.,1.,1.,1.,1.,1.,1.,1.,1.,1.,
1.,1.,1.,1.,1.,1.))
REPRESENTATION_ITEM('')
);
#134=(
BOUNDED_CURVE()
B_SPLINE_CURVE(5,(#22469,#22470,#22471,#22472,#22473,#22474,#22475,#22476,
#22477,#22478,#22479,#22480,#22481,#22482,#22483,#22484,#22485,#22486,#22487,
#22488,#22489,#22490,#22491,#22492,#22493,#22494,#22495,#22496,#22497,#22498,
#22499,#22500,#22501,#22502,#22503,#22504,#22505,#22506,#22507,#22508,#22509,
#22510,#22511,#22512,#22513,#22514,#22515,#22516,#22517,#22518,#22519,#22520,
#22521,#22522,#22523,#22524,#22525,#22526,#22527,#22528,#22529,#22530,#22531,
#22532,#22533,#22534,#22535,#22536,#22537,#22538),.UNSPECIFIED.,.F.,.F.)
B_SPLINE_CURVE_WITH_KNOTS((6,1,1,1,1,1,1,1,1,1,1,1,1,1,1,1,1,1,1,1,1,1,
1,1,1,1,1,1,1,1,1,1,1,1,1,1,1,1,1,1,1,1,1,1,1,1,1,1,1,1,1,1,1,1,1,1,1,1,
1,1,1,1,1,1,1,6),(0.,0.0153846153846154,0.0307692307692308,0.0461538461538462,
0.0615384615384615,0.0769230769230769,0.0923076923076923,0.107692307692308,
0.123076923076923,0.138461538461538,0.153846153846154,0.169230769230769,
0.184615384615385,0.2,0.215384615384615,0.230769230769231,0.246153846153846,
0.261538461538462,0.276923076923077,0.292307692307692,0.307692307692308,
0.323076923076923,0.338461538461538,0.353846153846154,0.369230769230769,
0.384615384615385,0.4,0.415384615384615,0.430769230769231,0.446153846153846,
0.461538461538462,0.476923076923077,0.492307692307692,0.507692307692308,
0.523076923076923,0.538461538461538,0.553846153846154,0.569230769230769,
0.584615384615384,0.6,0.615384615384615,0.63076923076923,0.646153846153846,
0.661538461538461,0.676923076923076,0.692307692307692,0.707692307692307,
0.723076923076922,0.738461538461538,0.753846153846153,0.769230769230768,
0.784615384615384,0.799999999999999,0.815384615384614,0.83076923076923,
0.846153846153845,0.86153846153846,0.876923076923076,0.892307692307691,
0.907692307692306,0.923076923076922,0.938461538461537,0.953846153846152,
0.969230769230768,0.984615384615383,1.),.UNSPECIFIED.)
CURVE()
GEOMETRIC_REPRESENTATION_ITEM()
RATIONAL_B_SPLINE_CURVE((1.,1.,1.,1.,1.,1.,1.,1.,1.,1.,1.,1.,1.,1.,1.,1.,
1.,1.,1.,1.,1.,1.,1.,1.,1.,1.,1.,1.,1.,1.,1.,1.,1.,1.,1.,1.,1.,1.,1.,1.,
1.,1.,1.,1.,1.,1.,1.,1.,1.,1.,1.,1.,1.,1.,1.,1.,1.,1.,1.,1.,1.,1.,1.,1.,
1.,1.,1.,1.,1.,1.))
REPRESENTATION_ITEM('')
);
#135=(
BOUNDED_CURVE()
B_SPLINE_CURVE(5,(#22542,#22543,#22544,#22545,#22546,#22547,#22548,#22549,
#22550,#22551,#22552,#22553,#22554,#22555,#22556,#22557,#22558,#22559,#22560,
#22561,#22562,#22563,#22564,#22565,#22566,#22567,#22568,#22569,#22570,#22571,
#22572,#22573,#22574,#22575,#22576,#22577,#22578,#22579,#22580,#22581,#22582,
#22583,#22584,#22585,#22586,#22587,#22588,#22589,#22590,#22591,#22592,#22593,
#22594,#22595,#22596,#22597,#22598,#22599,#22600,#22601,#22602,#22603,#22604,
#22605,#22606,#22607,#22608,#22609,#22610,#22611),.UNSPECIFIED.,.F.,.F.)
B_SPLINE_CURVE_WITH_KNOTS((6,1,1,1,1,1,1,1,1,1,1,1,1,1,1,1,1,1,1,1,1,1,
1,1,1,1,1,1,1,1,1,1,1,1,1,1,1,1,1,1,1,1,1,1,1,1,1,1,1,1,1,1,1,1,1,1,1,1,
1,1,1,1,1,1,1,6),(0.,0.0153846153846154,0.0307692307692308,0.0461538461538462,
0.0615384615384615,0.0769230769230769,0.0923076923076923,0.107692307692308,
0.123076923076923,0.138461538461538,0.153846153846154,0.169230769230769,
0.184615384615385,0.2,0.215384615384615,0.230769230769231,0.246153846153846,
0.261538461538462,0.276923076923077,0.292307692307692,0.307692307692308,
0.323076923076923,0.338461538461538,0.353846153846154,0.369230769230769,
0.384615384615385,0.4,0.415384615384615,0.430769230769231,0.446153846153846,
0.461538461538462,0.476923076923077,0.492307692307692,0.507692307692308,
0.523076923076923,0.538461538461538,0.553846153846154,0.569230769230769,
0.584615384615384,0.6,0.615384615384615,0.63076923076923,0.646153846153846,
0.661538461538461,0.676923076923076,0.692307692307692,0.707692307692307,
0.723076923076922,0.738461538461538,0.753846153846153,0.769230769230768,
0.784615384615384,0.799999999999999,0.815384615384614,0.83076923076923,
0.846153846153845,0.86153846153846,0.876923076923076,0.892307692307691,
0.907692307692306,0.923076923076922,0.938461538461537,0.953846153846152,
0.969230769230768,0.984615384615383,1.),.UNSPECIFIED.)
CURVE()
GEOMETRIC_REPRESENTATION_ITEM()
RATIONAL_B_SPLINE_CURVE((1.,1.,1.,1.,1.,1.,1.,1.,1.,1.,1.,1.,1.,1.,1.,1.,
1.,1.,1.,1.,1.,1.,1.,1.,1.,1.,1.,1.,1.,1.,1.,1.,1.,1.,1.,1.,1.,1.,1.,1.,
1.,1.,1.,1.,1.,1.,1.,1.,1.,1.,1.,1.,1.,1.,1.,1.,1.,1.,1.,1.,1.,1.,1.,1.,
1.,1.,1.,1.,1.,1.))
REPRESENTATION_ITEM('')
);
#136=(
BOUNDED_CURVE()
B_SPLINE_CURVE(5,(#22615,#22616,#22617,#22618,#22619,#22620,#22621,#22622,
#22623,#22624,#22625,#22626,#22627,#22628,#22629,#22630,#22631,#22632,#22633,
#22634,#22635,#22636,#22637,#22638,#22639,#22640,#22641,#22642,#22643,#22644,
#22645,#22646,#22647,#22648,#22649,#22650,#22651,#22652,#22653,#22654,#22655,
#22656,#22657,#22658,#22659,#22660,#22661,#22662,#22663,#22664,#22665,#22666,
#22667,#22668,#22669,#22670,#22671,#22672,#22673,#22674,#22675,#22676,#22677,
#22678,#22679,#22680,#22681,#22682,#22683,#22684),.UNSPECIFIED.,.F.,.F.)
B_SPLINE_CURVE_WITH_KNOTS((6,1,1,1,1,1,1,1,1,1,1,1,1,1,1,1,1,1,1,1,1,1,
1,1,1,1,1,1,1,1,1,1,1,1,1,1,1,1,1,1,1,1,1,1,1,1,1,1,1,1,1,1,1,1,1,1,1,1,
1,1,1,1,1,1,1,6),(0.,0.0153846153846154,0.0307692307692308,0.0461538461538462,
0.0615384615384615,0.0769230769230769,0.0923076923076923,0.107692307692308,
0.123076923076923,0.138461538461538,0.153846153846154,0.169230769230769,
0.184615384615385,0.2,0.215384615384615,0.230769230769231,0.246153846153846,
0.261538461538462,0.276923076923077,0.292307692307692,0.307692307692308,
0.323076923076923,0.338461538461538,0.353846153846154,0.369230769230769,
0.384615384615385,0.4,0.415384615384615,0.430769230769231,0.446153846153846,
0.461538461538462,0.476923076923077,0.492307692307692,0.507692307692308,
0.523076923076923,0.538461538461538,0.553846153846154,0.569230769230769,
0.584615384615384,0.6,0.615384615384615,0.63076923076923,0.646153846153846,
0.661538461538461,0.676923076923076,0.692307692307692,0.707692307692307,
0.723076923076922,0.738461538461538,0.753846153846153,0.769230769230768,
0.784615384615384,0.799999999999999,0.815384615384614,0.83076923076923,
0.846153846153845,0.86153846153846,0.876923076923076,0.892307692307691,
0.907692307692306,0.923076923076922,0.938461538461537,0.953846153846152,
0.969230769230768,0.984615384615383,1.),.UNSPECIFIED.)
CURVE()
GEOMETRIC_REPRESENTATION_ITEM()
RATIONAL_B_SPLINE_CURVE((1.,1.,1.,1.,1.,1.,1.,1.,1.,1.,1.,1.,1.,1.,1.,1.,
1.,1.,1.,1.,1.,1.,1.,1.,1.,1.,1.,1.,1.,1.,1.,1.,1.,1.,1.,1.,1.,1.,1.,1.,
1.,1.,1.,1.,1.,1.,1.,1.,1.,1.,1.,1.,1.,1.,1.,1.,1.,1.,1.,1.,1.,1.,1.,1.,
1.,1.,1.,1.,1.,1.))
REPRESENTATION_ITEM('')
);
#137=(
BOUNDED_CURVE()
B_SPLINE_CURVE(5,(#22688,#22689,#22690,#22691,#22692,#22693,#22694,#22695,
#22696,#22697,#22698,#22699,#22700,#22701,#22702,#22703,#22704,#22705,#22706,
#22707,#22708,#22709,#22710,#22711,#22712,#22713,#22714,#22715,#22716,#22717,
#22718,#22719,#22720,#22721,#22722,#22723,#22724,#22725,#22726,#22727,#22728,
#22729,#22730,#22731,#22732,#22733,#22734,#22735,#22736,#22737,#22738,#22739,
#22740,#22741,#22742,#22743,#22744,#22745,#22746,#22747,#22748,#22749,#22750,
#22751,#22752,#22753,#22754,#22755,#22756,#22757),.UNSPECIFIED.,.F.,.F.)
B_SPLINE_CURVE_WITH_KNOTS((6,1,1,1,1,1,1,1,1,1,1,1,1,1,1,1,1,1,1,1,1,1,
1,1,1,1,1,1,1,1,1,1,1,1,1,1,1,1,1,1,1,1,1,1,1,1,1,1,1,1,1,1,1,1,1,1,1,1,
1,1,1,1,1,1,1,6),(0.,0.0153846153846154,0.0307692307692308,0.0461538461538462,
0.0615384615384615,0.0769230769230769,0.0923076923076923,0.107692307692308,
0.123076923076923,0.138461538461538,0.153846153846154,0.169230769230769,
0.184615384615385,0.2,0.215384615384615,0.230769230769231,0.246153846153846,
0.261538461538462,0.276923076923077,0.292307692307692,0.307692307692308,
0.323076923076923,0.338461538461538,0.353846153846154,0.369230769230769,
0.384615384615385,0.4,0.415384615384615,0.430769230769231,0.446153846153846,
0.461538461538462,0.476923076923077,0.492307692307692,0.507692307692308,
0.523076923076923,0.538461538461538,0.553846153846154,0.569230769230769,
0.584615384615384,0.6,0.615384615384615,0.63076923076923,0.646153846153846,
0.661538461538461,0.676923076923076,0.692307692307692,0.707692307692307,
0.723076923076922,0.738461538461538,0.753846153846153,0.769230769230768,
0.784615384615384,0.799999999999999,0.815384615384614,0.83076923076923,
0.846153846153845,0.86153846153846,0.876923076923076,0.892307692307691,
0.907692307692306,0.923076923076922,0.938461538461537,0.953846153846152,
0.969230769230768,0.984615384615383,1.),.UNSPECIFIED.)
CURVE()
GEOMETRIC_REPRESENTATION_ITEM()
RATIONAL_B_SPLINE_CURVE((1.,1.,1.,1.,1.,1.,1.,1.,1.,1.,1.,1.,1.,1.,1.,1.,
1.,1.,1.,1.,1.,1.,1.,1.,1.,1.,1.,1.,1.,1.,1.,1.,1.,1.,1.,1.,1.,1.,1.,1.,
1.,1.,1.,1.,1.,1.,1.,1.,1.,1.,1.,1.,1.,1.,1.,1.,1.,1.,1.,1.,1.,1.,1.,1.,
1.,1.,1.,1.,1.,1.))
REPRESENTATION_ITEM('')
);
#138=(
BOUNDED_CURVE()
B_SPLINE_CURVE(5,(#22761,#22762,#22763,#22764,#22765,#22766,#22767,#22768,
#22769,#22770,#22771,#22772,#22773,#22774,#22775,#22776,#22777,#22778,#22779,
#22780,#22781,#22782,#22783,#22784,#22785,#22786,#22787,#22788,#22789,#22790,
#22791,#22792,#22793,#22794,#22795,#22796,#22797,#22798,#22799,#22800,#22801,
#22802,#22803,#22804,#22805,#22806,#22807,#22808,#22809,#22810,#22811,#22812,
#22813,#22814,#22815,#22816,#22817,#22818,#22819,#22820,#22821,#22822,#22823,
#22824,#22825,#22826,#22827,#22828,#22829,#22830),.UNSPECIFIED.,.F.,.F.)
B_SPLINE_CURVE_WITH_KNOTS((6,1,1,1,1,1,1,1,1,1,1,1,1,1,1,1,1,1,1,1,1,1,
1,1,1,1,1,1,1,1,1,1,1,1,1,1,1,1,1,1,1,1,1,1,1,1,1,1,1,1,1,1,1,1,1,1,1,1,
1,1,1,1,1,1,1,6),(0.,0.0153846153846154,0.0307692307692308,0.0461538461538462,
0.0615384615384615,0.0769230769230769,0.0923076923076923,0.107692307692308,
0.123076923076923,0.138461538461538,0.153846153846154,0.169230769230769,
0.184615384615385,0.2,0.215384615384615,0.230769230769231,0.246153846153846,
0.261538461538462,0.276923076923077,0.292307692307692,0.307692307692308,
0.323076923076923,0.338461538461538,0.353846153846154,0.369230769230769,
0.384615384615385,0.4,0.415384615384615,0.430769230769231,0.446153846153846,
0.461538461538462,0.476923076923077,0.492307692307692,0.507692307692308,
0.523076923076923,0.538461538461538,0.553846153846154,0.569230769230769,
0.584615384615384,0.6,0.615384615384615,0.63076923076923,0.646153846153846,
0.661538461538461,0.676923076923076,0.692307692307692,0.707692307692307,
0.723076923076922,0.738461538461538,0.753846153846153,0.769230769230768,
0.784615384615384,0.799999999999999,0.815384615384614,0.83076923076923,
0.846153846153845,0.86153846153846,0.876923076923076,0.892307692307691,
0.907692307692306,0.923076923076922,0.938461538461537,0.953846153846152,
0.969230769230768,0.984615384615383,1.),.UNSPECIFIED.)
CURVE()
GEOMETRIC_REPRESENTATION_ITEM()
RATIONAL_B_SPLINE_CURVE((1.,1.,1.,1.,1.,1.,1.,1.,1.,1.,1.,1.,1.,1.,1.,1.,
1.,1.,1.,1.,1.,1.,1.,1.,1.,1.,1.,1.,1.,1.,1.,1.,1.,1.,1.,1.,1.,1.,1.,1.,
1.,1.,1.,1.,1.,1.,1.,1.,1.,1.,1.,1.,1.,1.,1.,1.,1.,1.,1.,1.,1.,1.,1.,1.,
1.,1.,1.,1.,1.,1.))
REPRESENTATION_ITEM('')
);
#139=(
BOUNDED_CURVE()
B_SPLINE_CURVE(5,(#22834,#22835,#22836,#22837,#22838,#22839,#22840,#22841,
#22842,#22843,#22844,#22845,#22846,#22847,#22848,#22849,#22850,#22851,#22852,
#22853,#22854,#22855,#22856,#22857,#22858,#22859,#22860,#22861,#22862,#22863,
#22864,#22865,#22866,#22867,#22868,#22869,#22870,#22871,#22872,#22873,#22874,
#22875,#22876,#22877,#22878,#22879,#22880,#22881,#22882,#22883,#22884,#22885,
#22886,#22887,#22888,#22889,#22890,#22891,#22892,#22893,#22894,#22895,#22896,
#22897,#22898,#22899,#22900,#22901,#22902,#22903),.UNSPECIFIED.,.F.,.F.)
B_SPLINE_CURVE_WITH_KNOTS((6,1,1,1,1,1,1,1,1,1,1,1,1,1,1,1,1,1,1,1,1,1,
1,1,1,1,1,1,1,1,1,1,1,1,1,1,1,1,1,1,1,1,1,1,1,1,1,1,1,1,1,1,1,1,1,1,1,1,
1,1,1,1,1,1,1,6),(0.,0.0153846153846154,0.0307692307692308,0.0461538461538462,
0.0615384615384615,0.0769230769230769,0.0923076923076923,0.107692307692308,
0.123076923076923,0.138461538461538,0.153846153846154,0.169230769230769,
0.184615384615385,0.2,0.215384615384615,0.230769230769231,0.246153846153846,
0.261538461538462,0.276923076923077,0.292307692307692,0.307692307692308,
0.323076923076923,0.338461538461538,0.353846153846154,0.369230769230769,
0.384615384615385,0.4,0.415384615384615,0.430769230769231,0.446153846153846,
0.461538461538462,0.476923076923077,0.492307692307692,0.507692307692308,
0.523076923076923,0.538461538461538,0.553846153846154,0.569230769230769,
0.584615384615384,0.6,0.615384615384615,0.63076923076923,0.646153846153846,
0.661538461538461,0.676923076923076,0.692307692307692,0.707692307692307,
0.723076923076922,0.738461538461538,0.753846153846153,0.769230769230768,
0.784615384615384,0.799999999999999,0.815384615384614,0.83076923076923,
0.846153846153845,0.86153846153846,0.876923076923076,0.892307692307691,
0.907692307692306,0.923076923076922,0.938461538461537,0.953846153846152,
0.969230769230768,0.984615384615383,1.),.UNSPECIFIED.)
CURVE()
GEOMETRIC_REPRESENTATION_ITEM()
RATIONAL_B_SPLINE_CURVE((1.,1.,1.,1.,1.,1.,1.,1.,1.,1.,1.,1.,1.,1.,1.,1.,
1.,1.,1.,1.,1.,1.,1.,1.,1.,1.,1.,1.,1.,1.,1.,1.,1.,1.,1.,1.,1.,1.,1.,1.,
1.,1.,1.,1.,1.,1.,1.,1.,1.,1.,1.,1.,1.,1.,1.,1.,1.,1.,1.,1.,1.,1.,1.,1.,
1.,1.,1.,1.,1.,1.))
REPRESENTATION_ITEM('')
);
#140=(
BOUNDED_CURVE()
B_SPLINE_CURVE(5,(#22907,#22908,#22909,#22910,#22911,#22912,#22913,#22914,
#22915,#22916,#22917,#22918,#22919,#22920,#22921,#22922,#22923,#22924,#22925,
#22926,#22927,#22928,#22929,#22930,#22931,#22932,#22933,#22934,#22935,#22936,
#22937,#22938,#22939,#22940,#22941,#22942,#22943,#22944,#22945,#22946,#22947,
#22948,#22949,#22950,#22951,#22952,#22953,#22954,#22955,#22956,#22957,#22958,
#22959,#22960,#22961,#22962,#22963,#22964,#22965,#22966,#22967,#22968,#22969,
#22970,#22971,#22972,#22973,#22974,#22975,#22976),.UNSPECIFIED.,.F.,.F.)
B_SPLINE_CURVE_WITH_KNOTS((6,1,1,1,1,1,1,1,1,1,1,1,1,1,1,1,1,1,1,1,1,1,
1,1,1,1,1,1,1,1,1,1,1,1,1,1,1,1,1,1,1,1,1,1,1,1,1,1,1,1,1,1,1,1,1,1,1,1,
1,1,1,1,1,1,1,6),(0.,0.0153846153846154,0.0307692307692308,0.0461538461538462,
0.0615384615384615,0.0769230769230769,0.0923076923076923,0.107692307692308,
0.123076923076923,0.138461538461538,0.153846153846154,0.169230769230769,
0.184615384615385,0.2,0.215384615384615,0.230769230769231,0.246153846153846,
0.261538461538462,0.276923076923077,0.292307692307692,0.307692307692308,
0.323076923076923,0.338461538461538,0.353846153846154,0.369230769230769,
0.384615384615385,0.4,0.415384615384615,0.430769230769231,0.446153846153846,
0.461538461538462,0.476923076923077,0.492307692307692,0.507692307692308,
0.523076923076923,0.538461538461538,0.553846153846154,0.569230769230769,
0.584615384615384,0.6,0.615384615384615,0.63076923076923,0.646153846153846,
0.661538461538461,0.676923076923076,0.692307692307692,0.707692307692307,
0.723076923076922,0.738461538461538,0.753846153846153,0.769230769230768,
0.784615384615384,0.799999999999999,0.815384615384614,0.83076923076923,
0.846153846153845,0.86153846153846,0.876923076923076,0.892307692307691,
0.907692307692306,0.923076923076922,0.938461538461537,0.953846153846152,
0.969230769230768,0.984615384615383,1.),.UNSPECIFIED.)
CURVE()
GEOMETRIC_REPRESENTATION_ITEM()
RATIONAL_B_SPLINE_CURVE((1.,1.,1.,1.,1.,1.,1.,1.,1.,1.,1.,1.,1.,1.,1.,1.,
1.,1.,1.,1.,1.,1.,1.,1.,1.,1.,1.,1.,1.,1.,1.,1.,1.,1.,1.,1.,1.,1.,1.,1.,
1.,1.,1.,1.,1.,1.,1.,1.,1.,1.,1.,1.,1.,1.,1.,1.,1.,1.,1.,1.,1.,1.,1.,1.,
1.,1.,1.,1.,1.,1.))
REPRESENTATION_ITEM('')
);
#141=(
BOUNDED_CURVE()
B_SPLINE_CURVE(5,(#22980,#22981,#22982,#22983,#22984,#22985,#22986,#22987,
#22988,#22989,#22990,#22991,#22992,#22993,#22994,#22995,#22996,#22997,#22998,
#22999,#23000,#23001,#23002,#23003,#23004,#23005,#23006,#23007,#23008,#23009,
#23010,#23011,#23012,#23013,#23014,#23015,#23016,#23017,#23018,#23019,#23020,
#23021,#23022,#23023,#23024,#23025,#23026,#23027,#23028,#23029,#23030,#23031,
#23032,#23033,#23034,#23035,#23036,#23037,#23038,#23039,#23040,#23041,#23042,
#23043,#23044,#23045,#23046,#23047,#23048,#23049),.UNSPECIFIED.,.F.,.F.)
B_SPLINE_CURVE_WITH_KNOTS((6,1,1,1,1,1,1,1,1,1,1,1,1,1,1,1,1,1,1,1,1,1,
1,1,1,1,1,1,1,1,1,1,1,1,1,1,1,1,1,1,1,1,1,1,1,1,1,1,1,1,1,1,1,1,1,1,1,1,
1,1,1,1,1,1,1,6),(0.,0.0153846153846154,0.0307692307692308,0.0461538461538462,
0.0615384615384615,0.0769230769230769,0.0923076923076923,0.107692307692308,
0.123076923076923,0.138461538461538,0.153846153846154,0.169230769230769,
0.184615384615385,0.2,0.215384615384615,0.230769230769231,0.246153846153846,
0.261538461538462,0.276923076923077,0.292307692307692,0.307692307692308,
0.323076923076923,0.338461538461538,0.353846153846154,0.369230769230769,
0.384615384615385,0.4,0.415384615384615,0.430769230769231,0.446153846153846,
0.461538461538462,0.476923076923077,0.492307692307692,0.507692307692308,
0.523076923076923,0.538461538461538,0.553846153846154,0.569230769230769,
0.584615384615384,0.6,0.615384615384615,0.63076923076923,0.646153846153846,
0.661538461538461,0.676923076923076,0.692307692307692,0.707692307692307,
0.723076923076922,0.738461538461538,0.753846153846153,0.769230769230768,
0.784615384615384,0.799999999999999,0.815384615384614,0.83076923076923,
0.846153846153845,0.86153846153846,0.876923076923076,0.892307692307691,
0.907692307692306,0.923076923076922,0.938461538461537,0.953846153846152,
0.969230769230768,0.984615384615383,1.),.UNSPECIFIED.)
CURVE()
GEOMETRIC_REPRESENTATION_ITEM()
RATIONAL_B_SPLINE_CURVE((1.,1.,1.,1.,1.,1.,1.,1.,1.,1.,1.,1.,1.,1.,1.,1.,
1.,1.,1.,1.,1.,1.,1.,1.,1.,1.,1.,1.,1.,1.,1.,1.,1.,1.,1.,1.,1.,1.,1.,1.,
1.,1.,1.,1.,1.,1.,1.,1.,1.,1.,1.,1.,1.,1.,1.,1.,1.,1.,1.,1.,1.,1.,1.,1.,
1.,1.,1.,1.,1.,1.))
REPRESENTATION_ITEM('')
);
#142=(
BOUNDED_CURVE()
B_SPLINE_CURVE(5,(#23053,#23054,#23055,#23056,#23057,#23058,#23059,#23060,
#23061,#23062,#23063,#23064,#23065,#23066,#23067,#23068,#23069,#23070,#23071,
#23072,#23073,#23074,#23075,#23076,#23077,#23078,#23079,#23080,#23081,#23082,
#23083,#23084,#23085,#23086,#23087,#23088,#23089,#23090,#23091,#23092,#23093,
#23094,#23095,#23096,#23097,#23098,#23099,#23100,#23101,#23102,#23103,#23104,
#23105,#23106,#23107,#23108,#23109,#23110,#23111,#23112,#23113,#23114,#23115,
#23116,#23117,#23118,#23119,#23120,#23121,#23122),.UNSPECIFIED.,.F.,.F.)
B_SPLINE_CURVE_WITH_KNOTS((6,1,1,1,1,1,1,1,1,1,1,1,1,1,1,1,1,1,1,1,1,1,
1,1,1,1,1,1,1,1,1,1,1,1,1,1,1,1,1,1,1,1,1,1,1,1,1,1,1,1,1,1,1,1,1,1,1,1,
1,1,1,1,1,1,1,6),(0.,0.0153846153846154,0.0307692307692308,0.0461538461538462,
0.0615384615384615,0.0769230769230769,0.0923076923076923,0.107692307692308,
0.123076923076923,0.138461538461538,0.153846153846154,0.169230769230769,
0.184615384615385,0.2,0.215384615384615,0.230769230769231,0.246153846153846,
0.261538461538462,0.276923076923077,0.292307692307692,0.307692307692308,
0.323076923076923,0.338461538461538,0.353846153846154,0.369230769230769,
0.384615384615385,0.4,0.415384615384615,0.430769230769231,0.446153846153846,
0.461538461538462,0.476923076923077,0.492307692307692,0.507692307692308,
0.523076923076923,0.538461538461538,0.553846153846154,0.569230769230769,
0.584615384615384,0.6,0.615384615384615,0.63076923076923,0.646153846153846,
0.661538461538461,0.676923076923076,0.692307692307692,0.707692307692307,
0.723076923076922,0.738461538461538,0.753846153846153,0.769230769230768,
0.784615384615384,0.799999999999999,0.815384615384614,0.83076923076923,
0.846153846153845,0.86153846153846,0.876923076923076,0.892307692307691,
0.907692307692306,0.923076923076922,0.938461538461537,0.953846153846152,
0.969230769230768,0.984615384615383,1.),.UNSPECIFIED.)
CURVE()
GEOMETRIC_REPRESENTATION_ITEM()
RATIONAL_B_SPLINE_CURVE((1.,1.,1.,1.,1.,1.,1.,1.,1.,1.,1.,1.,1.,1.,1.,1.,
1.,1.,1.,1.,1.,1.,1.,1.,1.,1.,1.,1.,1.,1.,1.,1.,1.,1.,1.,1.,1.,1.,1.,1.,
1.,1.,1.,1.,1.,1.,1.,1.,1.,1.,1.,1.,1.,1.,1.,1.,1.,1.,1.,1.,1.,1.,1.,1.,
1.,1.,1.,1.,1.,1.))
REPRESENTATION_ITEM('')
);
#143=(
BOUNDED_CURVE()
B_SPLINE_CURVE(5,(#23126,#23127,#23128,#23129,#23130,#23131,#23132,#23133,
#23134,#23135,#23136,#23137,#23138,#23139,#23140,#23141,#23142,#23143,#23144,
#23145,#23146,#23147,#23148,#23149,#23150,#23151,#23152,#23153,#23154,#23155,
#23156,#23157,#23158,#23159,#23160,#23161,#23162,#23163,#23164,#23165,#23166,
#23167,#23168,#23169,#23170,#23171,#23172,#23173,#23174,#23175,#23176,#23177,
#23178,#23179,#23180,#23181,#23182,#23183,#23184,#23185,#23186,#23187,#23188,
#23189,#23190,#23191,#23192,#23193,#23194,#23195),.UNSPECIFIED.,.F.,.F.)
B_SPLINE_CURVE_WITH_KNOTS((6,1,1,1,1,1,1,1,1,1,1,1,1,1,1,1,1,1,1,1,1,1,
1,1,1,1,1,1,1,1,1,1,1,1,1,1,1,1,1,1,1,1,1,1,1,1,1,1,1,1,1,1,1,1,1,1,1,1,
1,1,1,1,1,1,1,6),(0.,0.0153846153846154,0.0307692307692308,0.0461538461538462,
0.0615384615384615,0.0769230769230769,0.0923076923076923,0.107692307692308,
0.123076923076923,0.138461538461538,0.153846153846154,0.169230769230769,
0.184615384615385,0.2,0.215384615384615,0.230769230769231,0.246153846153846,
0.261538461538462,0.276923076923077,0.292307692307692,0.307692307692308,
0.323076923076923,0.338461538461538,0.353846153846154,0.369230769230769,
0.384615384615385,0.4,0.415384615384615,0.430769230769231,0.446153846153846,
0.461538461538462,0.476923076923077,0.492307692307692,0.507692307692308,
0.523076923076923,0.538461538461538,0.553846153846154,0.569230769230769,
0.584615384615384,0.6,0.615384615384615,0.63076923076923,0.646153846153846,
0.661538461538461,0.676923076923076,0.692307692307692,0.707692307692307,
0.723076923076922,0.738461538461538,0.753846153846153,0.769230769230768,
0.784615384615384,0.799999999999999,0.815384615384614,0.83076923076923,
0.846153846153845,0.86153846153846,0.876923076923076,0.892307692307691,
0.907692307692306,0.923076923076922,0.938461538461537,0.953846153846152,
0.969230769230768,0.984615384615383,1.),.UNSPECIFIED.)
CURVE()
GEOMETRIC_REPRESENTATION_ITEM()
RATIONAL_B_SPLINE_CURVE((1.,1.,1.,1.,1.,1.,1.,1.,1.,1.,1.,1.,1.,1.,1.,1.,
1.,1.,1.,1.,1.,1.,1.,1.,1.,1.,1.,1.,1.,1.,1.,1.,1.,1.,1.,1.,1.,1.,1.,1.,
1.,1.,1.,1.,1.,1.,1.,1.,1.,1.,1.,1.,1.,1.,1.,1.,1.,1.,1.,1.,1.,1.,1.,1.,
1.,1.,1.,1.,1.,1.))
REPRESENTATION_ITEM('')
);
#144=(
BOUNDED_CURVE()
B_SPLINE_CURVE(5,(#23199,#23200,#23201,#23202,#23203,#23204,#23205,#23206,
#23207,#23208,#23209,#23210,#23211,#23212,#23213,#23214,#23215,#23216,#23217,
#23218,#23219,#23220,#23221,#23222,#23223,#23224,#23225,#23226,#23227,#23228,
#23229,#23230,#23231,#23232,#23233,#23234,#23235,#23236,#23237,#23238,#23239,
#23240,#23241,#23242,#23243,#23244,#23245,#23246,#23247,#23248,#23249,#23250,
#23251,#23252,#23253,#23254,#23255,#23256,#23257,#23258,#23259,#23260,#23261,
#23262,#23263,#23264,#23265,#23266,#23267,#23268),.UNSPECIFIED.,.F.,.F.)
B_SPLINE_CURVE_WITH_KNOTS((6,1,1,1,1,1,1,1,1,1,1,1,1,1,1,1,1,1,1,1,1,1,
1,1,1,1,1,1,1,1,1,1,1,1,1,1,1,1,1,1,1,1,1,1,1,1,1,1,1,1,1,1,1,1,1,1,1,1,
1,1,1,1,1,1,1,6),(0.,0.0153846153846154,0.0307692307692308,0.0461538461538462,
0.0615384615384615,0.0769230769230769,0.0923076923076923,0.107692307692308,
0.123076923076923,0.138461538461538,0.153846153846154,0.169230769230769,
0.184615384615385,0.2,0.215384615384615,0.230769230769231,0.246153846153846,
0.261538461538462,0.276923076923077,0.292307692307692,0.307692307692308,
0.323076923076923,0.338461538461538,0.353846153846154,0.369230769230769,
0.384615384615385,0.4,0.415384615384615,0.430769230769231,0.446153846153846,
0.461538461538462,0.476923076923077,0.492307692307692,0.507692307692308,
0.523076923076923,0.538461538461538,0.553846153846154,0.569230769230769,
0.584615384615384,0.6,0.615384615384615,0.63076923076923,0.646153846153846,
0.661538461538461,0.676923076923076,0.692307692307692,0.707692307692307,
0.723076923076922,0.738461538461538,0.753846153846153,0.769230769230768,
0.784615384615384,0.799999999999999,0.815384615384614,0.83076923076923,
0.846153846153845,0.86153846153846,0.876923076923076,0.892307692307691,
0.907692307692306,0.923076923076922,0.938461538461537,0.953846153846152,
0.969230769230768,0.984615384615383,1.),.UNSPECIFIED.)
CURVE()
GEOMETRIC_REPRESENTATION_ITEM()
RATIONAL_B_SPLINE_CURVE((1.,1.,1.,1.,1.,1.,1.,1.,1.,1.,1.,1.,1.,1.,1.,1.,
1.,1.,1.,1.,1.,1.,1.,1.,1.,1.,1.,1.,1.,1.,1.,1.,1.,1.,1.,1.,1.,1.,1.,1.,
1.,1.,1.,1.,1.,1.,1.,1.,1.,1.,1.,1.,1.,1.,1.,1.,1.,1.,1.,1.,1.,1.,1.,1.,
1.,1.,1.,1.,1.,1.))
REPRESENTATION_ITEM('')
);
#145=(
BOUNDED_CURVE()
B_SPLINE_CURVE(5,(#23272,#23273,#23274,#23275,#23276,#23277,#23278,#23279,
#23280,#23281,#23282,#23283,#23284,#23285,#23286,#23287,#23288,#23289,#23290,
#23291,#23292,#23293,#23294,#23295,#23296,#23297,#23298,#23299,#23300,#23301,
#23302,#23303,#23304,#23305,#23306,#23307,#23308,#23309,#23310,#23311,#23312,
#23313,#23314,#23315,#23316,#23317,#23318,#23319,#23320,#23321,#23322,#23323,
#23324,#23325,#23326,#23327,#23328,#23329,#23330,#23331,#23332,#23333,#23334,
#23335,#23336,#23337,#23338,#23339,#23340,#23341),.UNSPECIFIED.,.F.,.F.)
B_SPLINE_CURVE_WITH_KNOTS((6,1,1,1,1,1,1,1,1,1,1,1,1,1,1,1,1,1,1,1,1,1,
1,1,1,1,1,1,1,1,1,1,1,1,1,1,1,1,1,1,1,1,1,1,1,1,1,1,1,1,1,1,1,1,1,1,1,1,
1,1,1,1,1,1,1,6),(0.,0.0153846153846154,0.0307692307692308,0.0461538461538462,
0.0615384615384615,0.0769230769230769,0.0923076923076923,0.107692307692308,
0.123076923076923,0.138461538461538,0.153846153846154,0.169230769230769,
0.184615384615385,0.2,0.215384615384615,0.230769230769231,0.246153846153846,
0.261538461538462,0.276923076923077,0.292307692307692,0.307692307692308,
0.323076923076923,0.338461538461538,0.353846153846154,0.369230769230769,
0.384615384615385,0.4,0.415384615384615,0.430769230769231,0.446153846153846,
0.461538461538462,0.476923076923077,0.492307692307692,0.507692307692308,
0.523076923076923,0.538461538461538,0.553846153846154,0.569230769230769,
0.584615384615384,0.6,0.615384615384615,0.63076923076923,0.646153846153846,
0.661538461538461,0.676923076923076,0.692307692307692,0.707692307692307,
0.723076923076922,0.738461538461538,0.753846153846153,0.769230769230768,
0.784615384615384,0.799999999999999,0.815384615384614,0.83076923076923,
0.846153846153845,0.86153846153846,0.876923076923076,0.892307692307691,
0.907692307692306,0.923076923076922,0.938461538461537,0.953846153846152,
0.969230769230768,0.984615384615383,1.),.UNSPECIFIED.)
CURVE()
GEOMETRIC_REPRESENTATION_ITEM()
RATIONAL_B_SPLINE_CURVE((1.,1.,1.,1.,1.,1.,1.,1.,1.,1.,1.,1.,1.,1.,1.,1.,
1.,1.,1.,1.,1.,1.,1.,1.,1.,1.,1.,1.,1.,1.,1.,1.,1.,1.,1.,1.,1.,1.,1.,1.,
1.,1.,1.,1.,1.,1.,1.,1.,1.,1.,1.,1.,1.,1.,1.,1.,1.,1.,1.,1.,1.,1.,1.,1.,
1.,1.,1.,1.,1.,1.))
REPRESENTATION_ITEM('')
);
#146=(
BOUNDED_CURVE()
B_SPLINE_CURVE(5,(#23345,#23346,#23347,#23348,#23349,#23350,#23351,#23352,
#23353,#23354,#23355,#23356,#23357,#23358,#23359,#23360,#23361,#23362,#23363,
#23364,#23365,#23366,#23367,#23368,#23369,#23370,#23371,#23372,#23373,#23374,
#23375,#23376,#23377,#23378,#23379,#23380,#23381,#23382,#23383,#23384,#23385,
#23386,#23387,#23388,#23389,#23390,#23391,#23392,#23393,#23394,#23395,#23396,
#23397,#23398,#23399,#23400,#23401,#23402,#23403,#23404,#23405,#23406,#23407,
#23408,#23409,#23410,#23411,#23412,#23413,#23414),.UNSPECIFIED.,.F.,.F.)
B_SPLINE_CURVE_WITH_KNOTS((6,1,1,1,1,1,1,1,1,1,1,1,1,1,1,1,1,1,1,1,1,1,
1,1,1,1,1,1,1,1,1,1,1,1,1,1,1,1,1,1,1,1,1,1,1,1,1,1,1,1,1,1,1,1,1,1,1,1,
1,1,1,1,1,1,1,6),(0.,0.0153846153846154,0.0307692307692308,0.0461538461538462,
0.0615384615384615,0.0769230769230769,0.0923076923076923,0.107692307692308,
0.123076923076923,0.138461538461538,0.153846153846154,0.169230769230769,
0.184615384615385,0.2,0.215384615384615,0.230769230769231,0.246153846153846,
0.261538461538462,0.276923076923077,0.292307692307692,0.307692307692308,
0.323076923076923,0.338461538461538,0.353846153846154,0.369230769230769,
0.384615384615385,0.4,0.415384615384615,0.430769230769231,0.446153846153846,
0.461538461538462,0.476923076923077,0.492307692307692,0.507692307692308,
0.523076923076923,0.538461538461538,0.553846153846154,0.569230769230769,
0.584615384615384,0.6,0.615384615384615,0.63076923076923,0.646153846153846,
0.661538461538461,0.676923076923076,0.692307692307692,0.707692307692307,
0.723076923076922,0.738461538461538,0.753846153846153,0.769230769230768,
0.784615384615384,0.799999999999999,0.815384615384614,0.83076923076923,
0.846153846153845,0.86153846153846,0.876923076923076,0.892307692307691,
0.907692307692306,0.923076923076922,0.938461538461537,0.953846153846152,
0.969230769230768,0.984615384615383,1.),.UNSPECIFIED.)
CURVE()
GEOMETRIC_REPRESENTATION_ITEM()
RATIONAL_B_SPLINE_CURVE((1.,1.,1.,1.,1.,1.,1.,1.,1.,1.,1.,1.,1.,1.,1.,1.,
1.,1.,1.,1.,1.,1.,1.,1.,1.,1.,1.,1.,1.,1.,1.,1.,1.,1.,1.,1.,1.,1.,1.,1.,
1.,1.,1.,1.,1.,1.,1.,1.,1.,1.,1.,1.,1.,1.,1.,1.,1.,1.,1.,1.,1.,1.,1.,1.,
1.,1.,1.,1.,1.,1.))
REPRESENTATION_ITEM('')
);
#147=(
BOUNDED_CURVE()
B_SPLINE_CURVE(5,(#23418,#23419,#23420,#23421,#23422,#23423,#23424,#23425,
#23426,#23427,#23428,#23429,#23430,#23431,#23432,#23433,#23434,#23435,#23436,
#23437,#23438,#23439,#23440,#23441,#23442,#23443,#23444,#23445,#23446,#23447,
#23448,#23449,#23450,#23451,#23452,#23453,#23454,#23455,#23456,#23457,#23458,
#23459,#23460,#23461,#23462,#23463,#23464,#23465,#23466,#23467,#23468,#23469,
#23470,#23471,#23472,#23473,#23474,#23475,#23476,#23477,#23478,#23479,#23480,
#23481,#23482,#23483,#23484,#23485,#23486,#23487),.UNSPECIFIED.,.F.,.F.)
B_SPLINE_CURVE_WITH_KNOTS((6,1,1,1,1,1,1,1,1,1,1,1,1,1,1,1,1,1,1,1,1,1,
1,1,1,1,1,1,1,1,1,1,1,1,1,1,1,1,1,1,1,1,1,1,1,1,1,1,1,1,1,1,1,1,1,1,1,1,
1,1,1,1,1,1,1,6),(0.,0.0153846153846154,0.0307692307692308,0.0461538461538462,
0.0615384615384615,0.0769230769230769,0.0923076923076923,0.107692307692308,
0.123076923076923,0.138461538461538,0.153846153846154,0.169230769230769,
0.184615384615385,0.2,0.215384615384615,0.230769230769231,0.246153846153846,
0.261538461538462,0.276923076923077,0.292307692307692,0.307692307692308,
0.323076923076923,0.338461538461538,0.353846153846154,0.369230769230769,
0.384615384615385,0.4,0.415384615384615,0.430769230769231,0.446153846153846,
0.461538461538462,0.476923076923077,0.492307692307692,0.507692307692308,
0.523076923076923,0.538461538461538,0.553846153846154,0.569230769230769,
0.584615384615384,0.6,0.615384615384615,0.63076923076923,0.646153846153846,
0.661538461538461,0.676923076923076,0.692307692307692,0.707692307692307,
0.723076923076922,0.738461538461538,0.753846153846153,0.769230769230768,
0.784615384615384,0.799999999999999,0.815384615384614,0.83076923076923,
0.846153846153845,0.86153846153846,0.876923076923076,0.892307692307691,
0.907692307692306,0.923076923076922,0.938461538461537,0.953846153846152,
0.969230769230768,0.984615384615383,1.),.UNSPECIFIED.)
CURVE()
GEOMETRIC_REPRESENTATION_ITEM()
RATIONAL_B_SPLINE_CURVE((1.,1.,1.,1.,1.,1.,1.,1.,1.,1.,1.,1.,1.,1.,1.,1.,
1.,1.,1.,1.,1.,1.,1.,1.,1.,1.,1.,1.,1.,1.,1.,1.,1.,1.,1.,1.,1.,1.,1.,1.,
1.,1.,1.,1.,1.,1.,1.,1.,1.,1.,1.,1.,1.,1.,1.,1.,1.,1.,1.,1.,1.,1.,1.,1.,
1.,1.,1.,1.,1.,1.))
REPRESENTATION_ITEM('')
);
#148=(
BOUNDED_CURVE()
B_SPLINE_CURVE(5,(#23491,#23492,#23493,#23494,#23495,#23496,#23497,#23498,
#23499,#23500,#23501,#23502,#23503,#23504,#23505,#23506,#23507,#23508,#23509,
#23510,#23511,#23512,#23513,#23514,#23515,#23516,#23517,#23518,#23519,#23520,
#23521,#23522,#23523,#23524,#23525,#23526,#23527,#23528,#23529,#23530,#23531,
#23532,#23533,#23534,#23535,#23536,#23537,#23538,#23539,#23540,#23541,#23542,
#23543,#23544,#23545,#23546,#23547,#23548,#23549,#23550,#23551,#23552,#23553,
#23554,#23555,#23556,#23557,#23558,#23559,#23560),.UNSPECIFIED.,.F.,.F.)
B_SPLINE_CURVE_WITH_KNOTS((6,1,1,1,1,1,1,1,1,1,1,1,1,1,1,1,1,1,1,1,1,1,
1,1,1,1,1,1,1,1,1,1,1,1,1,1,1,1,1,1,1,1,1,1,1,1,1,1,1,1,1,1,1,1,1,1,1,1,
1,1,1,1,1,1,1,6),(0.,0.0153846153846154,0.0307692307692308,0.0461538461538462,
0.0615384615384615,0.0769230769230769,0.0923076923076923,0.107692307692308,
0.123076923076923,0.138461538461538,0.153846153846154,0.169230769230769,
0.184615384615385,0.2,0.215384615384615,0.230769230769231,0.246153846153846,
0.261538461538462,0.276923076923077,0.292307692307692,0.307692307692308,
0.323076923076923,0.338461538461538,0.353846153846154,0.369230769230769,
0.384615384615385,0.4,0.415384615384615,0.430769230769231,0.446153846153846,
0.461538461538462,0.476923076923077,0.492307692307692,0.507692307692308,
0.523076923076923,0.538461538461538,0.553846153846154,0.569230769230769,
0.584615384615384,0.6,0.615384615384615,0.63076923076923,0.646153846153846,
0.661538461538461,0.676923076923076,0.692307692307692,0.707692307692307,
0.723076923076922,0.738461538461538,0.753846153846153,0.769230769230768,
0.784615384615384,0.799999999999999,0.815384615384614,0.83076923076923,
0.846153846153845,0.86153846153846,0.876923076923076,0.892307692307691,
0.907692307692306,0.923076923076922,0.938461538461537,0.953846153846152,
0.969230769230768,0.984615384615383,1.),.UNSPECIFIED.)
CURVE()
GEOMETRIC_REPRESENTATION_ITEM()
RATIONAL_B_SPLINE_CURVE((1.,1.,1.,1.,1.,1.,1.,1.,1.,1.,1.,1.,1.,1.,1.,1.,
1.,1.,1.,1.,1.,1.,1.,1.,1.,1.,1.,1.,1.,1.,1.,1.,1.,1.,1.,1.,1.,1.,1.,1.,
1.,1.,1.,1.,1.,1.,1.,1.,1.,1.,1.,1.,1.,1.,1.,1.,1.,1.,1.,1.,1.,1.,1.,1.,
1.,1.,1.,1.,1.,1.))
REPRESENTATION_ITEM('')
);
#149=(
BOUNDED_CURVE()
B_SPLINE_CURVE(5,(#23564,#23565,#23566,#23567,#23568,#23569,#23570,#23571,
#23572,#23573,#23574,#23575,#23576,#23577,#23578,#23579,#23580,#23581,#23582,
#23583,#23584,#23585,#23586,#23587,#23588,#23589,#23590,#23591,#23592,#23593,
#23594,#23595,#23596,#23597,#23598,#23599,#23600,#23601,#23602,#23603,#23604,
#23605,#23606,#23607,#23608,#23609,#23610,#23611,#23612,#23613,#23614,#23615,
#23616,#23617,#23618,#23619,#23620,#23621,#23622,#23623,#23624,#23625,#23626,
#23627,#23628,#23629,#23630,#23631,#23632,#23633),.UNSPECIFIED.,.F.,.F.)
B_SPLINE_CURVE_WITH_KNOTS((6,1,1,1,1,1,1,1,1,1,1,1,1,1,1,1,1,1,1,1,1,1,
1,1,1,1,1,1,1,1,1,1,1,1,1,1,1,1,1,1,1,1,1,1,1,1,1,1,1,1,1,1,1,1,1,1,1,1,
1,1,1,1,1,1,1,6),(0.,0.0153846153846154,0.0307692307692308,0.0461538461538462,
0.0615384615384615,0.0769230769230769,0.0923076923076923,0.107692307692308,
0.123076923076923,0.138461538461538,0.153846153846154,0.169230769230769,
0.184615384615385,0.2,0.215384615384615,0.230769230769231,0.246153846153846,
0.261538461538462,0.276923076923077,0.292307692307692,0.307692307692308,
0.323076923076923,0.338461538461538,0.353846153846154,0.369230769230769,
0.384615384615385,0.4,0.415384615384615,0.430769230769231,0.446153846153846,
0.461538461538462,0.476923076923077,0.492307692307692,0.507692307692308,
0.523076923076923,0.538461538461538,0.553846153846154,0.569230769230769,
0.584615384615384,0.6,0.615384615384615,0.63076923076923,0.646153846153846,
0.661538461538461,0.676923076923076,0.692307692307692,0.707692307692307,
0.723076923076922,0.738461538461538,0.753846153846153,0.769230769230768,
0.784615384615384,0.799999999999999,0.815384615384614,0.83076923076923,
0.846153846153845,0.86153846153846,0.876923076923076,0.892307692307691,
0.907692307692306,0.923076923076922,0.938461538461537,0.953846153846152,
0.969230769230768,0.984615384615383,1.),.UNSPECIFIED.)
CURVE()
GEOMETRIC_REPRESENTATION_ITEM()
RATIONAL_B_SPLINE_CURVE((1.,1.,1.,1.,1.,1.,1.,1.,1.,1.,1.,1.,1.,1.,1.,1.,
1.,1.,1.,1.,1.,1.,1.,1.,1.,1.,1.,1.,1.,1.,1.,1.,1.,1.,1.,1.,1.,1.,1.,1.,
1.,1.,1.,1.,1.,1.,1.,1.,1.,1.,1.,1.,1.,1.,1.,1.,1.,1.,1.,1.,1.,1.,1.,1.,
1.,1.,1.,1.,1.,1.))
REPRESENTATION_ITEM('')
);
#150=(
BOUNDED_CURVE()
B_SPLINE_CURVE(5,(#23637,#23638,#23639,#23640,#23641,#23642,#23643,#23644,
#23645,#23646,#23647,#23648,#23649,#23650,#23651,#23652,#23653,#23654,#23655,
#23656,#23657,#23658,#23659,#23660,#23661,#23662,#23663,#23664,#23665,#23666,
#23667,#23668,#23669,#23670,#23671,#23672,#23673,#23674,#23675,#23676,#23677,
#23678,#23679,#23680,#23681,#23682,#23683,#23684,#23685,#23686,#23687,#23688,
#23689,#23690,#23691,#23692,#23693,#23694,#23695,#23696,#23697,#23698,#23699,
#23700,#23701,#23702,#23703,#23704,#23705,#23706),.UNSPECIFIED.,.F.,.F.)
B_SPLINE_CURVE_WITH_KNOTS((6,1,1,1,1,1,1,1,1,1,1,1,1,1,1,1,1,1,1,1,1,1,
1,1,1,1,1,1,1,1,1,1,1,1,1,1,1,1,1,1,1,1,1,1,1,1,1,1,1,1,1,1,1,1,1,1,1,1,
1,1,1,1,1,1,1,6),(0.,0.0153846153846154,0.0307692307692308,0.0461538461538462,
0.0615384615384615,0.0769230769230769,0.0923076923076923,0.107692307692308,
0.123076923076923,0.138461538461538,0.153846153846154,0.169230769230769,
0.184615384615385,0.2,0.215384615384615,0.230769230769231,0.246153846153846,
0.261538461538462,0.276923076923077,0.292307692307692,0.307692307692308,
0.323076923076923,0.338461538461538,0.353846153846154,0.369230769230769,
0.384615384615385,0.4,0.415384615384615,0.430769230769231,0.446153846153846,
0.461538461538462,0.476923076923077,0.492307692307692,0.507692307692308,
0.523076923076923,0.538461538461538,0.553846153846154,0.569230769230769,
0.584615384615384,0.6,0.615384615384615,0.63076923076923,0.646153846153846,
0.661538461538461,0.676923076923076,0.692307692307692,0.707692307692307,
0.723076923076922,0.738461538461538,0.753846153846153,0.769230769230768,
0.784615384615384,0.799999999999999,0.815384615384614,0.83076923076923,
0.846153846153845,0.86153846153846,0.876923076923076,0.892307692307691,
0.907692307692306,0.923076923076922,0.938461538461537,0.953846153846152,
0.969230769230768,0.984615384615383,1.),.UNSPECIFIED.)
CURVE()
GEOMETRIC_REPRESENTATION_ITEM()
RATIONAL_B_SPLINE_CURVE((1.,1.,1.,1.,1.,1.,1.,1.,1.,1.,1.,1.,1.,1.,1.,1.,
1.,1.,1.,1.,1.,1.,1.,1.,1.,1.,1.,1.,1.,1.,1.,1.,1.,1.,1.,1.,1.,1.,1.,1.,
1.,1.,1.,1.,1.,1.,1.,1.,1.,1.,1.,1.,1.,1.,1.,1.,1.,1.,1.,1.,1.,1.,1.,1.,
1.,1.,1.,1.,1.,1.))
REPRESENTATION_ITEM('')
);
#151=(
BOUNDED_CURVE()
B_SPLINE_CURVE(5,(#23710,#23711,#23712,#23713,#23714,#23715,#23716,#23717,
#23718,#23719,#23720,#23721,#23722,#23723,#23724,#23725,#23726,#23727,#23728,
#23729,#23730,#23731,#23732,#23733,#23734,#23735,#23736,#23737,#23738,#23739,
#23740,#23741,#23742,#23743,#23744,#23745,#23746,#23747,#23748,#23749,#23750,
#23751,#23752,#23753,#23754,#23755,#23756,#23757,#23758,#23759,#23760,#23761,
#23762,#23763,#23764,#23765,#23766,#23767,#23768,#23769,#23770,#23771,#23772,
#23773,#23774,#23775,#23776,#23777,#23778,#23779),.UNSPECIFIED.,.F.,.F.)
B_SPLINE_CURVE_WITH_KNOTS((6,1,1,1,1,1,1,1,1,1,1,1,1,1,1,1,1,1,1,1,1,1,
1,1,1,1,1,1,1,1,1,1,1,1,1,1,1,1,1,1,1,1,1,1,1,1,1,1,1,1,1,1,1,1,1,1,1,1,
1,1,1,1,1,1,1,6),(0.,0.0153846153846154,0.0307692307692308,0.0461538461538462,
0.0615384615384615,0.0769230769230769,0.0923076923076923,0.107692307692308,
0.123076923076923,0.138461538461538,0.153846153846154,0.169230769230769,
0.184615384615385,0.2,0.215384615384615,0.230769230769231,0.246153846153846,
0.261538461538462,0.276923076923077,0.292307692307692,0.307692307692308,
0.323076923076923,0.338461538461538,0.353846153846154,0.369230769230769,
0.384615384615385,0.4,0.415384615384615,0.430769230769231,0.446153846153846,
0.461538461538462,0.476923076923077,0.492307692307692,0.507692307692308,
0.523076923076923,0.538461538461538,0.553846153846154,0.569230769230769,
0.584615384615384,0.6,0.615384615384615,0.63076923076923,0.646153846153846,
0.661538461538461,0.676923076923076,0.692307692307692,0.707692307692307,
0.723076923076922,0.738461538461538,0.753846153846153,0.769230769230768,
0.784615384615384,0.799999999999999,0.815384615384614,0.83076923076923,
0.846153846153845,0.86153846153846,0.876923076923076,0.892307692307691,
0.907692307692306,0.923076923076922,0.938461538461537,0.953846153846152,
0.969230769230768,0.984615384615383,1.),.UNSPECIFIED.)
CURVE()
GEOMETRIC_REPRESENTATION_ITEM()
RATIONAL_B_SPLINE_CURVE((1.,1.,1.,1.,1.,1.,1.,1.,1.,1.,1.,1.,1.,1.,1.,1.,
1.,1.,1.,1.,1.,1.,1.,1.,1.,1.,1.,1.,1.,1.,1.,1.,1.,1.,1.,1.,1.,1.,1.,1.,
1.,1.,1.,1.,1.,1.,1.,1.,1.,1.,1.,1.,1.,1.,1.,1.,1.,1.,1.,1.,1.,1.,1.,1.,
1.,1.,1.,1.,1.,1.))
REPRESENTATION_ITEM('')
);
#152=(
BOUNDED_CURVE()
B_SPLINE_CURVE(5,(#23783,#23784,#23785,#23786,#23787,#23788,#23789,#23790,
#23791,#23792,#23793,#23794,#23795,#23796,#23797,#23798,#23799,#23800,#23801,
#23802,#23803,#23804,#23805,#23806,#23807,#23808,#23809,#23810,#23811,#23812,
#23813,#23814,#23815,#23816,#23817,#23818,#23819,#23820,#23821,#23822,#23823,
#23824,#23825,#23826,#23827,#23828,#23829,#23830,#23831,#23832,#23833,#23834,
#23835,#23836,#23837,#23838,#23839,#23840,#23841,#23842,#23843,#23844,#23845,
#23846,#23847,#23848,#23849,#23850,#23851,#23852),.UNSPECIFIED.,.F.,.F.)
B_SPLINE_CURVE_WITH_KNOTS((6,1,1,1,1,1,1,1,1,1,1,1,1,1,1,1,1,1,1,1,1,1,
1,1,1,1,1,1,1,1,1,1,1,1,1,1,1,1,1,1,1,1,1,1,1,1,1,1,1,1,1,1,1,1,1,1,1,1,
1,1,1,1,1,1,1,6),(0.,0.0153846153846154,0.0307692307692308,0.0461538461538462,
0.0615384615384615,0.0769230769230769,0.0923076923076923,0.107692307692308,
0.123076923076923,0.138461538461538,0.153846153846154,0.169230769230769,
0.184615384615385,0.2,0.215384615384615,0.230769230769231,0.246153846153846,
0.261538461538462,0.276923076923077,0.292307692307692,0.307692307692308,
0.323076923076923,0.338461538461538,0.353846153846154,0.369230769230769,
0.384615384615385,0.4,0.415384615384615,0.430769230769231,0.446153846153846,
0.461538461538462,0.476923076923077,0.492307692307692,0.507692307692308,
0.523076923076923,0.538461538461538,0.553846153846154,0.569230769230769,
0.584615384615384,0.6,0.615384615384615,0.63076923076923,0.646153846153846,
0.661538461538461,0.676923076923076,0.692307692307692,0.707692307692307,
0.723076923076922,0.738461538461538,0.753846153846153,0.769230769230768,
0.784615384615384,0.799999999999999,0.815384615384614,0.83076923076923,
0.846153846153845,0.86153846153846,0.876923076923076,0.892307692307691,
0.907692307692306,0.923076923076922,0.938461538461537,0.953846153846152,
0.969230769230768,0.984615384615383,1.),.UNSPECIFIED.)
CURVE()
GEOMETRIC_REPRESENTATION_ITEM()
RATIONAL_B_SPLINE_CURVE((1.,1.,1.,1.,1.,1.,1.,1.,1.,1.,1.,1.,1.,1.,1.,1.,
1.,1.,1.,1.,1.,1.,1.,1.,1.,1.,1.,1.,1.,1.,1.,1.,1.,1.,1.,1.,1.,1.,1.,1.,
1.,1.,1.,1.,1.,1.,1.,1.,1.,1.,1.,1.,1.,1.,1.,1.,1.,1.,1.,1.,1.,1.,1.,1.,
1.,1.,1.,1.,1.,1.))
REPRESENTATION_ITEM('')
);
#153=(
BOUNDED_CURVE()
B_SPLINE_CURVE(5,(#23856,#23857,#23858,#23859,#23860,#23861,#23862,#23863,
#23864,#23865,#23866,#23867,#23868,#23869,#23870,#23871,#23872,#23873,#23874,
#23875,#23876,#23877,#23878,#23879,#23880,#23881,#23882,#23883,#23884,#23885,
#23886,#23887,#23888,#23889,#23890,#23891,#23892,#23893,#23894,#23895,#23896,
#23897,#23898,#23899,#23900,#23901,#23902,#23903,#23904,#23905,#23906,#23907,
#23908,#23909,#23910,#23911,#23912,#23913,#23914,#23915,#23916,#23917,#23918,
#23919,#23920,#23921,#23922,#23923,#23924,#23925),.UNSPECIFIED.,.F.,.F.)
B_SPLINE_CURVE_WITH_KNOTS((6,1,1,1,1,1,1,1,1,1,1,1,1,1,1,1,1,1,1,1,1,1,
1,1,1,1,1,1,1,1,1,1,1,1,1,1,1,1,1,1,1,1,1,1,1,1,1,1,1,1,1,1,1,1,1,1,1,1,
1,1,1,1,1,1,1,6),(0.,0.0153846153846154,0.0307692307692308,0.0461538461538462,
0.0615384615384615,0.0769230769230769,0.0923076923076923,0.107692307692308,
0.123076923076923,0.138461538461538,0.153846153846154,0.169230769230769,
0.184615384615385,0.2,0.215384615384615,0.230769230769231,0.246153846153846,
0.261538461538462,0.276923076923077,0.292307692307692,0.307692307692308,
0.323076923076923,0.338461538461538,0.353846153846154,0.369230769230769,
0.384615384615385,0.4,0.415384615384615,0.430769230769231,0.446153846153846,
0.461538461538462,0.476923076923077,0.492307692307692,0.507692307692308,
0.523076923076923,0.538461538461538,0.553846153846154,0.569230769230769,
0.584615384615384,0.6,0.615384615384615,0.63076923076923,0.646153846153846,
0.661538461538461,0.676923076923076,0.692307692307692,0.707692307692307,
0.723076923076922,0.738461538461538,0.753846153846153,0.769230769230768,
0.784615384615384,0.799999999999999,0.815384615384614,0.83076923076923,
0.846153846153845,0.86153846153846,0.876923076923076,0.892307692307691,
0.907692307692306,0.923076923076922,0.938461538461537,0.953846153846152,
0.969230769230768,0.984615384615383,1.),.UNSPECIFIED.)
CURVE()
GEOMETRIC_REPRESENTATION_ITEM()
RATIONAL_B_SPLINE_CURVE((1.,1.,1.,1.,1.,1.,1.,1.,1.,1.,1.,1.,1.,1.,1.,1.,
1.,1.,1.,1.,1.,1.,1.,1.,1.,1.,1.,1.,1.,1.,1.,1.,1.,1.,1.,1.,1.,1.,1.,1.,
1.,1.,1.,1.,1.,1.,1.,1.,1.,1.,1.,1.,1.,1.,1.,1.,1.,1.,1.,1.,1.,1.,1.,1.,
1.,1.,1.,1.,1.,1.))
REPRESENTATION_ITEM('')
);
#154=(
BOUNDED_CURVE()
B_SPLINE_CURVE(5,(#23929,#23930,#23931,#23932,#23933,#23934,#23935,#23936,
#23937,#23938,#23939,#23940,#23941,#23942,#23943,#23944,#23945,#23946,#23947,
#23948,#23949,#23950,#23951,#23952,#23953,#23954,#23955,#23956,#23957,#23958,
#23959,#23960,#23961,#23962,#23963,#23964,#23965,#23966,#23967,#23968,#23969,
#23970,#23971,#23972,#23973,#23974,#23975,#23976,#23977,#23978,#23979,#23980,
#23981,#23982,#23983,#23984,#23985,#23986,#23987,#23988,#23989,#23990,#23991,
#23992,#23993,#23994,#23995,#23996,#23997,#23998),.UNSPECIFIED.,.F.,.F.)
B_SPLINE_CURVE_WITH_KNOTS((6,1,1,1,1,1,1,1,1,1,1,1,1,1,1,1,1,1,1,1,1,1,
1,1,1,1,1,1,1,1,1,1,1,1,1,1,1,1,1,1,1,1,1,1,1,1,1,1,1,1,1,1,1,1,1,1,1,1,
1,1,1,1,1,1,1,6),(0.,0.0153846153846154,0.0307692307692308,0.0461538461538462,
0.0615384615384615,0.0769230769230769,0.0923076923076923,0.107692307692308,
0.123076923076923,0.138461538461538,0.153846153846154,0.169230769230769,
0.184615384615385,0.2,0.215384615384615,0.230769230769231,0.246153846153846,
0.261538461538462,0.276923076923077,0.292307692307692,0.307692307692308,
0.323076923076923,0.338461538461538,0.353846153846154,0.369230769230769,
0.384615384615385,0.4,0.415384615384615,0.430769230769231,0.446153846153846,
0.461538461538462,0.476923076923077,0.492307692307692,0.507692307692308,
0.523076923076923,0.538461538461538,0.553846153846154,0.569230769230769,
0.584615384615384,0.6,0.615384615384615,0.63076923076923,0.646153846153846,
0.661538461538461,0.676923076923076,0.692307692307692,0.707692307692307,
0.723076923076922,0.738461538461538,0.753846153846153,0.769230769230768,
0.784615384615384,0.799999999999999,0.815384615384614,0.83076923076923,
0.846153846153845,0.86153846153846,0.876923076923076,0.892307692307691,
0.907692307692306,0.923076923076922,0.938461538461537,0.953846153846152,
0.969230769230768,0.984615384615383,1.),.UNSPECIFIED.)
CURVE()
GEOMETRIC_REPRESENTATION_ITEM()
RATIONAL_B_SPLINE_CURVE((1.,1.,1.,1.,1.,1.,1.,1.,1.,1.,1.,1.,1.,1.,1.,1.,
1.,1.,1.,1.,1.,1.,1.,1.,1.,1.,1.,1.,1.,1.,1.,1.,1.,1.,1.,1.,1.,1.,1.,1.,
1.,1.,1.,1.,1.,1.,1.,1.,1.,1.,1.,1.,1.,1.,1.,1.,1.,1.,1.,1.,1.,1.,1.,1.,
1.,1.,1.,1.,1.,1.))
REPRESENTATION_ITEM('')
);
#155=(
BOUNDED_CURVE()
B_SPLINE_CURVE(5,(#24002,#24003,#24004,#24005,#24006,#24007,#24008,#24009,
#24010,#24011,#24012,#24013,#24014,#24015,#24016,#24017,#24018,#24019,#24020,
#24021,#24022,#24023,#24024,#24025,#24026,#24027,#24028,#24029,#24030,#24031,
#24032,#24033,#24034,#24035,#24036,#24037,#24038,#24039,#24040,#24041,#24042,
#24043,#24044,#24045,#24046,#24047,#24048,#24049,#24050,#24051,#24052,#24053,
#24054,#24055,#24056,#24057,#24058,#24059,#24060,#24061,#24062,#24063,#24064,
#24065,#24066,#24067,#24068,#24069,#24070,#24071),.UNSPECIFIED.,.F.,.F.)
B_SPLINE_CURVE_WITH_KNOTS((6,1,1,1,1,1,1,1,1,1,1,1,1,1,1,1,1,1,1,1,1,1,
1,1,1,1,1,1,1,1,1,1,1,1,1,1,1,1,1,1,1,1,1,1,1,1,1,1,1,1,1,1,1,1,1,1,1,1,
1,1,1,1,1,1,1,6),(0.,0.0153846153846154,0.0307692307692308,0.0461538461538462,
0.0615384615384615,0.0769230769230769,0.0923076923076923,0.107692307692308,
0.123076923076923,0.138461538461538,0.153846153846154,0.169230769230769,
0.184615384615385,0.2,0.215384615384615,0.230769230769231,0.246153846153846,
0.261538461538462,0.276923076923077,0.292307692307692,0.307692307692308,
0.323076923076923,0.338461538461538,0.353846153846154,0.369230769230769,
0.384615384615385,0.4,0.415384615384615,0.430769230769231,0.446153846153846,
0.461538461538462,0.476923076923077,0.492307692307692,0.507692307692308,
0.523076923076923,0.538461538461538,0.553846153846154,0.569230769230769,
0.584615384615384,0.6,0.615384615384615,0.63076923076923,0.646153846153846,
0.661538461538461,0.676923076923076,0.692307692307692,0.707692307692307,
0.723076923076922,0.738461538461538,0.753846153846153,0.769230769230768,
0.784615384615384,0.799999999999999,0.815384615384614,0.83076923076923,
0.846153846153845,0.86153846153846,0.876923076923076,0.892307692307691,
0.907692307692306,0.923076923076922,0.938461538461537,0.953846153846152,
0.969230769230768,0.984615384615383,1.),.UNSPECIFIED.)
CURVE()
GEOMETRIC_REPRESENTATION_ITEM()
RATIONAL_B_SPLINE_CURVE((1.,1.,1.,1.,1.,1.,1.,1.,1.,1.,1.,1.,1.,1.,1.,1.,
1.,1.,1.,1.,1.,1.,1.,1.,1.,1.,1.,1.,1.,1.,1.,1.,1.,1.,1.,1.,1.,1.,1.,1.,
1.,1.,1.,1.,1.,1.,1.,1.,1.,1.,1.,1.,1.,1.,1.,1.,1.,1.,1.,1.,1.,1.,1.,1.,
1.,1.,1.,1.,1.,1.))
REPRESENTATION_ITEM('')
);
#156=(
BOUNDED_CURVE()
B_SPLINE_CURVE(5,(#24075,#24076,#24077,#24078,#24079,#24080,#24081,#24082,
#24083,#24084,#24085,#24086,#24087,#24088,#24089,#24090,#24091,#24092,#24093,
#24094,#24095,#24096,#24097,#24098,#24099,#24100,#24101,#24102,#24103,#24104,
#24105,#24106,#24107,#24108,#24109,#24110,#24111,#24112,#24113,#24114,#24115,
#24116,#24117,#24118,#24119,#24120,#24121,#24122,#24123,#24124,#24125,#24126,
#24127,#24128,#24129,#24130,#24131,#24132,#24133,#24134,#24135,#24136,#24137,
#24138,#24139,#24140,#24141,#24142,#24143,#24144),.UNSPECIFIED.,.F.,.F.)
B_SPLINE_CURVE_WITH_KNOTS((6,1,1,1,1,1,1,1,1,1,1,1,1,1,1,1,1,1,1,1,1,1,
1,1,1,1,1,1,1,1,1,1,1,1,1,1,1,1,1,1,1,1,1,1,1,1,1,1,1,1,1,1,1,1,1,1,1,1,
1,1,1,1,1,1,1,6),(0.,0.0153846153846154,0.0307692307692308,0.0461538461538462,
0.0615384615384615,0.0769230769230769,0.0923076923076923,0.107692307692308,
0.123076923076923,0.138461538461538,0.153846153846154,0.169230769230769,
0.184615384615385,0.2,0.215384615384615,0.230769230769231,0.246153846153846,
0.261538461538462,0.276923076923077,0.292307692307692,0.307692307692308,
0.323076923076923,0.338461538461538,0.353846153846154,0.369230769230769,
0.384615384615385,0.4,0.415384615384615,0.430769230769231,0.446153846153846,
0.461538461538462,0.476923076923077,0.492307692307692,0.507692307692308,
0.523076923076923,0.538461538461538,0.553846153846154,0.569230769230769,
0.584615384615384,0.6,0.615384615384615,0.63076923076923,0.646153846153846,
0.661538461538461,0.676923076923076,0.692307692307692,0.707692307692307,
0.723076923076922,0.738461538461538,0.753846153846153,0.769230769230768,
0.784615384615384,0.799999999999999,0.815384615384614,0.83076923076923,
0.846153846153845,0.86153846153846,0.876923076923076,0.892307692307691,
0.907692307692306,0.923076923076922,0.938461538461537,0.953846153846152,
0.969230769230768,0.984615384615383,1.),.UNSPECIFIED.)
CURVE()
GEOMETRIC_REPRESENTATION_ITEM()
RATIONAL_B_SPLINE_CURVE((1.,1.,1.,1.,1.,1.,1.,1.,1.,1.,1.,1.,1.,1.,1.,1.,
1.,1.,1.,1.,1.,1.,1.,1.,1.,1.,1.,1.,1.,1.,1.,1.,1.,1.,1.,1.,1.,1.,1.,1.,
1.,1.,1.,1.,1.,1.,1.,1.,1.,1.,1.,1.,1.,1.,1.,1.,1.,1.,1.,1.,1.,1.,1.,1.,
1.,1.,1.,1.,1.,1.))
REPRESENTATION_ITEM('')
);
#157=(
BOUNDED_CURVE()
B_SPLINE_CURVE(5,(#24148,#24149,#24150,#24151,#24152,#24153,#24154,#24155,
#24156,#24157,#24158,#24159,#24160,#24161,#24162,#24163,#24164,#24165,#24166,
#24167,#24168,#24169,#24170,#24171,#24172,#24173,#24174,#24175,#24176,#24177,
#24178,#24179,#24180,#24181,#24182,#24183,#24184,#24185,#24186,#24187,#24188,
#24189,#24190,#24191,#24192,#24193,#24194,#24195,#24196,#24197,#24198,#24199,
#24200,#24201,#24202,#24203,#24204,#24205,#24206,#24207,#24208,#24209,#24210,
#24211,#24212,#24213,#24214,#24215,#24216,#24217),.UNSPECIFIED.,.F.,.F.)
B_SPLINE_CURVE_WITH_KNOTS((6,1,1,1,1,1,1,1,1,1,1,1,1,1,1,1,1,1,1,1,1,1,
1,1,1,1,1,1,1,1,1,1,1,1,1,1,1,1,1,1,1,1,1,1,1,1,1,1,1,1,1,1,1,1,1,1,1,1,
1,1,1,1,1,1,1,6),(0.,0.0153846153846154,0.0307692307692308,0.0461538461538462,
0.0615384615384615,0.0769230769230769,0.0923076923076923,0.107692307692308,
0.123076923076923,0.138461538461538,0.153846153846154,0.169230769230769,
0.184615384615385,0.2,0.215384615384615,0.230769230769231,0.246153846153846,
0.261538461538462,0.276923076923077,0.292307692307692,0.307692307692308,
0.323076923076923,0.338461538461538,0.353846153846154,0.369230769230769,
0.384615384615385,0.4,0.415384615384615,0.430769230769231,0.446153846153846,
0.461538461538462,0.476923076923077,0.492307692307692,0.507692307692308,
0.523076923076923,0.538461538461538,0.553846153846154,0.569230769230769,
0.584615384615384,0.6,0.615384615384615,0.63076923076923,0.646153846153846,
0.661538461538461,0.676923076923076,0.692307692307692,0.707692307692307,
0.723076923076922,0.738461538461538,0.753846153846153,0.769230769230768,
0.784615384615384,0.799999999999999,0.815384615384614,0.83076923076923,
0.846153846153845,0.86153846153846,0.876923076923076,0.892307692307691,
0.907692307692306,0.923076923076922,0.938461538461537,0.953846153846152,
0.969230769230768,0.984615384615383,1.),.UNSPECIFIED.)
CURVE()
GEOMETRIC_REPRESENTATION_ITEM()
RATIONAL_B_SPLINE_CURVE((1.,1.,1.,1.,1.,1.,1.,1.,1.,1.,1.,1.,1.,1.,1.,1.,
1.,1.,1.,1.,1.,1.,1.,1.,1.,1.,1.,1.,1.,1.,1.,1.,1.,1.,1.,1.,1.,1.,1.,1.,
1.,1.,1.,1.,1.,1.,1.,1.,1.,1.,1.,1.,1.,1.,1.,1.,1.,1.,1.,1.,1.,1.,1.,1.,
1.,1.,1.,1.,1.,1.))
REPRESENTATION_ITEM('')
);
#158=(
BOUNDED_CURVE()
B_SPLINE_CURVE(5,(#24221,#24222,#24223,#24224,#24225,#24226,#24227,#24228,
#24229,#24230,#24231,#24232,#24233,#24234,#24235,#24236,#24237,#24238,#24239,
#24240,#24241,#24242,#24243,#24244,#24245,#24246,#24247,#24248,#24249,#24250,
#24251,#24252,#24253,#24254,#24255,#24256,#24257,#24258,#24259,#24260,#24261,
#24262,#24263,#24264,#24265,#24266,#24267,#24268,#24269,#24270,#24271,#24272,
#24273,#24274,#24275,#24276,#24277,#24278,#24279,#24280,#24281,#24282,#24283,
#24284,#24285,#24286,#24287,#24288,#24289,#24290),.UNSPECIFIED.,.F.,.F.)
B_SPLINE_CURVE_WITH_KNOTS((6,1,1,1,1,1,1,1,1,1,1,1,1,1,1,1,1,1,1,1,1,1,
1,1,1,1,1,1,1,1,1,1,1,1,1,1,1,1,1,1,1,1,1,1,1,1,1,1,1,1,1,1,1,1,1,1,1,1,
1,1,1,1,1,1,1,6),(0.,0.0153846153846154,0.0307692307692308,0.0461538461538462,
0.0615384615384615,0.0769230769230769,0.0923076923076923,0.107692307692308,
0.123076923076923,0.138461538461538,0.153846153846154,0.169230769230769,
0.184615384615385,0.2,0.215384615384615,0.230769230769231,0.246153846153846,
0.261538461538462,0.276923076923077,0.292307692307692,0.307692307692308,
0.323076923076923,0.338461538461538,0.353846153846154,0.369230769230769,
0.384615384615385,0.4,0.415384615384615,0.430769230769231,0.446153846153846,
0.461538461538462,0.476923076923077,0.492307692307692,0.507692307692308,
0.523076923076923,0.538461538461538,0.553846153846154,0.569230769230769,
0.584615384615384,0.6,0.615384615384615,0.63076923076923,0.646153846153846,
0.661538461538461,0.676923076923076,0.692307692307692,0.707692307692307,
0.723076923076922,0.738461538461538,0.753846153846153,0.769230769230768,
0.784615384615384,0.799999999999999,0.815384615384614,0.83076923076923,
0.846153846153845,0.86153846153846,0.876923076923076,0.892307692307691,
0.907692307692306,0.923076923076922,0.938461538461537,0.953846153846152,
0.969230769230768,0.984615384615383,1.),.UNSPECIFIED.)
CURVE()
GEOMETRIC_REPRESENTATION_ITEM()
RATIONAL_B_SPLINE_CURVE((1.,1.,1.,1.,1.,1.,1.,1.,1.,1.,1.,1.,1.,1.,1.,1.,
1.,1.,1.,1.,1.,1.,1.,1.,1.,1.,1.,1.,1.,1.,1.,1.,1.,1.,1.,1.,1.,1.,1.,1.,
1.,1.,1.,1.,1.,1.,1.,1.,1.,1.,1.,1.,1.,1.,1.,1.,1.,1.,1.,1.,1.,1.,1.,1.,
1.,1.,1.,1.,1.,1.))
REPRESENTATION_ITEM('')
);
#159=(
BOUNDED_CURVE()
B_SPLINE_CURVE(5,(#24294,#24295,#24296,#24297,#24298,#24299,#24300,#24301,
#24302,#24303,#24304,#24305,#24306,#24307,#24308,#24309,#24310,#24311,#24312,
#24313,#24314,#24315,#24316,#24317,#24318,#24319,#24320,#24321,#24322,#24323,
#24324,#24325,#24326,#24327,#24328,#24329,#24330,#24331,#24332,#24333,#24334,
#24335,#24336,#24337,#24338,#24339,#24340,#24341,#24342,#24343,#24344,#24345,
#24346,#24347,#24348,#24349,#24350,#24351,#24352,#24353,#24354,#24355,#24356,
#24357,#24358,#24359,#24360,#24361,#24362,#24363),.UNSPECIFIED.,.F.,.F.)
B_SPLINE_CURVE_WITH_KNOTS((6,1,1,1,1,1,1,1,1,1,1,1,1,1,1,1,1,1,1,1,1,1,
1,1,1,1,1,1,1,1,1,1,1,1,1,1,1,1,1,1,1,1,1,1,1,1,1,1,1,1,1,1,1,1,1,1,1,1,
1,1,1,1,1,1,1,6),(0.,0.0153846153846154,0.0307692307692308,0.0461538461538462,
0.0615384615384615,0.0769230769230769,0.0923076923076923,0.107692307692308,
0.123076923076923,0.138461538461538,0.153846153846154,0.169230769230769,
0.184615384615385,0.2,0.215384615384615,0.230769230769231,0.246153846153846,
0.261538461538462,0.276923076923077,0.292307692307692,0.307692307692308,
0.323076923076923,0.338461538461538,0.353846153846154,0.369230769230769,
0.384615384615385,0.4,0.415384615384615,0.430769230769231,0.446153846153846,
0.461538461538462,0.476923076923077,0.492307692307692,0.507692307692308,
0.523076923076923,0.538461538461538,0.553846153846154,0.569230769230769,
0.584615384615384,0.6,0.615384615384615,0.63076923076923,0.646153846153846,
0.661538461538461,0.676923076923076,0.692307692307692,0.707692307692307,
0.723076923076922,0.738461538461538,0.753846153846153,0.769230769230768,
0.784615384615384,0.799999999999999,0.815384615384614,0.83076923076923,
0.846153846153845,0.86153846153846,0.876923076923076,0.892307692307691,
0.907692307692306,0.923076923076922,0.938461538461537,0.953846153846152,
0.969230769230768,0.984615384615383,1.),.UNSPECIFIED.)
CURVE()
GEOMETRIC_REPRESENTATION_ITEM()
RATIONAL_B_SPLINE_CURVE((1.,1.,1.,1.,1.,1.,1.,1.,1.,1.,1.,1.,1.,1.,1.,1.,
1.,1.,1.,1.,1.,1.,1.,1.,1.,1.,1.,1.,1.,1.,1.,1.,1.,1.,1.,1.,1.,1.,1.,1.,
1.,1.,1.,1.,1.,1.,1.,1.,1.,1.,1.,1.,1.,1.,1.,1.,1.,1.,1.,1.,1.,1.,1.,1.,
1.,1.,1.,1.,1.,1.))
REPRESENTATION_ITEM('')
);
#160=(
BOUNDED_CURVE()
B_SPLINE_CURVE(5,(#24367,#24368,#24369,#24370,#24371,#24372,#24373,#24374,
#24375,#24376,#24377,#24378,#24379,#24380,#24381,#24382,#24383,#24384,#24385,
#24386,#24387,#24388,#24389,#24390,#24391,#24392,#24393,#24394,#24395,#24396,
#24397,#24398,#24399,#24400,#24401,#24402,#24403,#24404,#24405,#24406,#24407,
#24408,#24409,#24410,#24411,#24412,#24413,#24414,#24415,#24416,#24417,#24418,
#24419,#24420,#24421,#24422,#24423,#24424,#24425,#24426,#24427,#24428,#24429,
#24430,#24431,#24432,#24433,#24434,#24435,#24436),.UNSPECIFIED.,.F.,.F.)
B_SPLINE_CURVE_WITH_KNOTS((6,1,1,1,1,1,1,1,1,1,1,1,1,1,1,1,1,1,1,1,1,1,
1,1,1,1,1,1,1,1,1,1,1,1,1,1,1,1,1,1,1,1,1,1,1,1,1,1,1,1,1,1,1,1,1,1,1,1,
1,1,1,1,1,1,1,6),(0.,0.0153846153846154,0.0307692307692308,0.0461538461538462,
0.0615384615384615,0.0769230769230769,0.0923076923076923,0.107692307692308,
0.123076923076923,0.138461538461538,0.153846153846154,0.169230769230769,
0.184615384615385,0.2,0.215384615384615,0.230769230769231,0.246153846153846,
0.261538461538462,0.276923076923077,0.292307692307692,0.307692307692308,
0.323076923076923,0.338461538461538,0.353846153846154,0.369230769230769,
0.384615384615385,0.4,0.415384615384615,0.430769230769231,0.446153846153846,
0.461538461538462,0.476923076923077,0.492307692307692,0.507692307692308,
0.523076923076923,0.538461538461538,0.553846153846154,0.569230769230769,
0.584615384615384,0.6,0.615384615384615,0.63076923076923,0.646153846153846,
0.661538461538461,0.676923076923076,0.692307692307692,0.707692307692307,
0.723076923076922,0.738461538461538,0.753846153846153,0.769230769230768,
0.784615384615384,0.799999999999999,0.815384615384614,0.83076923076923,
0.846153846153845,0.86153846153846,0.876923076923076,0.892307692307691,
0.907692307692306,0.923076923076922,0.938461538461537,0.953846153846152,
0.969230769230768,0.984615384615383,1.),.UNSPECIFIED.)
CURVE()
GEOMETRIC_REPRESENTATION_ITEM()
RATIONAL_B_SPLINE_CURVE((1.,1.,1.,1.,1.,1.,1.,1.,1.,1.,1.,1.,1.,1.,1.,1.,
1.,1.,1.,1.,1.,1.,1.,1.,1.,1.,1.,1.,1.,1.,1.,1.,1.,1.,1.,1.,1.,1.,1.,1.,
1.,1.,1.,1.,1.,1.,1.,1.,1.,1.,1.,1.,1.,1.,1.,1.,1.,1.,1.,1.,1.,1.,1.,1.,
1.,1.,1.,1.,1.,1.))
REPRESENTATION_ITEM('')
);
#161=(
BOUNDED_CURVE()
B_SPLINE_CURVE(5,(#24440,#24441,#24442,#24443,#24444,#24445,#24446,#24447,
#24448,#24449,#24450,#24451,#24452,#24453,#24454,#24455,#24456,#24457,#24458,
#24459,#24460,#24461,#24462,#24463,#24464,#24465,#24466,#24467,#24468,#24469,
#24470,#24471,#24472,#24473,#24474,#24475,#24476,#24477,#24478,#24479,#24480,
#24481,#24482,#24483,#24484,#24485,#24486,#24487,#24488,#24489,#24490,#24491,
#24492,#24493,#24494,#24495,#24496,#24497,#24498,#24499,#24500,#24501,#24502,
#24503,#24504,#24505,#24506,#24507,#24508,#24509),.UNSPECIFIED.,.F.,.F.)
B_SPLINE_CURVE_WITH_KNOTS((6,1,1,1,1,1,1,1,1,1,1,1,1,1,1,1,1,1,1,1,1,1,
1,1,1,1,1,1,1,1,1,1,1,1,1,1,1,1,1,1,1,1,1,1,1,1,1,1,1,1,1,1,1,1,1,1,1,1,
1,1,1,1,1,1,1,6),(0.,0.0153846153846154,0.0307692307692308,0.0461538461538462,
0.0615384615384615,0.0769230769230769,0.0923076923076923,0.107692307692308,
0.123076923076923,0.138461538461538,0.153846153846154,0.169230769230769,
0.184615384615385,0.2,0.215384615384615,0.230769230769231,0.246153846153846,
0.261538461538462,0.276923076923077,0.292307692307692,0.307692307692308,
0.323076923076923,0.338461538461538,0.353846153846154,0.369230769230769,
0.384615384615385,0.4,0.415384615384615,0.430769230769231,0.446153846153846,
0.461538461538462,0.476923076923077,0.492307692307692,0.507692307692308,
0.523076923076923,0.538461538461538,0.553846153846154,0.569230769230769,
0.584615384615384,0.6,0.615384615384615,0.63076923076923,0.646153846153846,
0.661538461538461,0.676923076923076,0.692307692307692,0.707692307692307,
0.723076923076922,0.738461538461538,0.753846153846153,0.769230769230768,
0.784615384615384,0.799999999999999,0.815384615384614,0.83076923076923,
0.846153846153845,0.86153846153846,0.876923076923076,0.892307692307691,
0.907692307692306,0.923076923076922,0.938461538461537,0.953846153846152,
0.969230769230768,0.984615384615383,1.),.UNSPECIFIED.)
CURVE()
GEOMETRIC_REPRESENTATION_ITEM()
RATIONAL_B_SPLINE_CURVE((1.,1.,1.,1.,1.,1.,1.,1.,1.,1.,1.,1.,1.,1.,1.,1.,
1.,1.,1.,1.,1.,1.,1.,1.,1.,1.,1.,1.,1.,1.,1.,1.,1.,1.,1.,1.,1.,1.,1.,1.,
1.,1.,1.,1.,1.,1.,1.,1.,1.,1.,1.,1.,1.,1.,1.,1.,1.,1.,1.,1.,1.,1.,1.,1.,
1.,1.,1.,1.,1.,1.))
REPRESENTATION_ITEM('')
);
#162=(
BOUNDED_CURVE()
B_SPLINE_CURVE(5,(#24513,#24514,#24515,#24516,#24517,#24518,#24519,#24520,
#24521,#24522,#24523,#24524,#24525,#24526,#24527,#24528,#24529,#24530,#24531,
#24532,#24533,#24534,#24535,#24536,#24537,#24538,#24539,#24540,#24541,#24542,
#24543,#24544,#24545,#24546,#24547,#24548,#24549,#24550,#24551,#24552,#24553,
#24554,#24555,#24556,#24557,#24558,#24559,#24560,#24561,#24562,#24563,#24564,
#24565,#24566,#24567,#24568,#24569,#24570,#24571,#24572,#24573,#24574,#24575,
#24576,#24577,#24578,#24579,#24580,#24581,#24582),.UNSPECIFIED.,.F.,.F.)
B_SPLINE_CURVE_WITH_KNOTS((6,1,1,1,1,1,1,1,1,1,1,1,1,1,1,1,1,1,1,1,1,1,
1,1,1,1,1,1,1,1,1,1,1,1,1,1,1,1,1,1,1,1,1,1,1,1,1,1,1,1,1,1,1,1,1,1,1,1,
1,1,1,1,1,1,1,6),(0.,0.0153846153846154,0.0307692307692308,0.0461538461538462,
0.0615384615384615,0.0769230769230769,0.0923076923076923,0.107692307692308,
0.123076923076923,0.138461538461538,0.153846153846154,0.169230769230769,
0.184615384615385,0.2,0.215384615384615,0.230769230769231,0.246153846153846,
0.261538461538462,0.276923076923077,0.292307692307692,0.307692307692308,
0.323076923076923,0.338461538461538,0.353846153846154,0.369230769230769,
0.384615384615385,0.4,0.415384615384615,0.430769230769231,0.446153846153846,
0.461538461538462,0.476923076923077,0.492307692307692,0.507692307692308,
0.523076923076923,0.538461538461538,0.553846153846154,0.569230769230769,
0.584615384615384,0.6,0.615384615384615,0.63076923076923,0.646153846153846,
0.661538461538461,0.676923076923076,0.692307692307692,0.707692307692307,
0.723076923076922,0.738461538461538,0.753846153846153,0.769230769230768,
0.784615384615384,0.799999999999999,0.815384615384614,0.83076923076923,
0.846153846153845,0.86153846153846,0.876923076923076,0.892307692307691,
0.907692307692306,0.923076923076922,0.938461538461537,0.953846153846152,
0.969230769230768,0.984615384615383,1.),.UNSPECIFIED.)
CURVE()
GEOMETRIC_REPRESENTATION_ITEM()
RATIONAL_B_SPLINE_CURVE((1.,1.,1.,1.,1.,1.,1.,1.,1.,1.,1.,1.,1.,1.,1.,1.,
1.,1.,1.,1.,1.,1.,1.,1.,1.,1.,1.,1.,1.,1.,1.,1.,1.,1.,1.,1.,1.,1.,1.,1.,
1.,1.,1.,1.,1.,1.,1.,1.,1.,1.,1.,1.,1.,1.,1.,1.,1.,1.,1.,1.,1.,1.,1.,1.,
1.,1.,1.,1.,1.,1.))
REPRESENTATION_ITEM('')
);
#163=(
BOUNDED_CURVE()
B_SPLINE_CURVE(5,(#24586,#24587,#24588,#24589,#24590,#24591,#24592,#24593,
#24594,#24595,#24596,#24597,#24598,#24599,#24600,#24601,#24602,#24603,#24604,
#24605,#24606,#24607,#24608,#24609,#24610,#24611,#24612,#24613,#24614,#24615,
#24616,#24617,#24618,#24619,#24620,#24621,#24622,#24623,#24624,#24625,#24626,
#24627,#24628,#24629,#24630,#24631,#24632,#24633,#24634,#24635,#24636,#24637,
#24638,#24639,#24640,#24641,#24642,#24643,#24644,#24645,#24646,#24647,#24648,
#24649,#24650,#24651,#24652,#24653,#24654,#24655),.UNSPECIFIED.,.F.,.F.)
B_SPLINE_CURVE_WITH_KNOTS((6,1,1,1,1,1,1,1,1,1,1,1,1,1,1,1,1,1,1,1,1,1,
1,1,1,1,1,1,1,1,1,1,1,1,1,1,1,1,1,1,1,1,1,1,1,1,1,1,1,1,1,1,1,1,1,1,1,1,
1,1,1,1,1,1,1,6),(0.,0.0153846153846154,0.0307692307692308,0.0461538461538462,
0.0615384615384615,0.0769230769230769,0.0923076923076923,0.107692307692308,
0.123076923076923,0.138461538461538,0.153846153846154,0.169230769230769,
0.184615384615385,0.2,0.215384615384615,0.230769230769231,0.246153846153846,
0.261538461538462,0.276923076923077,0.292307692307692,0.307692307692308,
0.323076923076923,0.338461538461538,0.353846153846154,0.369230769230769,
0.384615384615385,0.4,0.415384615384615,0.430769230769231,0.446153846153846,
0.461538461538462,0.476923076923077,0.492307692307692,0.507692307692308,
0.523076923076923,0.538461538461538,0.553846153846154,0.569230769230769,
0.584615384615384,0.6,0.615384615384615,0.63076923076923,0.646153846153846,
0.661538461538461,0.676923076923076,0.692307692307692,0.707692307692307,
0.723076923076922,0.738461538461538,0.753846153846153,0.769230769230768,
0.784615384615384,0.799999999999999,0.815384615384614,0.83076923076923,
0.846153846153845,0.86153846153846,0.876923076923076,0.892307692307691,
0.907692307692306,0.923076923076922,0.938461538461537,0.953846153846152,
0.969230769230768,0.984615384615383,1.),.UNSPECIFIED.)
CURVE()
GEOMETRIC_REPRESENTATION_ITEM()
RATIONAL_B_SPLINE_CURVE((1.,1.,1.,1.,1.,1.,1.,1.,1.,1.,1.,1.,1.,1.,1.,1.,
1.,1.,1.,1.,1.,1.,1.,1.,1.,1.,1.,1.,1.,1.,1.,1.,1.,1.,1.,1.,1.,1.,1.,1.,
1.,1.,1.,1.,1.,1.,1.,1.,1.,1.,1.,1.,1.,1.,1.,1.,1.,1.,1.,1.,1.,1.,1.,1.,
1.,1.,1.,1.,1.,1.))
REPRESENTATION_ITEM('')
);
#164=(
BOUNDED_CURVE()
B_SPLINE_CURVE(5,(#24659,#24660,#24661,#24662,#24663,#24664,#24665,#24666,
#24667,#24668,#24669,#24670,#24671,#24672,#24673,#24674,#24675,#24676,#24677,
#24678,#24679,#24680,#24681,#24682,#24683,#24684,#24685,#24686,#24687,#24688,
#24689,#24690,#24691,#24692,#24693,#24694,#24695,#24696,#24697,#24698,#24699,
#24700,#24701,#24702,#24703,#24704,#24705,#24706,#24707,#24708,#24709,#24710,
#24711,#24712,#24713,#24714,#24715,#24716,#24717,#24718,#24719,#24720,#24721,
#24722,#24723,#24724,#24725,#24726,#24727,#24728),.UNSPECIFIED.,.F.,.F.)
B_SPLINE_CURVE_WITH_KNOTS((6,1,1,1,1,1,1,1,1,1,1,1,1,1,1,1,1,1,1,1,1,1,
1,1,1,1,1,1,1,1,1,1,1,1,1,1,1,1,1,1,1,1,1,1,1,1,1,1,1,1,1,1,1,1,1,1,1,1,
1,1,1,1,1,1,1,6),(0.,0.0153846153846154,0.0307692307692308,0.0461538461538462,
0.0615384615384615,0.0769230769230769,0.0923076923076923,0.107692307692308,
0.123076923076923,0.138461538461538,0.153846153846154,0.169230769230769,
0.184615384615385,0.2,0.215384615384615,0.230769230769231,0.246153846153846,
0.261538461538462,0.276923076923077,0.292307692307692,0.307692307692308,
0.323076923076923,0.338461538461538,0.353846153846154,0.369230769230769,
0.384615384615385,0.4,0.415384615384615,0.430769230769231,0.446153846153846,
0.461538461538462,0.476923076923077,0.492307692307692,0.507692307692308,
0.523076923076923,0.538461538461538,0.553846153846154,0.569230769230769,
0.584615384615384,0.6,0.615384615384615,0.63076923076923,0.646153846153846,
0.661538461538461,0.676923076923076,0.692307692307692,0.707692307692307,
0.723076923076922,0.738461538461538,0.753846153846153,0.769230769230768,
0.784615384615384,0.799999999999999,0.815384615384614,0.83076923076923,
0.846153846153845,0.86153846153846,0.876923076923076,0.892307692307691,
0.907692307692306,0.923076923076922,0.938461538461537,0.953846153846152,
0.969230769230768,0.984615384615383,1.),.UNSPECIFIED.)
CURVE()
GEOMETRIC_REPRESENTATION_ITEM()
RATIONAL_B_SPLINE_CURVE((1.,1.,1.,1.,1.,1.,1.,1.,1.,1.,1.,1.,1.,1.,1.,1.,
1.,1.,1.,1.,1.,1.,1.,1.,1.,1.,1.,1.,1.,1.,1.,1.,1.,1.,1.,1.,1.,1.,1.,1.,
1.,1.,1.,1.,1.,1.,1.,1.,1.,1.,1.,1.,1.,1.,1.,1.,1.,1.,1.,1.,1.,1.,1.,1.,
1.,1.,1.,1.,1.,1.))
REPRESENTATION_ITEM('')
);
#165=(
BOUNDED_CURVE()
B_SPLINE_CURVE(5,(#24732,#24733,#24734,#24735,#24736,#24737,#24738,#24739,
#24740,#24741,#24742,#24743,#24744,#24745,#24746,#24747,#24748,#24749,#24750,
#24751,#24752,#24753,#24754,#24755,#24756,#24757,#24758,#24759,#24760,#24761,
#24762,#24763,#24764,#24765,#24766,#24767,#24768,#24769,#24770,#24771,#24772,
#24773,#24774,#24775,#24776,#24777,#24778,#24779,#24780,#24781,#24782,#24783,
#24784,#24785,#24786,#24787,#24788,#24789,#24790,#24791,#24792,#24793,#24794,
#24795,#24796,#24797,#24798,#24799,#24800,#24801),.UNSPECIFIED.,.F.,.F.)
B_SPLINE_CURVE_WITH_KNOTS((6,1,1,1,1,1,1,1,1,1,1,1,1,1,1,1,1,1,1,1,1,1,
1,1,1,1,1,1,1,1,1,1,1,1,1,1,1,1,1,1,1,1,1,1,1,1,1,1,1,1,1,1,1,1,1,1,1,1,
1,1,1,1,1,1,1,6),(0.,0.0153846153846154,0.0307692307692308,0.0461538461538462,
0.0615384615384615,0.0769230769230769,0.0923076923076923,0.107692307692308,
0.123076923076923,0.138461538461538,0.153846153846154,0.169230769230769,
0.184615384615385,0.2,0.215384615384615,0.230769230769231,0.246153846153846,
0.261538461538462,0.276923076923077,0.292307692307692,0.307692307692308,
0.323076923076923,0.338461538461538,0.353846153846154,0.369230769230769,
0.384615384615385,0.4,0.415384615384615,0.430769230769231,0.446153846153846,
0.461538461538462,0.476923076923077,0.492307692307692,0.507692307692308,
0.523076923076923,0.538461538461538,0.553846153846154,0.569230769230769,
0.584615384615384,0.6,0.615384615384615,0.63076923076923,0.646153846153846,
0.661538461538461,0.676923076923076,0.692307692307692,0.707692307692307,
0.723076923076922,0.738461538461538,0.753846153846153,0.769230769230768,
0.784615384615384,0.799999999999999,0.815384615384614,0.83076923076923,
0.846153846153845,0.86153846153846,0.876923076923076,0.892307692307691,
0.907692307692306,0.923076923076922,0.938461538461537,0.953846153846152,
0.969230769230768,0.984615384615383,1.),.UNSPECIFIED.)
CURVE()
GEOMETRIC_REPRESENTATION_ITEM()
RATIONAL_B_SPLINE_CURVE((1.,1.,1.,1.,1.,1.,1.,1.,1.,1.,1.,1.,1.,1.,1.,1.,
1.,1.,1.,1.,1.,1.,1.,1.,1.,1.,1.,1.,1.,1.,1.,1.,1.,1.,1.,1.,1.,1.,1.,1.,
1.,1.,1.,1.,1.,1.,1.,1.,1.,1.,1.,1.,1.,1.,1.,1.,1.,1.,1.,1.,1.,1.,1.,1.,
1.,1.,1.,1.,1.,1.))
REPRESENTATION_ITEM('')
);
#166=(
BOUNDED_CURVE()
B_SPLINE_CURVE(5,(#24805,#24806,#24807,#24808,#24809,#24810,#24811,#24812,
#24813,#24814,#24815,#24816,#24817,#24818,#24819,#24820,#24821,#24822,#24823,
#24824,#24825,#24826,#24827,#24828,#24829,#24830,#24831,#24832,#24833,#24834,
#24835,#24836,#24837,#24838,#24839,#24840,#24841,#24842,#24843,#24844,#24845,
#24846,#24847,#24848,#24849,#24850,#24851,#24852,#24853,#24854,#24855,#24856,
#24857,#24858,#24859,#24860,#24861,#24862,#24863,#24864,#24865,#24866,#24867,
#24868,#24869,#24870,#24871,#24872,#24873,#24874),.UNSPECIFIED.,.F.,.F.)
B_SPLINE_CURVE_WITH_KNOTS((6,1,1,1,1,1,1,1,1,1,1,1,1,1,1,1,1,1,1,1,1,1,
1,1,1,1,1,1,1,1,1,1,1,1,1,1,1,1,1,1,1,1,1,1,1,1,1,1,1,1,1,1,1,1,1,1,1,1,
1,1,1,1,1,1,1,6),(0.,0.0153846153846154,0.0307692307692308,0.0461538461538462,
0.0615384615384615,0.0769230769230769,0.0923076923076923,0.107692307692308,
0.123076923076923,0.138461538461538,0.153846153846154,0.169230769230769,
0.184615384615385,0.2,0.215384615384615,0.230769230769231,0.246153846153846,
0.261538461538462,0.276923076923077,0.292307692307692,0.307692307692308,
0.323076923076923,0.338461538461538,0.353846153846154,0.369230769230769,
0.384615384615385,0.4,0.415384615384615,0.430769230769231,0.446153846153846,
0.461538461538462,0.476923076923077,0.492307692307692,0.507692307692308,
0.523076923076923,0.538461538461538,0.553846153846154,0.569230769230769,
0.584615384615384,0.6,0.615384615384615,0.63076923076923,0.646153846153846,
0.661538461538461,0.676923076923076,0.692307692307692,0.707692307692307,
0.723076923076922,0.738461538461538,0.753846153846153,0.769230769230768,
0.784615384615384,0.799999999999999,0.815384615384614,0.83076923076923,
0.846153846153845,0.86153846153846,0.876923076923076,0.892307692307691,
0.907692307692306,0.923076923076922,0.938461538461537,0.953846153846152,
0.969230769230768,0.984615384615383,1.),.UNSPECIFIED.)
CURVE()
GEOMETRIC_REPRESENTATION_ITEM()
RATIONAL_B_SPLINE_CURVE((1.,1.,1.,1.,1.,1.,1.,1.,1.,1.,1.,1.,1.,1.,1.,1.,
1.,1.,1.,1.,1.,1.,1.,1.,1.,1.,1.,1.,1.,1.,1.,1.,1.,1.,1.,1.,1.,1.,1.,1.,
1.,1.,1.,1.,1.,1.,1.,1.,1.,1.,1.,1.,1.,1.,1.,1.,1.,1.,1.,1.,1.,1.,1.,1.,
1.,1.,1.,1.,1.,1.))
REPRESENTATION_ITEM('')
);
#167=(
BOUNDED_CURVE()
B_SPLINE_CURVE(5,(#24878,#24879,#24880,#24881,#24882,#24883,#24884,#24885,
#24886,#24887,#24888,#24889,#24890,#24891,#24892,#24893,#24894,#24895,#24896,
#24897,#24898,#24899,#24900,#24901,#24902,#24903,#24904,#24905,#24906,#24907,
#24908,#24909,#24910,#24911,#24912,#24913,#24914,#24915,#24916,#24917,#24918,
#24919,#24920,#24921,#24922,#24923,#24924,#24925,#24926,#24927,#24928,#24929,
#24930,#24931,#24932,#24933,#24934,#24935,#24936,#24937,#24938,#24939,#24940,
#24941,#24942,#24943,#24944,#24945,#24946,#24947),.UNSPECIFIED.,.F.,.F.)
B_SPLINE_CURVE_WITH_KNOTS((6,1,1,1,1,1,1,1,1,1,1,1,1,1,1,1,1,1,1,1,1,1,
1,1,1,1,1,1,1,1,1,1,1,1,1,1,1,1,1,1,1,1,1,1,1,1,1,1,1,1,1,1,1,1,1,1,1,1,
1,1,1,1,1,1,1,6),(0.,0.0153846153846154,0.0307692307692308,0.0461538461538462,
0.0615384615384615,0.0769230769230769,0.0923076923076923,0.107692307692308,
0.123076923076923,0.138461538461538,0.153846153846154,0.169230769230769,
0.184615384615385,0.2,0.215384615384615,0.230769230769231,0.246153846153846,
0.261538461538462,0.276923076923077,0.292307692307692,0.307692307692308,
0.323076923076923,0.338461538461538,0.353846153846154,0.369230769230769,
0.384615384615385,0.4,0.415384615384615,0.430769230769231,0.446153846153846,
0.461538461538462,0.476923076923077,0.492307692307692,0.507692307692308,
0.523076923076923,0.538461538461538,0.553846153846154,0.569230769230769,
0.584615384615384,0.6,0.615384615384615,0.63076923076923,0.646153846153846,
0.661538461538461,0.676923076923076,0.692307692307692,0.707692307692307,
0.723076923076922,0.738461538461538,0.753846153846153,0.769230769230768,
0.784615384615384,0.799999999999999,0.815384615384614,0.83076923076923,
0.846153846153845,0.86153846153846,0.876923076923076,0.892307692307691,
0.907692307692306,0.923076923076922,0.938461538461537,0.953846153846152,
0.969230769230768,0.984615384615383,1.),.UNSPECIFIED.)
CURVE()
GEOMETRIC_REPRESENTATION_ITEM()
RATIONAL_B_SPLINE_CURVE((1.,1.,1.,1.,1.,1.,1.,1.,1.,1.,1.,1.,1.,1.,1.,1.,
1.,1.,1.,1.,1.,1.,1.,1.,1.,1.,1.,1.,1.,1.,1.,1.,1.,1.,1.,1.,1.,1.,1.,1.,
1.,1.,1.,1.,1.,1.,1.,1.,1.,1.,1.,1.,1.,1.,1.,1.,1.,1.,1.,1.,1.,1.,1.,1.,
1.,1.,1.,1.,1.,1.))
REPRESENTATION_ITEM('')
);
#168=(
BOUNDED_CURVE()
B_SPLINE_CURVE(5,(#24951,#24952,#24953,#24954,#24955,#24956,#24957,#24958,
#24959,#24960,#24961,#24962,#24963,#24964,#24965,#24966,#24967,#24968,#24969,
#24970,#24971,#24972,#24973,#24974,#24975,#24976,#24977,#24978,#24979,#24980,
#24981,#24982,#24983,#24984,#24985,#24986,#24987,#24988,#24989,#24990,#24991,
#24992,#24993,#24994,#24995,#24996,#24997,#24998,#24999,#25000,#25001,#25002,
#25003,#25004,#25005,#25006,#25007,#25008,#25009,#25010,#25011,#25012,#25013,
#25014,#25015,#25016,#25017,#25018,#25019,#25020),.UNSPECIFIED.,.F.,.F.)
B_SPLINE_CURVE_WITH_KNOTS((6,1,1,1,1,1,1,1,1,1,1,1,1,1,1,1,1,1,1,1,1,1,
1,1,1,1,1,1,1,1,1,1,1,1,1,1,1,1,1,1,1,1,1,1,1,1,1,1,1,1,1,1,1,1,1,1,1,1,
1,1,1,1,1,1,1,6),(0.,0.0153846153846154,0.0307692307692308,0.0461538461538462,
0.0615384615384615,0.0769230769230769,0.0923076923076923,0.107692307692308,
0.123076923076923,0.138461538461538,0.153846153846154,0.169230769230769,
0.184615384615385,0.2,0.215384615384615,0.230769230769231,0.246153846153846,
0.261538461538462,0.276923076923077,0.292307692307692,0.307692307692308,
0.323076923076923,0.338461538461538,0.353846153846154,0.369230769230769,
0.384615384615385,0.4,0.415384615384615,0.430769230769231,0.446153846153846,
0.461538461538462,0.476923076923077,0.492307692307692,0.507692307692308,
0.523076923076923,0.538461538461538,0.553846153846154,0.569230769230769,
0.584615384615384,0.6,0.615384615384615,0.63076923076923,0.646153846153846,
0.661538461538461,0.676923076923076,0.692307692307692,0.707692307692307,
0.723076923076922,0.738461538461538,0.753846153846153,0.769230769230768,
0.784615384615384,0.799999999999999,0.815384615384614,0.83076923076923,
0.846153846153845,0.86153846153846,0.876923076923076,0.892307692307691,
0.907692307692306,0.923076923076922,0.938461538461537,0.953846153846152,
0.969230769230768,0.984615384615383,1.),.UNSPECIFIED.)
CURVE()
GEOMETRIC_REPRESENTATION_ITEM()
RATIONAL_B_SPLINE_CURVE((1.,1.,1.,1.,1.,1.,1.,1.,1.,1.,1.,1.,1.,1.,1.,1.,
1.,1.,1.,1.,1.,1.,1.,1.,1.,1.,1.,1.,1.,1.,1.,1.,1.,1.,1.,1.,1.,1.,1.,1.,
1.,1.,1.,1.,1.,1.,1.,1.,1.,1.,1.,1.,1.,1.,1.,1.,1.,1.,1.,1.,1.,1.,1.,1.,
1.,1.,1.,1.,1.,1.))
REPRESENTATION_ITEM('')
);
#169=(
BOUNDED_CURVE()
B_SPLINE_CURVE(5,(#25024,#25025,#25026,#25027,#25028,#25029,#25030,#25031,
#25032,#25033,#25034,#25035,#25036,#25037,#25038,#25039,#25040,#25041,#25042,
#25043,#25044,#25045,#25046,#25047,#25048,#25049,#25050,#25051,#25052,#25053,
#25054,#25055,#25056,#25057,#25058,#25059,#25060,#25061,#25062,#25063,#25064,
#25065,#25066,#25067,#25068,#25069,#25070,#25071,#25072,#25073,#25074,#25075,
#25076,#25077,#25078,#25079,#25080,#25081,#25082,#25083,#25084,#25085,#25086,
#25087,#25088,#25089,#25090,#25091,#25092,#25093),.UNSPECIFIED.,.F.,.F.)
B_SPLINE_CURVE_WITH_KNOTS((6,1,1,1,1,1,1,1,1,1,1,1,1,1,1,1,1,1,1,1,1,1,
1,1,1,1,1,1,1,1,1,1,1,1,1,1,1,1,1,1,1,1,1,1,1,1,1,1,1,1,1,1,1,1,1,1,1,1,
1,1,1,1,1,1,1,6),(0.,0.0153846153846154,0.0307692307692308,0.0461538461538462,
0.0615384615384615,0.0769230769230769,0.0923076923076923,0.107692307692308,
0.123076923076923,0.138461538461538,0.153846153846154,0.169230769230769,
0.184615384615385,0.2,0.215384615384615,0.230769230769231,0.246153846153846,
0.261538461538462,0.276923076923077,0.292307692307692,0.307692307692308,
0.323076923076923,0.338461538461538,0.353846153846154,0.369230769230769,
0.384615384615385,0.4,0.415384615384615,0.430769230769231,0.446153846153846,
0.461538461538462,0.476923076923077,0.492307692307692,0.507692307692308,
0.523076923076923,0.538461538461538,0.553846153846154,0.569230769230769,
0.584615384615384,0.6,0.615384615384615,0.63076923076923,0.646153846153846,
0.661538461538461,0.676923076923076,0.692307692307692,0.707692307692307,
0.723076923076922,0.738461538461538,0.753846153846153,0.769230769230768,
0.784615384615384,0.799999999999999,0.815384615384614,0.83076923076923,
0.846153846153845,0.86153846153846,0.876923076923076,0.892307692307691,
0.907692307692306,0.923076923076922,0.938461538461537,0.953846153846152,
0.969230769230768,0.984615384615383,1.),.UNSPECIFIED.)
CURVE()
GEOMETRIC_REPRESENTATION_ITEM()
RATIONAL_B_SPLINE_CURVE((1.,1.,1.,1.,1.,1.,1.,1.,1.,1.,1.,1.,1.,1.,1.,1.,
1.,1.,1.,1.,1.,1.,1.,1.,1.,1.,1.,1.,1.,1.,1.,1.,1.,1.,1.,1.,1.,1.,1.,1.,
1.,1.,1.,1.,1.,1.,1.,1.,1.,1.,1.,1.,1.,1.,1.,1.,1.,1.,1.,1.,1.,1.,1.,1.,
1.,1.,1.,1.,1.,1.))
REPRESENTATION_ITEM('')
);
#170=(
BOUNDED_CURVE()
B_SPLINE_CURVE(5,(#25096,#25097,#25098,#25099,#25100,#25101,#25102,#25103,
#25104,#25105,#25106,#25107,#25108,#25109,#25110,#25111,#25112,#25113,#25114,
#25115,#25116,#25117,#25118,#25119,#25120,#25121,#25122,#25123,#25124,#25125,
#25126,#25127,#25128,#25129,#25130,#25131,#25132,#25133,#25134,#25135,#25136,
#25137,#25138,#25139,#25140,#25141,#25142,#25143,#25144,#25145,#25146,#25147,
#25148,#25149,#25150,#25151,#25152,#25153,#25154,#25155,#25156,#25157,#25158,
#25159,#25160,#25161,#25162,#25163,#25164,#25165),.UNSPECIFIED.,.F.,.F.)
B_SPLINE_CURVE_WITH_KNOTS((6,1,1,1,1,1,1,1,1,1,1,1,1,1,1,1,1,1,1,1,1,1,
1,1,1,1,1,1,1,1,1,1,1,1,1,1,1,1,1,1,1,1,1,1,1,1,1,1,1,1,1,1,1,1,1,1,1,1,
1,1,1,1,1,1,1,6),(0.,0.0153846153846154,0.0307692307692308,0.0461538461538462,
0.0615384615384615,0.0769230769230769,0.0923076923076923,0.107692307692308,
0.123076923076923,0.138461538461538,0.153846153846154,0.169230769230769,
0.184615384615385,0.2,0.215384615384615,0.230769230769231,0.246153846153846,
0.261538461538462,0.276923076923077,0.292307692307692,0.307692307692308,
0.323076923076923,0.338461538461538,0.353846153846154,0.369230769230769,
0.384615384615385,0.4,0.415384615384615,0.430769230769231,0.446153846153846,
0.461538461538462,0.476923076923077,0.492307692307692,0.507692307692308,
0.523076923076923,0.538461538461538,0.553846153846154,0.569230769230769,
0.584615384615384,0.6,0.615384615384615,0.63076923076923,0.646153846153846,
0.661538461538461,0.676923076923076,0.692307692307692,0.707692307692307,
0.723076923076922,0.738461538461538,0.753846153846153,0.769230769230768,
0.784615384615384,0.799999999999999,0.815384615384614,0.83076923076923,
0.846153846153845,0.86153846153846,0.876923076923076,0.892307692307691,
0.907692307692306,0.923076923076922,0.938461538461537,0.953846153846152,
0.969230769230768,0.984615384615383,1.),.UNSPECIFIED.)
CURVE()
GEOMETRIC_REPRESENTATION_ITEM()
RATIONAL_B_SPLINE_CURVE((1.,1.,1.,1.,1.,1.,1.,1.,1.,1.,1.,1.,1.,1.,1.,1.,
1.,1.,1.,1.,1.,1.,1.,1.,1.,1.,1.,1.,1.,1.,1.,1.,1.,1.,1.,1.,1.,1.,1.,1.,
1.,1.,1.,1.,1.,1.,1.,1.,1.,1.,1.,1.,1.,1.,1.,1.,1.,1.,1.,1.,1.,1.,1.,1.,
1.,1.,1.,1.,1.,1.))
REPRESENTATION_ITEM('')
);
#171=(
BOUNDED_CURVE()
B_SPLINE_CURVE(5,(#25319,#25320,#25321,#25322,#25323,#25324,#25325,#25326,
#25327,#25328,#25329,#25330,#25331,#25332,#25333,#25334,#25335,#25336,#25337,
#25338,#25339,#25340,#25341,#25342,#25343,#25344,#25345,#25346,#25347,#25348,
#25349,#25350,#25351,#25352,#25353,#25354,#25355,#25356,#25357,#25358,#25359,
#25360,#25361,#25362,#25363,#25364,#25365,#25366,#25367,#25368,#25369,#25370,
#25371,#25372,#25373,#25374,#25375,#25376,#25377,#25378,#25379,#25380,#25381,
#25382,#25383,#25384,#25385,#25386,#25387,#25388),.UNSPECIFIED.,.F.,.F.)
B_SPLINE_CURVE_WITH_KNOTS((6,1,1,1,1,1,1,1,1,1,1,1,1,1,1,1,1,1,1,1,1,1,
1,1,1,1,1,1,1,1,1,1,1,1,1,1,1,1,1,1,1,1,1,1,1,1,1,1,1,1,1,1,1,1,1,1,1,1,
1,1,1,1,1,1,1,6),(-1.,-0.984615384615383,-0.969230769230768,-0.953846153846152,
-0.938461538461537,-0.923076923076922,-0.907692307692306,-0.892307692307691,
-0.876923076923076,-0.86153846153846,-0.846153846153845,-0.83076923076923,
-0.815384615384614,-0.799999999999999,-0.784615384615384,-0.769230769230768,
-0.753846153846153,-0.738461538461538,-0.723076923076922,-0.707692307692307,
-0.692307692307692,-0.676923076923076,-0.661538461538461,-0.646153846153846,
-0.63076923076923,-0.615384615384615,-0.6,-0.584615384615384,-0.569230769230769,
-0.553846153846154,-0.538461538461538,-0.523076923076923,-0.507692307692308,
-0.492307692307692,-0.476923076923077,-0.461538461538462,-0.446153846153846,
-0.430769230769231,-0.415384615384615,-0.4,-0.384615384615385,-0.369230769230769,
-0.353846153846154,-0.338461538461538,-0.323076923076923,-0.307692307692308,
-0.292307692307692,-0.276923076923077,-0.261538461538462,-0.246153846153846,
-0.230769230769231,-0.215384615384615,-0.2,-0.184615384615385,-0.169230769230769,
-0.153846153846154,-0.138461538461538,-0.123076923076923,-0.107692307692308,
-0.0923076923076923,-0.0769230769230769,-0.0615384615384615,-0.0461538461538462,
-0.0307692307692308,-0.0153846153846154,0.),.UNSPECIFIED.)
CURVE()
GEOMETRIC_REPRESENTATION_ITEM()
RATIONAL_B_SPLINE_CURVE((1.,1.,1.,1.,1.,1.,1.,1.,1.,1.,1.,1.,1.,1.,1.,1.,
1.,1.,1.,1.,1.,1.,1.,1.,1.,1.,1.,1.,1.,1.,1.,1.,1.,1.,1.,1.,1.,1.,1.,1.,
1.,1.,1.,1.,1.,1.,1.,1.,1.,1.,1.,1.,1.,1.,1.,1.,1.,1.,1.,1.,1.,1.,1.,1.,
1.,1.,1.,1.,1.,1.))
REPRESENTATION_ITEM('')
);
#172=(
BOUNDED_CURVE()
B_SPLINE_CURVE(5,(#25535,#25536,#25537,#25538,#25539,#25540,#25541,#25542,
#25543,#25544,#25545,#25546,#25547,#25548,#25549,#25550,#25551,#25552,#25553,
#25554,#25555,#25556,#25557,#25558,#25559,#25560,#25561,#25562,#25563,#25564,
#25565,#25566,#25567,#25568,#25569,#25570,#25571,#25572,#25573,#25574,#25575,
#25576,#25577,#25578,#25579,#25580,#25581,#25582,#25583,#25584,#25585,#25586,
#25587,#25588,#25589,#25590,#25591,#25592,#25593,#25594,#25595,#25596,#25597,
#25598,#25599,#25600,#25601,#25602,#25603,#25604),.UNSPECIFIED.,.F.,.F.)
B_SPLINE_CURVE_WITH_KNOTS((6,1,1,1,1,1,1,1,1,1,1,1,1,1,1,1,1,1,1,1,1,1,
1,1,1,1,1,1,1,1,1,1,1,1,1,1,1,1,1,1,1,1,1,1,1,1,1,1,1,1,1,1,1,1,1,1,1,1,
1,1,1,1,1,1,1,6),(-1.,-0.984615384615383,-0.969230769230768,-0.953846153846152,
-0.938461538461537,-0.923076923076922,-0.907692307692306,-0.892307692307691,
-0.876923076923076,-0.86153846153846,-0.846153846153845,-0.83076923076923,
-0.815384615384614,-0.799999999999999,-0.784615384615384,-0.769230769230768,
-0.753846153846153,-0.738461538461538,-0.723076923076922,-0.707692307692307,
-0.692307692307692,-0.676923076923076,-0.661538461538461,-0.646153846153846,
-0.63076923076923,-0.615384615384615,-0.6,-0.584615384615384,-0.569230769230769,
-0.553846153846154,-0.538461538461538,-0.523076923076923,-0.507692307692308,
-0.492307692307692,-0.476923076923077,-0.461538461538462,-0.446153846153846,
-0.430769230769231,-0.415384615384615,-0.4,-0.384615384615385,-0.369230769230769,
-0.353846153846154,-0.338461538461538,-0.323076923076923,-0.307692307692308,
-0.292307692307692,-0.276923076923077,-0.261538461538462,-0.246153846153846,
-0.230769230769231,-0.215384615384615,-0.2,-0.184615384615385,-0.169230769230769,
-0.153846153846154,-0.138461538461538,-0.123076923076923,-0.107692307692308,
-0.0923076923076923,-0.0769230769230769,-0.0615384615384615,-0.0461538461538462,
-0.0307692307692308,-0.0153846153846154,0.),.UNSPECIFIED.)
CURVE()
GEOMETRIC_REPRESENTATION_ITEM()
RATIONAL_B_SPLINE_CURVE((1.,1.,1.,1.,1.,1.,1.,1.,1.,1.,1.,1.,1.,1.,1.,1.,
1.,1.,1.,1.,1.,1.,1.,1.,1.,1.,1.,1.,1.,1.,1.,1.,1.,1.,1.,1.,1.,1.,1.,1.,
1.,1.,1.,1.,1.,1.,1.,1.,1.,1.,1.,1.,1.,1.,1.,1.,1.,1.,1.,1.,1.,1.,1.,1.,
1.,1.,1.,1.,1.,1.))
REPRESENTATION_ITEM('')
);
#173=(
BOUNDED_CURVE()
B_SPLINE_CURVE(5,(#25751,#25752,#25753,#25754,#25755,#25756,#25757,#25758,
#25759,#25760,#25761,#25762,#25763,#25764,#25765,#25766,#25767,#25768,#25769,
#25770,#25771,#25772,#25773,#25774,#25775,#25776,#25777,#25778,#25779,#25780,
#25781,#25782,#25783,#25784,#25785,#25786,#25787,#25788,#25789,#25790,#25791,
#25792,#25793,#25794,#25795,#25796,#25797,#25798,#25799,#25800,#25801,#25802,
#25803,#25804,#25805,#25806,#25807,#25808,#25809,#25810,#25811,#25812,#25813,
#25814,#25815,#25816,#25817,#25818,#25819,#25820),.UNSPECIFIED.,.F.,.F.)
B_SPLINE_CURVE_WITH_KNOTS((6,1,1,1,1,1,1,1,1,1,1,1,1,1,1,1,1,1,1,1,1,1,
1,1,1,1,1,1,1,1,1,1,1,1,1,1,1,1,1,1,1,1,1,1,1,1,1,1,1,1,1,1,1,1,1,1,1,1,
1,1,1,1,1,1,1,6),(-1.,-0.984615384615383,-0.969230769230768,-0.953846153846152,
-0.938461538461537,-0.923076923076922,-0.907692307692306,-0.892307692307691,
-0.876923076923076,-0.86153846153846,-0.846153846153845,-0.83076923076923,
-0.815384615384614,-0.799999999999999,-0.784615384615384,-0.769230769230768,
-0.753846153846153,-0.738461538461538,-0.723076923076922,-0.707692307692307,
-0.692307692307692,-0.676923076923076,-0.661538461538461,-0.646153846153846,
-0.63076923076923,-0.615384615384615,-0.6,-0.584615384615384,-0.569230769230769,
-0.553846153846154,-0.538461538461538,-0.523076923076923,-0.507692307692308,
-0.492307692307692,-0.476923076923077,-0.461538461538462,-0.446153846153846,
-0.430769230769231,-0.415384615384615,-0.4,-0.384615384615385,-0.369230769230769,
-0.353846153846154,-0.338461538461538,-0.323076923076923,-0.307692307692308,
-0.292307692307692,-0.276923076923077,-0.261538461538462,-0.246153846153846,
-0.230769230769231,-0.215384615384615,-0.2,-0.184615384615385,-0.169230769230769,
-0.153846153846154,-0.138461538461538,-0.123076923076923,-0.107692307692308,
-0.0923076923076923,-0.0769230769230769,-0.0615384615384615,-0.0461538461538462,
-0.0307692307692308,-0.0153846153846154,0.),.UNSPECIFIED.)
CURVE()
GEOMETRIC_REPRESENTATION_ITEM()
RATIONAL_B_SPLINE_CURVE((1.,1.,1.,1.,1.,1.,1.,1.,1.,1.,1.,1.,1.,1.,1.,1.,
1.,1.,1.,1.,1.,1.,1.,1.,1.,1.,1.,1.,1.,1.,1.,1.,1.,1.,1.,1.,1.,1.,1.,1.,
1.,1.,1.,1.,1.,1.,1.,1.,1.,1.,1.,1.,1.,1.,1.,1.,1.,1.,1.,1.,1.,1.,1.,1.,
1.,1.,1.,1.,1.,1.))
REPRESENTATION_ITEM('')
);
#174=(
BOUNDED_CURVE()
B_SPLINE_CURVE(5,(#25967,#25968,#25969,#25970,#25971,#25972,#25973,#25974,
#25975,#25976,#25977,#25978,#25979,#25980,#25981,#25982,#25983,#25984,#25985,
#25986,#25987,#25988,#25989,#25990,#25991,#25992,#25993,#25994,#25995,#25996,
#25997,#25998,#25999,#26000,#26001,#26002,#26003,#26004,#26005,#26006,#26007,
#26008,#26009,#26010,#26011,#26012,#26013,#26014,#26015,#26016,#26017,#26018,
#26019,#26020,#26021,#26022,#26023,#26024,#26025,#26026,#26027,#26028,#26029,
#26030,#26031,#26032,#26033,#26034,#26035,#26036),.UNSPECIFIED.,.F.,.F.)
B_SPLINE_CURVE_WITH_KNOTS((6,1,1,1,1,1,1,1,1,1,1,1,1,1,1,1,1,1,1,1,1,1,
1,1,1,1,1,1,1,1,1,1,1,1,1,1,1,1,1,1,1,1,1,1,1,1,1,1,1,1,1,1,1,1,1,1,1,1,
1,1,1,1,1,1,1,6),(-1.,-0.984615384615383,-0.969230769230768,-0.953846153846152,
-0.938461538461537,-0.923076923076922,-0.907692307692306,-0.892307692307691,
-0.876923076923076,-0.86153846153846,-0.846153846153845,-0.83076923076923,
-0.815384615384614,-0.799999999999999,-0.784615384615384,-0.769230769230768,
-0.753846153846153,-0.738461538461538,-0.723076923076922,-0.707692307692307,
-0.692307692307692,-0.676923076923076,-0.661538461538461,-0.646153846153846,
-0.63076923076923,-0.615384615384615,-0.6,-0.584615384615384,-0.569230769230769,
-0.553846153846154,-0.538461538461538,-0.523076923076923,-0.507692307692308,
-0.492307692307692,-0.476923076923077,-0.461538461538462,-0.446153846153846,
-0.430769230769231,-0.415384615384615,-0.4,-0.384615384615385,-0.369230769230769,
-0.353846153846154,-0.338461538461538,-0.323076923076923,-0.307692307692308,
-0.292307692307692,-0.276923076923077,-0.261538461538462,-0.246153846153846,
-0.230769230769231,-0.215384615384615,-0.2,-0.184615384615385,-0.169230769230769,
-0.153846153846154,-0.138461538461538,-0.123076923076923,-0.107692307692308,
-0.0923076923076923,-0.0769230769230769,-0.0615384615384615,-0.0461538461538462,
-0.0307692307692308,-0.0153846153846154,0.),.UNSPECIFIED.)
CURVE()
GEOMETRIC_REPRESENTATION_ITEM()
RATIONAL_B_SPLINE_CURVE((1.,1.,1.,1.,1.,1.,1.,1.,1.,1.,1.,1.,1.,1.,1.,1.,
1.,1.,1.,1.,1.,1.,1.,1.,1.,1.,1.,1.,1.,1.,1.,1.,1.,1.,1.,1.,1.,1.,1.,1.,
1.,1.,1.,1.,1.,1.,1.,1.,1.,1.,1.,1.,1.,1.,1.,1.,1.,1.,1.,1.,1.,1.,1.,1.,
1.,1.,1.,1.,1.,1.))
REPRESENTATION_ITEM('')
);
#175=(
BOUNDED_CURVE()
B_SPLINE_CURVE(5,(#26183,#26184,#26185,#26186,#26187,#26188,#26189,#26190,
#26191,#26192,#26193,#26194,#26195,#26196,#26197,#26198,#26199,#26200,#26201,
#26202,#26203,#26204,#26205,#26206,#26207,#26208,#26209,#26210,#26211,#26212,
#26213,#26214,#26215,#26216,#26217,#26218,#26219,#26220,#26221,#26222,#26223,
#26224,#26225,#26226,#26227,#26228,#26229,#26230,#26231,#26232,#26233,#26234,
#26235,#26236,#26237,#26238,#26239,#26240,#26241,#26242,#26243,#26244,#26245,
#26246,#26247,#26248,#26249,#26250,#26251,#26252),.UNSPECIFIED.,.F.,.F.)
B_SPLINE_CURVE_WITH_KNOTS((6,1,1,1,1,1,1,1,1,1,1,1,1,1,1,1,1,1,1,1,1,1,
1,1,1,1,1,1,1,1,1,1,1,1,1,1,1,1,1,1,1,1,1,1,1,1,1,1,1,1,1,1,1,1,1,1,1,1,
1,1,1,1,1,1,1,6),(-1.,-0.984615384615383,-0.969230769230768,-0.953846153846152,
-0.938461538461537,-0.923076923076922,-0.907692307692306,-0.892307692307691,
-0.876923076923076,-0.86153846153846,-0.846153846153845,-0.83076923076923,
-0.815384615384614,-0.799999999999999,-0.784615384615384,-0.769230769230768,
-0.753846153846153,-0.738461538461538,-0.723076923076922,-0.707692307692307,
-0.692307692307692,-0.676923076923076,-0.661538461538461,-0.646153846153846,
-0.63076923076923,-0.615384615384615,-0.6,-0.584615384615384,-0.569230769230769,
-0.553846153846154,-0.538461538461538,-0.523076923076923,-0.507692307692308,
-0.492307692307692,-0.476923076923077,-0.461538461538462,-0.446153846153846,
-0.430769230769231,-0.415384615384615,-0.4,-0.384615384615385,-0.369230769230769,
-0.353846153846154,-0.338461538461538,-0.323076923076923,-0.307692307692308,
-0.292307692307692,-0.276923076923077,-0.261538461538462,-0.246153846153846,
-0.230769230769231,-0.215384615384615,-0.2,-0.184615384615385,-0.169230769230769,
-0.153846153846154,-0.138461538461538,-0.123076923076923,-0.107692307692308,
-0.0923076923076923,-0.0769230769230769,-0.0615384615384615,-0.0461538461538462,
-0.0307692307692308,-0.0153846153846154,0.),.UNSPECIFIED.)
CURVE()
GEOMETRIC_REPRESENTATION_ITEM()
RATIONAL_B_SPLINE_CURVE((1.,1.,1.,1.,1.,1.,1.,1.,1.,1.,1.,1.,1.,1.,1.,1.,
1.,1.,1.,1.,1.,1.,1.,1.,1.,1.,1.,1.,1.,1.,1.,1.,1.,1.,1.,1.,1.,1.,1.,1.,
1.,1.,1.,1.,1.,1.,1.,1.,1.,1.,1.,1.,1.,1.,1.,1.,1.,1.,1.,1.,1.,1.,1.,1.,
1.,1.,1.,1.,1.,1.))
REPRESENTATION_ITEM('')
);
#176=(
BOUNDED_CURVE()
B_SPLINE_CURVE(5,(#26399,#26400,#26401,#26402,#26403,#26404,#26405,#26406,
#26407,#26408,#26409,#26410,#26411,#26412,#26413,#26414,#26415,#26416,#26417,
#26418,#26419,#26420,#26421,#26422,#26423,#26424,#26425,#26426,#26427,#26428,
#26429,#26430,#26431,#26432,#26433,#26434,#26435,#26436,#26437,#26438,#26439,
#26440,#26441,#26442,#26443,#26444,#26445,#26446,#26447,#26448,#26449,#26450,
#26451,#26452,#26453,#26454,#26455,#26456,#26457,#26458,#26459,#26460,#26461,
#26462,#26463,#26464,#26465,#26466,#26467,#26468),.UNSPECIFIED.,.F.,.F.)
B_SPLINE_CURVE_WITH_KNOTS((6,1,1,1,1,1,1,1,1,1,1,1,1,1,1,1,1,1,1,1,1,1,
1,1,1,1,1,1,1,1,1,1,1,1,1,1,1,1,1,1,1,1,1,1,1,1,1,1,1,1,1,1,1,1,1,1,1,1,
1,1,1,1,1,1,1,6),(-1.,-0.984615384615383,-0.969230769230768,-0.953846153846152,
-0.938461538461537,-0.923076923076922,-0.907692307692306,-0.892307692307691,
-0.876923076923076,-0.86153846153846,-0.846153846153845,-0.83076923076923,
-0.815384615384614,-0.799999999999999,-0.784615384615384,-0.769230769230768,
-0.753846153846153,-0.738461538461538,-0.723076923076922,-0.707692307692307,
-0.692307692307692,-0.676923076923076,-0.661538461538461,-0.646153846153846,
-0.63076923076923,-0.615384615384615,-0.6,-0.584615384615384,-0.569230769230769,
-0.553846153846154,-0.538461538461538,-0.523076923076923,-0.507692307692308,
-0.492307692307692,-0.476923076923077,-0.461538461538462,-0.446153846153846,
-0.430769230769231,-0.415384615384615,-0.4,-0.384615384615385,-0.369230769230769,
-0.353846153846154,-0.338461538461538,-0.323076923076923,-0.307692307692308,
-0.292307692307692,-0.276923076923077,-0.261538461538462,-0.246153846153846,
-0.230769230769231,-0.215384615384615,-0.2,-0.184615384615385,-0.169230769230769,
-0.153846153846154,-0.138461538461538,-0.123076923076923,-0.107692307692308,
-0.0923076923076923,-0.0769230769230769,-0.0615384615384615,-0.0461538461538462,
-0.0307692307692308,-0.0153846153846154,0.),.UNSPECIFIED.)
CURVE()
GEOMETRIC_REPRESENTATION_ITEM()
RATIONAL_B_SPLINE_CURVE((1.,1.,1.,1.,1.,1.,1.,1.,1.,1.,1.,1.,1.,1.,1.,1.,
1.,1.,1.,1.,1.,1.,1.,1.,1.,1.,1.,1.,1.,1.,1.,1.,1.,1.,1.,1.,1.,1.,1.,1.,
1.,1.,1.,1.,1.,1.,1.,1.,1.,1.,1.,1.,1.,1.,1.,1.,1.,1.,1.,1.,1.,1.,1.,1.,
1.,1.,1.,1.,1.,1.))
REPRESENTATION_ITEM('')
);
#177=(
BOUNDED_CURVE()
B_SPLINE_CURVE(5,(#26615,#26616,#26617,#26618,#26619,#26620,#26621,#26622,
#26623,#26624,#26625,#26626,#26627,#26628,#26629,#26630,#26631,#26632,#26633,
#26634,#26635,#26636,#26637,#26638,#26639,#26640,#26641,#26642,#26643,#26644,
#26645,#26646,#26647,#26648,#26649,#26650,#26651,#26652,#26653,#26654,#26655,
#26656,#26657,#26658,#26659,#26660,#26661,#26662,#26663,#26664,#26665,#26666,
#26667,#26668,#26669,#26670,#26671,#26672,#26673,#26674,#26675,#26676,#26677,
#26678,#26679,#26680,#26681,#26682,#26683,#26684),.UNSPECIFIED.,.F.,.F.)
B_SPLINE_CURVE_WITH_KNOTS((6,1,1,1,1,1,1,1,1,1,1,1,1,1,1,1,1,1,1,1,1,1,
1,1,1,1,1,1,1,1,1,1,1,1,1,1,1,1,1,1,1,1,1,1,1,1,1,1,1,1,1,1,1,1,1,1,1,1,
1,1,1,1,1,1,1,6),(-1.,-0.984615384615383,-0.969230769230768,-0.953846153846152,
-0.938461538461537,-0.923076923076922,-0.907692307692306,-0.892307692307691,
-0.876923076923076,-0.86153846153846,-0.846153846153845,-0.83076923076923,
-0.815384615384614,-0.799999999999999,-0.784615384615384,-0.769230769230768,
-0.753846153846153,-0.738461538461538,-0.723076923076922,-0.707692307692307,
-0.692307692307692,-0.676923076923076,-0.661538461538461,-0.646153846153846,
-0.63076923076923,-0.615384615384615,-0.6,-0.584615384615384,-0.569230769230769,
-0.553846153846154,-0.538461538461538,-0.523076923076923,-0.507692307692308,
-0.492307692307692,-0.476923076923077,-0.461538461538462,-0.446153846153846,
-0.430769230769231,-0.415384615384615,-0.4,-0.384615384615385,-0.369230769230769,
-0.353846153846154,-0.338461538461538,-0.323076923076923,-0.307692307692308,
-0.292307692307692,-0.276923076923077,-0.261538461538462,-0.246153846153846,
-0.230769230769231,-0.215384615384615,-0.2,-0.184615384615385,-0.169230769230769,
-0.153846153846154,-0.138461538461538,-0.123076923076923,-0.107692307692308,
-0.0923076923076923,-0.0769230769230769,-0.0615384615384615,-0.0461538461538462,
-0.0307692307692308,-0.0153846153846154,0.),.UNSPECIFIED.)
CURVE()
GEOMETRIC_REPRESENTATION_ITEM()
RATIONAL_B_SPLINE_CURVE((1.,1.,1.,1.,1.,1.,1.,1.,1.,1.,1.,1.,1.,1.,1.,1.,
1.,1.,1.,1.,1.,1.,1.,1.,1.,1.,1.,1.,1.,1.,1.,1.,1.,1.,1.,1.,1.,1.,1.,1.,
1.,1.,1.,1.,1.,1.,1.,1.,1.,1.,1.,1.,1.,1.,1.,1.,1.,1.,1.,1.,1.,1.,1.,1.,
1.,1.,1.,1.,1.,1.))
REPRESENTATION_ITEM('')
);
#178=(
BOUNDED_CURVE()
B_SPLINE_CURVE(5,(#26831,#26832,#26833,#26834,#26835,#26836,#26837,#26838,
#26839,#26840,#26841,#26842,#26843,#26844,#26845,#26846,#26847,#26848,#26849,
#26850,#26851,#26852,#26853,#26854,#26855,#26856,#26857,#26858,#26859,#26860,
#26861,#26862,#26863,#26864,#26865,#26866,#26867,#26868,#26869,#26870,#26871,
#26872,#26873,#26874,#26875,#26876,#26877,#26878,#26879,#26880,#26881,#26882,
#26883,#26884,#26885,#26886,#26887,#26888,#26889,#26890,#26891,#26892,#26893,
#26894,#26895,#26896,#26897,#26898,#26899,#26900),.UNSPECIFIED.,.F.,.F.)
B_SPLINE_CURVE_WITH_KNOTS((6,1,1,1,1,1,1,1,1,1,1,1,1,1,1,1,1,1,1,1,1,1,
1,1,1,1,1,1,1,1,1,1,1,1,1,1,1,1,1,1,1,1,1,1,1,1,1,1,1,1,1,1,1,1,1,1,1,1,
1,1,1,1,1,1,1,6),(-1.,-0.984615384615383,-0.969230769230768,-0.953846153846152,
-0.938461538461537,-0.923076923076922,-0.907692307692306,-0.892307692307691,
-0.876923076923076,-0.86153846153846,-0.846153846153845,-0.83076923076923,
-0.815384615384614,-0.799999999999999,-0.784615384615384,-0.769230769230768,
-0.753846153846153,-0.738461538461538,-0.723076923076922,-0.707692307692307,
-0.692307692307692,-0.676923076923076,-0.661538461538461,-0.646153846153846,
-0.63076923076923,-0.615384615384615,-0.6,-0.584615384615384,-0.569230769230769,
-0.553846153846154,-0.538461538461538,-0.523076923076923,-0.507692307692308,
-0.492307692307692,-0.476923076923077,-0.461538461538462,-0.446153846153846,
-0.430769230769231,-0.415384615384615,-0.4,-0.384615384615385,-0.369230769230769,
-0.353846153846154,-0.338461538461538,-0.323076923076923,-0.307692307692308,
-0.292307692307692,-0.276923076923077,-0.261538461538462,-0.246153846153846,
-0.230769230769231,-0.215384615384615,-0.2,-0.184615384615385,-0.169230769230769,
-0.153846153846154,-0.138461538461538,-0.123076923076923,-0.107692307692308,
-0.0923076923076923,-0.0769230769230769,-0.0615384615384615,-0.0461538461538462,
-0.0307692307692308,-0.0153846153846154,0.),.UNSPECIFIED.)
CURVE()
GEOMETRIC_REPRESENTATION_ITEM()
RATIONAL_B_SPLINE_CURVE((1.,1.,1.,1.,1.,1.,1.,1.,1.,1.,1.,1.,1.,1.,1.,1.,
1.,1.,1.,1.,1.,1.,1.,1.,1.,1.,1.,1.,1.,1.,1.,1.,1.,1.,1.,1.,1.,1.,1.,1.,
1.,1.,1.,1.,1.,1.,1.,1.,1.,1.,1.,1.,1.,1.,1.,1.,1.,1.,1.,1.,1.,1.,1.,1.,
1.,1.,1.,1.,1.,1.))
REPRESENTATION_ITEM('')
);
#179=(
BOUNDED_CURVE()
B_SPLINE_CURVE(5,(#27047,#27048,#27049,#27050,#27051,#27052,#27053,#27054,
#27055,#27056,#27057,#27058,#27059,#27060,#27061,#27062,#27063,#27064,#27065,
#27066,#27067,#27068,#27069,#27070,#27071,#27072,#27073,#27074,#27075,#27076,
#27077,#27078,#27079,#27080,#27081,#27082,#27083,#27084,#27085,#27086,#27087,
#27088,#27089,#27090,#27091,#27092,#27093,#27094,#27095,#27096,#27097,#27098,
#27099,#27100,#27101,#27102,#27103,#27104,#27105,#27106,#27107,#27108,#27109,
#27110,#27111,#27112,#27113,#27114,#27115,#27116),.UNSPECIFIED.,.F.,.F.)
B_SPLINE_CURVE_WITH_KNOTS((6,1,1,1,1,1,1,1,1,1,1,1,1,1,1,1,1,1,1,1,1,1,
1,1,1,1,1,1,1,1,1,1,1,1,1,1,1,1,1,1,1,1,1,1,1,1,1,1,1,1,1,1,1,1,1,1,1,1,
1,1,1,1,1,1,1,6),(-1.,-0.984615384615383,-0.969230769230768,-0.953846153846152,
-0.938461538461537,-0.923076923076922,-0.907692307692306,-0.892307692307691,
-0.876923076923076,-0.86153846153846,-0.846153846153845,-0.83076923076923,
-0.815384615384614,-0.799999999999999,-0.784615384615384,-0.769230769230768,
-0.753846153846153,-0.738461538461538,-0.723076923076922,-0.707692307692307,
-0.692307692307692,-0.676923076923076,-0.661538461538461,-0.646153846153846,
-0.63076923076923,-0.615384615384615,-0.6,-0.584615384615384,-0.569230769230769,
-0.553846153846154,-0.538461538461538,-0.523076923076923,-0.507692307692308,
-0.492307692307692,-0.476923076923077,-0.461538461538462,-0.446153846153846,
-0.430769230769231,-0.415384615384615,-0.4,-0.384615384615385,-0.369230769230769,
-0.353846153846154,-0.338461538461538,-0.323076923076923,-0.307692307692308,
-0.292307692307692,-0.276923076923077,-0.261538461538462,-0.246153846153846,
-0.230769230769231,-0.215384615384615,-0.2,-0.184615384615385,-0.169230769230769,
-0.153846153846154,-0.138461538461538,-0.123076923076923,-0.107692307692308,
-0.0923076923076923,-0.0769230769230769,-0.0615384615384615,-0.0461538461538462,
-0.0307692307692308,-0.0153846153846154,0.),.UNSPECIFIED.)
CURVE()
GEOMETRIC_REPRESENTATION_ITEM()
RATIONAL_B_SPLINE_CURVE((1.,1.,1.,1.,1.,1.,1.,1.,1.,1.,1.,1.,1.,1.,1.,1.,
1.,1.,1.,1.,1.,1.,1.,1.,1.,1.,1.,1.,1.,1.,1.,1.,1.,1.,1.,1.,1.,1.,1.,1.,
1.,1.,1.,1.,1.,1.,1.,1.,1.,1.,1.,1.,1.,1.,1.,1.,1.,1.,1.,1.,1.,1.,1.,1.,
1.,1.,1.,1.,1.,1.))
REPRESENTATION_ITEM('')
);
#180=(
BOUNDED_CURVE()
B_SPLINE_CURVE(5,(#27263,#27264,#27265,#27266,#27267,#27268,#27269,#27270,
#27271,#27272,#27273,#27274,#27275,#27276,#27277,#27278,#27279,#27280,#27281,
#27282,#27283,#27284,#27285,#27286,#27287,#27288,#27289,#27290,#27291,#27292,
#27293,#27294,#27295,#27296,#27297,#27298,#27299,#27300,#27301,#27302,#27303,
#27304,#27305,#27306,#27307,#27308,#27309,#27310,#27311,#27312,#27313,#27314,
#27315,#27316,#27317,#27318,#27319,#27320,#27321,#27322,#27323,#27324,#27325,
#27326,#27327,#27328,#27329,#27330,#27331,#27332),.UNSPECIFIED.,.F.,.F.)
B_SPLINE_CURVE_WITH_KNOTS((6,1,1,1,1,1,1,1,1,1,1,1,1,1,1,1,1,1,1,1,1,1,
1,1,1,1,1,1,1,1,1,1,1,1,1,1,1,1,1,1,1,1,1,1,1,1,1,1,1,1,1,1,1,1,1,1,1,1,
1,1,1,1,1,1,1,6),(-1.,-0.984615384615383,-0.969230769230768,-0.953846153846152,
-0.938461538461537,-0.923076923076922,-0.907692307692306,-0.892307692307691,
-0.876923076923076,-0.86153846153846,-0.846153846153845,-0.83076923076923,
-0.815384615384614,-0.799999999999999,-0.784615384615384,-0.769230769230768,
-0.753846153846153,-0.738461538461538,-0.723076923076922,-0.707692307692307,
-0.692307692307692,-0.676923076923076,-0.661538461538461,-0.646153846153846,
-0.63076923076923,-0.615384615384615,-0.6,-0.584615384615384,-0.569230769230769,
-0.553846153846154,-0.538461538461538,-0.523076923076923,-0.507692307692308,
-0.492307692307692,-0.476923076923077,-0.461538461538462,-0.446153846153846,
-0.430769230769231,-0.415384615384615,-0.4,-0.384615384615385,-0.369230769230769,
-0.353846153846154,-0.338461538461538,-0.323076923076923,-0.307692307692308,
-0.292307692307692,-0.276923076923077,-0.261538461538462,-0.246153846153846,
-0.230769230769231,-0.215384615384615,-0.2,-0.184615384615385,-0.169230769230769,
-0.153846153846154,-0.138461538461538,-0.123076923076923,-0.107692307692308,
-0.0923076923076923,-0.0769230769230769,-0.0615384615384615,-0.0461538461538462,
-0.0307692307692308,-0.0153846153846154,0.),.UNSPECIFIED.)
CURVE()
GEOMETRIC_REPRESENTATION_ITEM()
RATIONAL_B_SPLINE_CURVE((1.,1.,1.,1.,1.,1.,1.,1.,1.,1.,1.,1.,1.,1.,1.,1.,
1.,1.,1.,1.,1.,1.,1.,1.,1.,1.,1.,1.,1.,1.,1.,1.,1.,1.,1.,1.,1.,1.,1.,1.,
1.,1.,1.,1.,1.,1.,1.,1.,1.,1.,1.,1.,1.,1.,1.,1.,1.,1.,1.,1.,1.,1.,1.,1.,
1.,1.,1.,1.,1.,1.))
REPRESENTATION_ITEM('')
);
#181=(
BOUNDED_CURVE()
B_SPLINE_CURVE(5,(#27479,#27480,#27481,#27482,#27483,#27484,#27485,#27486,
#27487,#27488,#27489,#27490,#27491,#27492,#27493,#27494,#27495,#27496,#27497,
#27498,#27499,#27500,#27501,#27502,#27503,#27504,#27505,#27506,#27507,#27508,
#27509,#27510,#27511,#27512,#27513,#27514,#27515,#27516,#27517,#27518,#27519,
#27520,#27521,#27522,#27523,#27524,#27525,#27526,#27527,#27528,#27529,#27530,
#27531,#27532,#27533,#27534,#27535,#27536,#27537,#27538,#27539,#27540,#27541,
#27542,#27543,#27544,#27545,#27546,#27547,#27548),.UNSPECIFIED.,.F.,.F.)
B_SPLINE_CURVE_WITH_KNOTS((6,1,1,1,1,1,1,1,1,1,1,1,1,1,1,1,1,1,1,1,1,1,
1,1,1,1,1,1,1,1,1,1,1,1,1,1,1,1,1,1,1,1,1,1,1,1,1,1,1,1,1,1,1,1,1,1,1,1,
1,1,1,1,1,1,1,6),(-1.,-0.984615384615383,-0.969230769230768,-0.953846153846152,
-0.938461538461537,-0.923076923076922,-0.907692307692306,-0.892307692307691,
-0.876923076923076,-0.86153846153846,-0.846153846153845,-0.83076923076923,
-0.815384615384614,-0.799999999999999,-0.784615384615384,-0.769230769230768,
-0.753846153846153,-0.738461538461538,-0.723076923076922,-0.707692307692307,
-0.692307692307692,-0.676923076923076,-0.661538461538461,-0.646153846153846,
-0.63076923076923,-0.615384615384615,-0.6,-0.584615384615384,-0.569230769230769,
-0.553846153846154,-0.538461538461538,-0.523076923076923,-0.507692307692308,
-0.492307692307692,-0.476923076923077,-0.461538461538462,-0.446153846153846,
-0.430769230769231,-0.415384615384615,-0.4,-0.384615384615385,-0.369230769230769,
-0.353846153846154,-0.338461538461538,-0.323076923076923,-0.307692307692308,
-0.292307692307692,-0.276923076923077,-0.261538461538462,-0.246153846153846,
-0.230769230769231,-0.215384615384615,-0.2,-0.184615384615385,-0.169230769230769,
-0.153846153846154,-0.138461538461538,-0.123076923076923,-0.107692307692308,
-0.0923076923076923,-0.0769230769230769,-0.0615384615384615,-0.0461538461538462,
-0.0307692307692308,-0.0153846153846154,0.),.UNSPECIFIED.)
CURVE()
GEOMETRIC_REPRESENTATION_ITEM()
RATIONAL_B_SPLINE_CURVE((1.,1.,1.,1.,1.,1.,1.,1.,1.,1.,1.,1.,1.,1.,1.,1.,
1.,1.,1.,1.,1.,1.,1.,1.,1.,1.,1.,1.,1.,1.,1.,1.,1.,1.,1.,1.,1.,1.,1.,1.,
1.,1.,1.,1.,1.,1.,1.,1.,1.,1.,1.,1.,1.,1.,1.,1.,1.,1.,1.,1.,1.,1.,1.,1.,
1.,1.,1.,1.,1.,1.))
REPRESENTATION_ITEM('')
);
#182=(
BOUNDED_CURVE()
B_SPLINE_CURVE(5,(#27695,#27696,#27697,#27698,#27699,#27700,#27701,#27702,
#27703,#27704,#27705,#27706,#27707,#27708,#27709,#27710,#27711,#27712,#27713,
#27714,#27715,#27716,#27717,#27718,#27719,#27720,#27721,#27722,#27723,#27724,
#27725,#27726,#27727,#27728,#27729,#27730,#27731,#27732,#27733,#27734,#27735,
#27736,#27737,#27738,#27739,#27740,#27741,#27742,#27743,#27744,#27745,#27746,
#27747,#27748,#27749,#27750,#27751,#27752,#27753,#27754,#27755,#27756,#27757,
#27758,#27759,#27760,#27761,#27762,#27763,#27764),.UNSPECIFIED.,.F.,.F.)
B_SPLINE_CURVE_WITH_KNOTS((6,1,1,1,1,1,1,1,1,1,1,1,1,1,1,1,1,1,1,1,1,1,
1,1,1,1,1,1,1,1,1,1,1,1,1,1,1,1,1,1,1,1,1,1,1,1,1,1,1,1,1,1,1,1,1,1,1,1,
1,1,1,1,1,1,1,6),(-1.,-0.984615384615383,-0.969230769230768,-0.953846153846152,
-0.938461538461537,-0.923076923076922,-0.907692307692306,-0.892307692307691,
-0.876923076923076,-0.86153846153846,-0.846153846153845,-0.83076923076923,
-0.815384615384614,-0.799999999999999,-0.784615384615384,-0.769230769230768,
-0.753846153846153,-0.738461538461538,-0.723076923076922,-0.707692307692307,
-0.692307692307692,-0.676923076923076,-0.661538461538461,-0.646153846153846,
-0.63076923076923,-0.615384615384615,-0.6,-0.584615384615384,-0.569230769230769,
-0.553846153846154,-0.538461538461538,-0.523076923076923,-0.507692307692308,
-0.492307692307692,-0.476923076923077,-0.461538461538462,-0.446153846153846,
-0.430769230769231,-0.415384615384615,-0.4,-0.384615384615385,-0.369230769230769,
-0.353846153846154,-0.338461538461538,-0.323076923076923,-0.307692307692308,
-0.292307692307692,-0.276923076923077,-0.261538461538462,-0.246153846153846,
-0.230769230769231,-0.215384615384615,-0.2,-0.184615384615385,-0.169230769230769,
-0.153846153846154,-0.138461538461538,-0.123076923076923,-0.107692307692308,
-0.0923076923076923,-0.0769230769230769,-0.0615384615384615,-0.0461538461538462,
-0.0307692307692308,-0.0153846153846154,0.),.UNSPECIFIED.)
CURVE()
GEOMETRIC_REPRESENTATION_ITEM()
RATIONAL_B_SPLINE_CURVE((1.,1.,1.,1.,1.,1.,1.,1.,1.,1.,1.,1.,1.,1.,1.,1.,
1.,1.,1.,1.,1.,1.,1.,1.,1.,1.,1.,1.,1.,1.,1.,1.,1.,1.,1.,1.,1.,1.,1.,1.,
1.,1.,1.,1.,1.,1.,1.,1.,1.,1.,1.,1.,1.,1.,1.,1.,1.,1.,1.,1.,1.,1.,1.,1.,
1.,1.,1.,1.,1.,1.))
REPRESENTATION_ITEM('')
);
#183=(
BOUNDED_CURVE()
B_SPLINE_CURVE(5,(#27911,#27912,#27913,#27914,#27915,#27916,#27917,#27918,
#27919,#27920,#27921,#27922,#27923,#27924,#27925,#27926,#27927,#27928,#27929,
#27930,#27931,#27932,#27933,#27934,#27935,#27936,#27937,#27938,#27939,#27940,
#27941,#27942,#27943,#27944,#27945,#27946,#27947,#27948,#27949,#27950,#27951,
#27952,#27953,#27954,#27955,#27956,#27957,#27958,#27959,#27960,#27961,#27962,
#27963,#27964,#27965,#27966,#27967,#27968,#27969,#27970,#27971,#27972,#27973,
#27974,#27975,#27976,#27977,#27978,#27979,#27980),.UNSPECIFIED.,.F.,.F.)
B_SPLINE_CURVE_WITH_KNOTS((6,1,1,1,1,1,1,1,1,1,1,1,1,1,1,1,1,1,1,1,1,1,
1,1,1,1,1,1,1,1,1,1,1,1,1,1,1,1,1,1,1,1,1,1,1,1,1,1,1,1,1,1,1,1,1,1,1,1,
1,1,1,1,1,1,1,6),(-1.,-0.984615384615383,-0.969230769230768,-0.953846153846152,
-0.938461538461537,-0.923076923076922,-0.907692307692306,-0.892307692307691,
-0.876923076923076,-0.86153846153846,-0.846153846153845,-0.83076923076923,
-0.815384615384614,-0.799999999999999,-0.784615384615384,-0.769230769230768,
-0.753846153846153,-0.738461538461538,-0.723076923076922,-0.707692307692307,
-0.692307692307692,-0.676923076923076,-0.661538461538461,-0.646153846153846,
-0.63076923076923,-0.615384615384615,-0.6,-0.584615384615384,-0.569230769230769,
-0.553846153846154,-0.538461538461538,-0.523076923076923,-0.507692307692308,
-0.492307692307692,-0.476923076923077,-0.461538461538462,-0.446153846153846,
-0.430769230769231,-0.415384615384615,-0.4,-0.384615384615385,-0.369230769230769,
-0.353846153846154,-0.338461538461538,-0.323076923076923,-0.307692307692308,
-0.292307692307692,-0.276923076923077,-0.261538461538462,-0.246153846153846,
-0.230769230769231,-0.215384615384615,-0.2,-0.184615384615385,-0.169230769230769,
-0.153846153846154,-0.138461538461538,-0.123076923076923,-0.107692307692308,
-0.0923076923076923,-0.0769230769230769,-0.0615384615384615,-0.0461538461538462,
-0.0307692307692308,-0.0153846153846154,0.),.UNSPECIFIED.)
CURVE()
GEOMETRIC_REPRESENTATION_ITEM()
RATIONAL_B_SPLINE_CURVE((1.,1.,1.,1.,1.,1.,1.,1.,1.,1.,1.,1.,1.,1.,1.,1.,
1.,1.,1.,1.,1.,1.,1.,1.,1.,1.,1.,1.,1.,1.,1.,1.,1.,1.,1.,1.,1.,1.,1.,1.,
1.,1.,1.,1.,1.,1.,1.,1.,1.,1.,1.,1.,1.,1.,1.,1.,1.,1.,1.,1.,1.,1.,1.,1.,
1.,1.,1.,1.,1.,1.))
REPRESENTATION_ITEM('')
);
#184=(
BOUNDED_CURVE()
B_SPLINE_CURVE(5,(#28127,#28128,#28129,#28130,#28131,#28132,#28133,#28134,
#28135,#28136,#28137,#28138,#28139,#28140,#28141,#28142,#28143,#28144,#28145,
#28146,#28147,#28148,#28149,#28150,#28151,#28152,#28153,#28154,#28155,#28156,
#28157,#28158,#28159,#28160,#28161,#28162,#28163,#28164,#28165,#28166,#28167,
#28168,#28169,#28170,#28171,#28172,#28173,#28174,#28175,#28176,#28177,#28178,
#28179,#28180,#28181,#28182,#28183,#28184,#28185,#28186,#28187,#28188,#28189,
#28190,#28191,#28192,#28193,#28194,#28195,#28196),.UNSPECIFIED.,.F.,.F.)
B_SPLINE_CURVE_WITH_KNOTS((6,1,1,1,1,1,1,1,1,1,1,1,1,1,1,1,1,1,1,1,1,1,
1,1,1,1,1,1,1,1,1,1,1,1,1,1,1,1,1,1,1,1,1,1,1,1,1,1,1,1,1,1,1,1,1,1,1,1,
1,1,1,1,1,1,1,6),(-1.,-0.984615384615383,-0.969230769230768,-0.953846153846152,
-0.938461538461537,-0.923076923076922,-0.907692307692306,-0.892307692307691,
-0.876923076923076,-0.86153846153846,-0.846153846153845,-0.83076923076923,
-0.815384615384614,-0.799999999999999,-0.784615384615384,-0.769230769230768,
-0.753846153846153,-0.738461538461538,-0.723076923076922,-0.707692307692307,
-0.692307692307692,-0.676923076923076,-0.661538461538461,-0.646153846153846,
-0.63076923076923,-0.615384615384615,-0.6,-0.584615384615384,-0.569230769230769,
-0.553846153846154,-0.538461538461538,-0.523076923076923,-0.507692307692308,
-0.492307692307692,-0.476923076923077,-0.461538461538462,-0.446153846153846,
-0.430769230769231,-0.415384615384615,-0.4,-0.384615384615385,-0.369230769230769,
-0.353846153846154,-0.338461538461538,-0.323076923076923,-0.307692307692308,
-0.292307692307692,-0.276923076923077,-0.261538461538462,-0.246153846153846,
-0.230769230769231,-0.215384615384615,-0.2,-0.184615384615385,-0.169230769230769,
-0.153846153846154,-0.138461538461538,-0.123076923076923,-0.107692307692308,
-0.0923076923076923,-0.0769230769230769,-0.0615384615384615,-0.0461538461538462,
-0.0307692307692308,-0.0153846153846154,0.),.UNSPECIFIED.)
CURVE()
GEOMETRIC_REPRESENTATION_ITEM()
RATIONAL_B_SPLINE_CURVE((1.,1.,1.,1.,1.,1.,1.,1.,1.,1.,1.,1.,1.,1.,1.,1.,
1.,1.,1.,1.,1.,1.,1.,1.,1.,1.,1.,1.,1.,1.,1.,1.,1.,1.,1.,1.,1.,1.,1.,1.,
1.,1.,1.,1.,1.,1.,1.,1.,1.,1.,1.,1.,1.,1.,1.,1.,1.,1.,1.,1.,1.,1.,1.,1.,
1.,1.,1.,1.,1.,1.))
REPRESENTATION_ITEM('')
);
#185=(
BOUNDED_CURVE()
B_SPLINE_CURVE(5,(#28343,#28344,#28345,#28346,#28347,#28348,#28349,#28350,
#28351,#28352,#28353,#28354,#28355,#28356,#28357,#28358,#28359,#28360,#28361,
#28362,#28363,#28364,#28365,#28366,#28367,#28368,#28369,#28370,#28371,#28372,
#28373,#28374,#28375,#28376,#28377,#28378,#28379,#28380,#28381,#28382,#28383,
#28384,#28385,#28386,#28387,#28388,#28389,#28390,#28391,#28392,#28393,#28394,
#28395,#28396,#28397,#28398,#28399,#28400,#28401,#28402,#28403,#28404,#28405,
#28406,#28407,#28408,#28409,#28410,#28411,#28412),.UNSPECIFIED.,.F.,.F.)
B_SPLINE_CURVE_WITH_KNOTS((6,1,1,1,1,1,1,1,1,1,1,1,1,1,1,1,1,1,1,1,1,1,
1,1,1,1,1,1,1,1,1,1,1,1,1,1,1,1,1,1,1,1,1,1,1,1,1,1,1,1,1,1,1,1,1,1,1,1,
1,1,1,1,1,1,1,6),(-1.,-0.984615384615383,-0.969230769230768,-0.953846153846152,
-0.938461538461537,-0.923076923076922,-0.907692307692306,-0.892307692307691,
-0.876923076923076,-0.86153846153846,-0.846153846153845,-0.83076923076923,
-0.815384615384614,-0.799999999999999,-0.784615384615384,-0.769230769230768,
-0.753846153846153,-0.738461538461538,-0.723076923076922,-0.707692307692307,
-0.692307692307692,-0.676923076923076,-0.661538461538461,-0.646153846153846,
-0.63076923076923,-0.615384615384615,-0.6,-0.584615384615384,-0.569230769230769,
-0.553846153846154,-0.538461538461538,-0.523076923076923,-0.507692307692308,
-0.492307692307692,-0.476923076923077,-0.461538461538462,-0.446153846153846,
-0.430769230769231,-0.415384615384615,-0.4,-0.384615384615385,-0.369230769230769,
-0.353846153846154,-0.338461538461538,-0.323076923076923,-0.307692307692308,
-0.292307692307692,-0.276923076923077,-0.261538461538462,-0.246153846153846,
-0.230769230769231,-0.215384615384615,-0.2,-0.184615384615385,-0.169230769230769,
-0.153846153846154,-0.138461538461538,-0.123076923076923,-0.107692307692308,
-0.0923076923076923,-0.0769230769230769,-0.0615384615384615,-0.0461538461538462,
-0.0307692307692308,-0.0153846153846154,0.),.UNSPECIFIED.)
CURVE()
GEOMETRIC_REPRESENTATION_ITEM()
RATIONAL_B_SPLINE_CURVE((1.,1.,1.,1.,1.,1.,1.,1.,1.,1.,1.,1.,1.,1.,1.,1.,
1.,1.,1.,1.,1.,1.,1.,1.,1.,1.,1.,1.,1.,1.,1.,1.,1.,1.,1.,1.,1.,1.,1.,1.,
1.,1.,1.,1.,1.,1.,1.,1.,1.,1.,1.,1.,1.,1.,1.,1.,1.,1.,1.,1.,1.,1.,1.,1.,
1.,1.,1.,1.,1.,1.))
REPRESENTATION_ITEM('')
);
#186=(
BOUNDED_CURVE()
B_SPLINE_CURVE(5,(#28559,#28560,#28561,#28562,#28563,#28564,#28565,#28566,
#28567,#28568,#28569,#28570,#28571,#28572,#28573,#28574,#28575,#28576,#28577,
#28578,#28579,#28580,#28581,#28582,#28583,#28584,#28585,#28586,#28587,#28588,
#28589,#28590,#28591,#28592,#28593,#28594,#28595,#28596,#28597,#28598,#28599,
#28600,#28601,#28602,#28603,#28604,#28605,#28606,#28607,#28608,#28609,#28610,
#28611,#28612,#28613,#28614,#28615,#28616,#28617,#28618,#28619,#28620,#28621,
#28622,#28623,#28624,#28625,#28626,#28627,#28628),.UNSPECIFIED.,.F.,.F.)
B_SPLINE_CURVE_WITH_KNOTS((6,1,1,1,1,1,1,1,1,1,1,1,1,1,1,1,1,1,1,1,1,1,
1,1,1,1,1,1,1,1,1,1,1,1,1,1,1,1,1,1,1,1,1,1,1,1,1,1,1,1,1,1,1,1,1,1,1,1,
1,1,1,1,1,1,1,6),(-1.,-0.984615384615383,-0.969230769230768,-0.953846153846152,
-0.938461538461537,-0.923076923076922,-0.907692307692306,-0.892307692307691,
-0.876923076923076,-0.86153846153846,-0.846153846153845,-0.83076923076923,
-0.815384615384614,-0.799999999999999,-0.784615384615384,-0.769230769230768,
-0.753846153846153,-0.738461538461538,-0.723076923076922,-0.707692307692307,
-0.692307692307692,-0.676923076923076,-0.661538461538461,-0.646153846153846,
-0.63076923076923,-0.615384615384615,-0.6,-0.584615384615384,-0.569230769230769,
-0.553846153846154,-0.538461538461538,-0.523076923076923,-0.507692307692308,
-0.492307692307692,-0.476923076923077,-0.461538461538462,-0.446153846153846,
-0.430769230769231,-0.415384615384615,-0.4,-0.384615384615385,-0.369230769230769,
-0.353846153846154,-0.338461538461538,-0.323076923076923,-0.307692307692308,
-0.292307692307692,-0.276923076923077,-0.261538461538462,-0.246153846153846,
-0.230769230769231,-0.215384615384615,-0.2,-0.184615384615385,-0.169230769230769,
-0.153846153846154,-0.138461538461538,-0.123076923076923,-0.107692307692308,
-0.0923076923076923,-0.0769230769230769,-0.0615384615384615,-0.0461538461538462,
-0.0307692307692308,-0.0153846153846154,0.),.UNSPECIFIED.)
CURVE()
GEOMETRIC_REPRESENTATION_ITEM()
RATIONAL_B_SPLINE_CURVE((1.,1.,1.,1.,1.,1.,1.,1.,1.,1.,1.,1.,1.,1.,1.,1.,
1.,1.,1.,1.,1.,1.,1.,1.,1.,1.,1.,1.,1.,1.,1.,1.,1.,1.,1.,1.,1.,1.,1.,1.,
1.,1.,1.,1.,1.,1.,1.,1.,1.,1.,1.,1.,1.,1.,1.,1.,1.,1.,1.,1.,1.,1.,1.,1.,
1.,1.,1.,1.,1.,1.))
REPRESENTATION_ITEM('')
);
#187=(
BOUNDED_CURVE()
B_SPLINE_CURVE(5,(#28775,#28776,#28777,#28778,#28779,#28780,#28781,#28782,
#28783,#28784,#28785,#28786,#28787,#28788,#28789,#28790,#28791,#28792,#28793,
#28794,#28795,#28796,#28797,#28798,#28799,#28800,#28801,#28802,#28803,#28804,
#28805,#28806,#28807,#28808,#28809,#28810,#28811,#28812,#28813,#28814,#28815,
#28816,#28817,#28818,#28819,#28820,#28821,#28822,#28823,#28824,#28825,#28826,
#28827,#28828,#28829,#28830,#28831,#28832,#28833,#28834,#28835,#28836,#28837,
#28838,#28839,#28840,#28841,#28842,#28843,#28844),.UNSPECIFIED.,.F.,.F.)
B_SPLINE_CURVE_WITH_KNOTS((6,1,1,1,1,1,1,1,1,1,1,1,1,1,1,1,1,1,1,1,1,1,
1,1,1,1,1,1,1,1,1,1,1,1,1,1,1,1,1,1,1,1,1,1,1,1,1,1,1,1,1,1,1,1,1,1,1,1,
1,1,1,1,1,1,1,6),(-1.,-0.984615384615383,-0.969230769230768,-0.953846153846152,
-0.938461538461537,-0.923076923076922,-0.907692307692306,-0.892307692307691,
-0.876923076923076,-0.86153846153846,-0.846153846153845,-0.83076923076923,
-0.815384615384614,-0.799999999999999,-0.784615384615384,-0.769230769230768,
-0.753846153846153,-0.738461538461538,-0.723076923076922,-0.707692307692307,
-0.692307692307692,-0.676923076923076,-0.661538461538461,-0.646153846153846,
-0.63076923076923,-0.615384615384615,-0.6,-0.584615384615384,-0.569230769230769,
-0.553846153846154,-0.538461538461538,-0.523076923076923,-0.507692307692308,
-0.492307692307692,-0.476923076923077,-0.461538461538462,-0.446153846153846,
-0.430769230769231,-0.415384615384615,-0.4,-0.384615384615385,-0.369230769230769,
-0.353846153846154,-0.338461538461538,-0.323076923076923,-0.307692307692308,
-0.292307692307692,-0.276923076923077,-0.261538461538462,-0.246153846153846,
-0.230769230769231,-0.215384615384615,-0.2,-0.184615384615385,-0.169230769230769,
-0.153846153846154,-0.138461538461538,-0.123076923076923,-0.107692307692308,
-0.0923076923076923,-0.0769230769230769,-0.0615384615384615,-0.0461538461538462,
-0.0307692307692308,-0.0153846153846154,0.),.UNSPECIFIED.)
CURVE()
GEOMETRIC_REPRESENTATION_ITEM()
RATIONAL_B_SPLINE_CURVE((1.,1.,1.,1.,1.,1.,1.,1.,1.,1.,1.,1.,1.,1.,1.,1.,
1.,1.,1.,1.,1.,1.,1.,1.,1.,1.,1.,1.,1.,1.,1.,1.,1.,1.,1.,1.,1.,1.,1.,1.,
1.,1.,1.,1.,1.,1.,1.,1.,1.,1.,1.,1.,1.,1.,1.,1.,1.,1.,1.,1.,1.,1.,1.,1.,
1.,1.,1.,1.,1.,1.))
REPRESENTATION_ITEM('')
);
#188=(
BOUNDED_CURVE()
B_SPLINE_CURVE(5,(#28991,#28992,#28993,#28994,#28995,#28996,#28997,#28998,
#28999,#29000,#29001,#29002,#29003,#29004,#29005,#29006,#29007,#29008,#29009,
#29010,#29011,#29012,#29013,#29014,#29015,#29016,#29017,#29018,#29019,#29020,
#29021,#29022,#29023,#29024,#29025,#29026,#29027,#29028,#29029,#29030,#29031,
#29032,#29033,#29034,#29035,#29036,#29037,#29038,#29039,#29040,#29041,#29042,
#29043,#29044,#29045,#29046,#29047,#29048,#29049,#29050,#29051,#29052,#29053,
#29054,#29055,#29056,#29057,#29058,#29059,#29060),.UNSPECIFIED.,.F.,.F.)
B_SPLINE_CURVE_WITH_KNOTS((6,1,1,1,1,1,1,1,1,1,1,1,1,1,1,1,1,1,1,1,1,1,
1,1,1,1,1,1,1,1,1,1,1,1,1,1,1,1,1,1,1,1,1,1,1,1,1,1,1,1,1,1,1,1,1,1,1,1,
1,1,1,1,1,1,1,6),(-1.,-0.984615384615383,-0.969230769230768,-0.953846153846152,
-0.938461538461537,-0.923076923076922,-0.907692307692306,-0.892307692307691,
-0.876923076923076,-0.86153846153846,-0.846153846153845,-0.83076923076923,
-0.815384615384614,-0.799999999999999,-0.784615384615384,-0.769230769230768,
-0.753846153846153,-0.738461538461538,-0.723076923076922,-0.707692307692307,
-0.692307692307692,-0.676923076923076,-0.661538461538461,-0.646153846153846,
-0.63076923076923,-0.615384615384615,-0.6,-0.584615384615384,-0.569230769230769,
-0.553846153846154,-0.538461538461538,-0.523076923076923,-0.507692307692308,
-0.492307692307692,-0.476923076923077,-0.461538461538462,-0.446153846153846,
-0.430769230769231,-0.415384615384615,-0.4,-0.384615384615385,-0.369230769230769,
-0.353846153846154,-0.338461538461538,-0.323076923076923,-0.307692307692308,
-0.292307692307692,-0.276923076923077,-0.261538461538462,-0.246153846153846,
-0.230769230769231,-0.215384615384615,-0.2,-0.184615384615385,-0.169230769230769,
-0.153846153846154,-0.138461538461538,-0.123076923076923,-0.107692307692308,
-0.0923076923076923,-0.0769230769230769,-0.0615384615384615,-0.0461538461538462,
-0.0307692307692308,-0.0153846153846154,0.),.UNSPECIFIED.)
CURVE()
GEOMETRIC_REPRESENTATION_ITEM()
RATIONAL_B_SPLINE_CURVE((1.,1.,1.,1.,1.,1.,1.,1.,1.,1.,1.,1.,1.,1.,1.,1.,
1.,1.,1.,1.,1.,1.,1.,1.,1.,1.,1.,1.,1.,1.,1.,1.,1.,1.,1.,1.,1.,1.,1.,1.,
1.,1.,1.,1.,1.,1.,1.,1.,1.,1.,1.,1.,1.,1.,1.,1.,1.,1.,1.,1.,1.,1.,1.,1.,
1.,1.,1.,1.,1.,1.))
REPRESENTATION_ITEM('')
);
#189=(
BOUNDED_CURVE()
B_SPLINE_CURVE(5,(#29207,#29208,#29209,#29210,#29211,#29212,#29213,#29214,
#29215,#29216,#29217,#29218,#29219,#29220,#29221,#29222,#29223,#29224,#29225,
#29226,#29227,#29228,#29229,#29230,#29231,#29232,#29233,#29234,#29235,#29236,
#29237,#29238,#29239,#29240,#29241,#29242,#29243,#29244,#29245,#29246,#29247,
#29248,#29249,#29250,#29251,#29252,#29253,#29254,#29255,#29256,#29257,#29258,
#29259,#29260,#29261,#29262,#29263,#29264,#29265,#29266,#29267,#29268,#29269,
#29270,#29271,#29272,#29273,#29274,#29275,#29276),.UNSPECIFIED.,.F.,.F.)
B_SPLINE_CURVE_WITH_KNOTS((6,1,1,1,1,1,1,1,1,1,1,1,1,1,1,1,1,1,1,1,1,1,
1,1,1,1,1,1,1,1,1,1,1,1,1,1,1,1,1,1,1,1,1,1,1,1,1,1,1,1,1,1,1,1,1,1,1,1,
1,1,1,1,1,1,1,6),(-1.,-0.984615384615383,-0.969230769230768,-0.953846153846152,
-0.938461538461537,-0.923076923076922,-0.907692307692306,-0.892307692307691,
-0.876923076923076,-0.86153846153846,-0.846153846153845,-0.83076923076923,
-0.815384615384614,-0.799999999999999,-0.784615384615384,-0.769230769230768,
-0.753846153846153,-0.738461538461538,-0.723076923076922,-0.707692307692307,
-0.692307692307692,-0.676923076923076,-0.661538461538461,-0.646153846153846,
-0.63076923076923,-0.615384615384615,-0.6,-0.584615384615384,-0.569230769230769,
-0.553846153846154,-0.538461538461538,-0.523076923076923,-0.507692307692308,
-0.492307692307692,-0.476923076923077,-0.461538461538462,-0.446153846153846,
-0.430769230769231,-0.415384615384615,-0.4,-0.384615384615385,-0.369230769230769,
-0.353846153846154,-0.338461538461538,-0.323076923076923,-0.307692307692308,
-0.292307692307692,-0.276923076923077,-0.261538461538462,-0.246153846153846,
-0.230769230769231,-0.215384615384615,-0.2,-0.184615384615385,-0.169230769230769,
-0.153846153846154,-0.138461538461538,-0.123076923076923,-0.107692307692308,
-0.0923076923076923,-0.0769230769230769,-0.0615384615384615,-0.0461538461538462,
-0.0307692307692308,-0.0153846153846154,0.),.UNSPECIFIED.)
CURVE()
GEOMETRIC_REPRESENTATION_ITEM()
RATIONAL_B_SPLINE_CURVE((1.,1.,1.,1.,1.,1.,1.,1.,1.,1.,1.,1.,1.,1.,1.,1.,
1.,1.,1.,1.,1.,1.,1.,1.,1.,1.,1.,1.,1.,1.,1.,1.,1.,1.,1.,1.,1.,1.,1.,1.,
1.,1.,1.,1.,1.,1.,1.,1.,1.,1.,1.,1.,1.,1.,1.,1.,1.,1.,1.,1.,1.,1.,1.,1.,
1.,1.,1.,1.,1.,1.))
REPRESENTATION_ITEM('')
);
#190=(
BOUNDED_CURVE()
B_SPLINE_CURVE(5,(#29423,#29424,#29425,#29426,#29427,#29428,#29429,#29430,
#29431,#29432,#29433,#29434,#29435,#29436,#29437,#29438,#29439,#29440,#29441,
#29442,#29443,#29444,#29445,#29446,#29447,#29448,#29449,#29450,#29451,#29452,
#29453,#29454,#29455,#29456,#29457,#29458,#29459,#29460,#29461,#29462,#29463,
#29464,#29465,#29466,#29467,#29468,#29469,#29470,#29471,#29472,#29473,#29474,
#29475,#29476,#29477,#29478,#29479,#29480,#29481,#29482,#29483,#29484,#29485,
#29486,#29487,#29488,#29489,#29490,#29491,#29492),.UNSPECIFIED.,.F.,.F.)
B_SPLINE_CURVE_WITH_KNOTS((6,1,1,1,1,1,1,1,1,1,1,1,1,1,1,1,1,1,1,1,1,1,
1,1,1,1,1,1,1,1,1,1,1,1,1,1,1,1,1,1,1,1,1,1,1,1,1,1,1,1,1,1,1,1,1,1,1,1,
1,1,1,1,1,1,1,6),(-1.,-0.984615384615383,-0.969230769230768,-0.953846153846152,
-0.938461538461537,-0.923076923076922,-0.907692307692306,-0.892307692307691,
-0.876923076923076,-0.86153846153846,-0.846153846153845,-0.83076923076923,
-0.815384615384614,-0.799999999999999,-0.784615384615384,-0.769230769230768,
-0.753846153846153,-0.738461538461538,-0.723076923076922,-0.707692307692307,
-0.692307692307692,-0.676923076923076,-0.661538461538461,-0.646153846153846,
-0.63076923076923,-0.615384615384615,-0.6,-0.584615384615384,-0.569230769230769,
-0.553846153846154,-0.538461538461538,-0.523076923076923,-0.507692307692308,
-0.492307692307692,-0.476923076923077,-0.461538461538462,-0.446153846153846,
-0.430769230769231,-0.415384615384615,-0.4,-0.384615384615385,-0.369230769230769,
-0.353846153846154,-0.338461538461538,-0.323076923076923,-0.307692307692308,
-0.292307692307692,-0.276923076923077,-0.261538461538462,-0.246153846153846,
-0.230769230769231,-0.215384615384615,-0.2,-0.184615384615385,-0.169230769230769,
-0.153846153846154,-0.138461538461538,-0.123076923076923,-0.107692307692308,
-0.0923076923076923,-0.0769230769230769,-0.0615384615384615,-0.0461538461538462,
-0.0307692307692308,-0.0153846153846154,0.),.UNSPECIFIED.)
CURVE()
GEOMETRIC_REPRESENTATION_ITEM()
RATIONAL_B_SPLINE_CURVE((1.,1.,1.,1.,1.,1.,1.,1.,1.,1.,1.,1.,1.,1.,1.,1.,
1.,1.,1.,1.,1.,1.,1.,1.,1.,1.,1.,1.,1.,1.,1.,1.,1.,1.,1.,1.,1.,1.,1.,1.,
1.,1.,1.,1.,1.,1.,1.,1.,1.,1.,1.,1.,1.,1.,1.,1.,1.,1.,1.,1.,1.,1.,1.,1.,
1.,1.,1.,1.,1.,1.))
REPRESENTATION_ITEM('')
);
#191=(
BOUNDED_CURVE()
B_SPLINE_CURVE(5,(#29639,#29640,#29641,#29642,#29643,#29644,#29645,#29646,
#29647,#29648,#29649,#29650,#29651,#29652,#29653,#29654,#29655,#29656,#29657,
#29658,#29659,#29660,#29661,#29662,#29663,#29664,#29665,#29666,#29667,#29668,
#29669,#29670,#29671,#29672,#29673,#29674,#29675,#29676,#29677,#29678,#29679,
#29680,#29681,#29682,#29683,#29684,#29685,#29686,#29687,#29688,#29689,#29690,
#29691,#29692,#29693,#29694,#29695,#29696,#29697,#29698,#29699,#29700,#29701,
#29702,#29703,#29704,#29705,#29706,#29707,#29708),.UNSPECIFIED.,.F.,.F.)
B_SPLINE_CURVE_WITH_KNOTS((6,1,1,1,1,1,1,1,1,1,1,1,1,1,1,1,1,1,1,1,1,1,
1,1,1,1,1,1,1,1,1,1,1,1,1,1,1,1,1,1,1,1,1,1,1,1,1,1,1,1,1,1,1,1,1,1,1,1,
1,1,1,1,1,1,1,6),(-1.,-0.984615384615383,-0.969230769230768,-0.953846153846152,
-0.938461538461537,-0.923076923076922,-0.907692307692306,-0.892307692307691,
-0.876923076923076,-0.86153846153846,-0.846153846153845,-0.83076923076923,
-0.815384615384614,-0.799999999999999,-0.784615384615384,-0.769230769230768,
-0.753846153846153,-0.738461538461538,-0.723076923076922,-0.707692307692307,
-0.692307692307692,-0.676923076923076,-0.661538461538461,-0.646153846153846,
-0.63076923076923,-0.615384615384615,-0.6,-0.584615384615384,-0.569230769230769,
-0.553846153846154,-0.538461538461538,-0.523076923076923,-0.507692307692308,
-0.492307692307692,-0.476923076923077,-0.461538461538462,-0.446153846153846,
-0.430769230769231,-0.415384615384615,-0.4,-0.384615384615385,-0.369230769230769,
-0.353846153846154,-0.338461538461538,-0.323076923076923,-0.307692307692308,
-0.292307692307692,-0.276923076923077,-0.261538461538462,-0.246153846153846,
-0.230769230769231,-0.215384615384615,-0.2,-0.184615384615385,-0.169230769230769,
-0.153846153846154,-0.138461538461538,-0.123076923076923,-0.107692307692308,
-0.0923076923076923,-0.0769230769230769,-0.0615384615384615,-0.0461538461538462,
-0.0307692307692308,-0.0153846153846154,0.),.UNSPECIFIED.)
CURVE()
GEOMETRIC_REPRESENTATION_ITEM()
RATIONAL_B_SPLINE_CURVE((1.,1.,1.,1.,1.,1.,1.,1.,1.,1.,1.,1.,1.,1.,1.,1.,
1.,1.,1.,1.,1.,1.,1.,1.,1.,1.,1.,1.,1.,1.,1.,1.,1.,1.,1.,1.,1.,1.,1.,1.,
1.,1.,1.,1.,1.,1.,1.,1.,1.,1.,1.,1.,1.,1.,1.,1.,1.,1.,1.,1.,1.,1.,1.,1.,
1.,1.,1.,1.,1.,1.))
REPRESENTATION_ITEM('')
);
#192=(
BOUNDED_CURVE()
B_SPLINE_CURVE(5,(#29855,#29856,#29857,#29858,#29859,#29860,#29861,#29862,
#29863,#29864,#29865,#29866,#29867,#29868,#29869,#29870,#29871,#29872,#29873,
#29874,#29875,#29876,#29877,#29878,#29879,#29880,#29881,#29882,#29883,#29884,
#29885,#29886,#29887,#29888,#29889,#29890,#29891,#29892,#29893,#29894,#29895,
#29896,#29897,#29898,#29899,#29900,#29901,#29902,#29903,#29904,#29905,#29906,
#29907,#29908,#29909,#29910,#29911,#29912,#29913,#29914,#29915,#29916,#29917,
#29918,#29919,#29920,#29921,#29922,#29923,#29924),.UNSPECIFIED.,.F.,.F.)
B_SPLINE_CURVE_WITH_KNOTS((6,1,1,1,1,1,1,1,1,1,1,1,1,1,1,1,1,1,1,1,1,1,
1,1,1,1,1,1,1,1,1,1,1,1,1,1,1,1,1,1,1,1,1,1,1,1,1,1,1,1,1,1,1,1,1,1,1,1,
1,1,1,1,1,1,1,6),(-1.,-0.984615384615383,-0.969230769230768,-0.953846153846152,
-0.938461538461537,-0.923076923076922,-0.907692307692306,-0.892307692307691,
-0.876923076923076,-0.86153846153846,-0.846153846153845,-0.83076923076923,
-0.815384615384614,-0.799999999999999,-0.784615384615384,-0.769230769230768,
-0.753846153846153,-0.738461538461538,-0.723076923076922,-0.707692307692307,
-0.692307692307692,-0.676923076923076,-0.661538461538461,-0.646153846153846,
-0.63076923076923,-0.615384615384615,-0.6,-0.584615384615384,-0.569230769230769,
-0.553846153846154,-0.538461538461538,-0.523076923076923,-0.507692307692308,
-0.492307692307692,-0.476923076923077,-0.461538461538462,-0.446153846153846,
-0.430769230769231,-0.415384615384615,-0.4,-0.384615384615385,-0.369230769230769,
-0.353846153846154,-0.338461538461538,-0.323076923076923,-0.307692307692308,
-0.292307692307692,-0.276923076923077,-0.261538461538462,-0.246153846153846,
-0.230769230769231,-0.215384615384615,-0.2,-0.184615384615385,-0.169230769230769,
-0.153846153846154,-0.138461538461538,-0.123076923076923,-0.107692307692308,
-0.0923076923076923,-0.0769230769230769,-0.0615384615384615,-0.0461538461538462,
-0.0307692307692308,-0.0153846153846154,0.),.UNSPECIFIED.)
CURVE()
GEOMETRIC_REPRESENTATION_ITEM()
RATIONAL_B_SPLINE_CURVE((1.,1.,1.,1.,1.,1.,1.,1.,1.,1.,1.,1.,1.,1.,1.,1.,
1.,1.,1.,1.,1.,1.,1.,1.,1.,1.,1.,1.,1.,1.,1.,1.,1.,1.,1.,1.,1.,1.,1.,1.,
1.,1.,1.,1.,1.,1.,1.,1.,1.,1.,1.,1.,1.,1.,1.,1.,1.,1.,1.,1.,1.,1.,1.,1.,
1.,1.,1.,1.,1.,1.))
REPRESENTATION_ITEM('')
);
#193=(
BOUNDED_CURVE()
B_SPLINE_CURVE(5,(#30071,#30072,#30073,#30074,#30075,#30076,#30077,#30078,
#30079,#30080,#30081,#30082,#30083,#30084,#30085,#30086,#30087,#30088,#30089,
#30090,#30091,#30092,#30093,#30094,#30095,#30096,#30097,#30098,#30099,#30100,
#30101,#30102,#30103,#30104,#30105,#30106,#30107,#30108,#30109,#30110,#30111,
#30112,#30113,#30114,#30115,#30116,#30117,#30118,#30119,#30120,#30121,#30122,
#30123,#30124,#30125,#30126,#30127,#30128,#30129,#30130,#30131,#30132,#30133,
#30134,#30135,#30136,#30137,#30138,#30139,#30140),.UNSPECIFIED.,.F.,.F.)
B_SPLINE_CURVE_WITH_KNOTS((6,1,1,1,1,1,1,1,1,1,1,1,1,1,1,1,1,1,1,1,1,1,
1,1,1,1,1,1,1,1,1,1,1,1,1,1,1,1,1,1,1,1,1,1,1,1,1,1,1,1,1,1,1,1,1,1,1,1,
1,1,1,1,1,1,1,6),(-1.,-0.984615384615383,-0.969230769230768,-0.953846153846152,
-0.938461538461537,-0.923076923076922,-0.907692307692306,-0.892307692307691,
-0.876923076923076,-0.86153846153846,-0.846153846153845,-0.83076923076923,
-0.815384615384614,-0.799999999999999,-0.784615384615384,-0.769230769230768,
-0.753846153846153,-0.738461538461538,-0.723076923076922,-0.707692307692307,
-0.692307692307692,-0.676923076923076,-0.661538461538461,-0.646153846153846,
-0.63076923076923,-0.615384615384615,-0.6,-0.584615384615384,-0.569230769230769,
-0.553846153846154,-0.538461538461538,-0.523076923076923,-0.507692307692308,
-0.492307692307692,-0.476923076923077,-0.461538461538462,-0.446153846153846,
-0.430769230769231,-0.415384615384615,-0.4,-0.384615384615385,-0.369230769230769,
-0.353846153846154,-0.338461538461538,-0.323076923076923,-0.307692307692308,
-0.292307692307692,-0.276923076923077,-0.261538461538462,-0.246153846153846,
-0.230769230769231,-0.215384615384615,-0.2,-0.184615384615385,-0.169230769230769,
-0.153846153846154,-0.138461538461538,-0.123076923076923,-0.107692307692308,
-0.0923076923076923,-0.0769230769230769,-0.0615384615384615,-0.0461538461538462,
-0.0307692307692308,-0.0153846153846154,0.),.UNSPECIFIED.)
CURVE()
GEOMETRIC_REPRESENTATION_ITEM()
RATIONAL_B_SPLINE_CURVE((1.,1.,1.,1.,1.,1.,1.,1.,1.,1.,1.,1.,1.,1.,1.,1.,
1.,1.,1.,1.,1.,1.,1.,1.,1.,1.,1.,1.,1.,1.,1.,1.,1.,1.,1.,1.,1.,1.,1.,1.,
1.,1.,1.,1.,1.,1.,1.,1.,1.,1.,1.,1.,1.,1.,1.,1.,1.,1.,1.,1.,1.,1.,1.,1.,
1.,1.,1.,1.,1.,1.))
REPRESENTATION_ITEM('')
);
#194=(
BOUNDED_CURVE()
B_SPLINE_CURVE(5,(#30287,#30288,#30289,#30290,#30291,#30292,#30293,#30294,
#30295,#30296,#30297,#30298,#30299,#30300,#30301,#30302,#30303,#30304,#30305,
#30306,#30307,#30308,#30309,#30310,#30311,#30312,#30313,#30314,#30315,#30316,
#30317,#30318,#30319,#30320,#30321,#30322,#30323,#30324,#30325,#30326,#30327,
#30328,#30329,#30330,#30331,#30332,#30333,#30334,#30335,#30336,#30337,#30338,
#30339,#30340,#30341,#30342,#30343,#30344,#30345,#30346,#30347,#30348,#30349,
#30350,#30351,#30352,#30353,#30354,#30355,#30356),.UNSPECIFIED.,.F.,.F.)
B_SPLINE_CURVE_WITH_KNOTS((6,1,1,1,1,1,1,1,1,1,1,1,1,1,1,1,1,1,1,1,1,1,
1,1,1,1,1,1,1,1,1,1,1,1,1,1,1,1,1,1,1,1,1,1,1,1,1,1,1,1,1,1,1,1,1,1,1,1,
1,1,1,1,1,1,1,6),(-1.,-0.984615384615383,-0.969230769230768,-0.953846153846152,
-0.938461538461537,-0.923076923076922,-0.907692307692306,-0.892307692307691,
-0.876923076923076,-0.86153846153846,-0.846153846153845,-0.83076923076923,
-0.815384615384614,-0.799999999999999,-0.784615384615384,-0.769230769230768,
-0.753846153846153,-0.738461538461538,-0.723076923076922,-0.707692307692307,
-0.692307692307692,-0.676923076923076,-0.661538461538461,-0.646153846153846,
-0.63076923076923,-0.615384615384615,-0.6,-0.584615384615384,-0.569230769230769,
-0.553846153846154,-0.538461538461538,-0.523076923076923,-0.507692307692308,
-0.492307692307692,-0.476923076923077,-0.461538461538462,-0.446153846153846,
-0.430769230769231,-0.415384615384615,-0.4,-0.384615384615385,-0.369230769230769,
-0.353846153846154,-0.338461538461538,-0.323076923076923,-0.307692307692308,
-0.292307692307692,-0.276923076923077,-0.261538461538462,-0.246153846153846,
-0.230769230769231,-0.215384615384615,-0.2,-0.184615384615385,-0.169230769230769,
-0.153846153846154,-0.138461538461538,-0.123076923076923,-0.107692307692308,
-0.0923076923076923,-0.0769230769230769,-0.0615384615384615,-0.0461538461538462,
-0.0307692307692308,-0.0153846153846154,0.),.UNSPECIFIED.)
CURVE()
GEOMETRIC_REPRESENTATION_ITEM()
RATIONAL_B_SPLINE_CURVE((1.,1.,1.,1.,1.,1.,1.,1.,1.,1.,1.,1.,1.,1.,1.,1.,
1.,1.,1.,1.,1.,1.,1.,1.,1.,1.,1.,1.,1.,1.,1.,1.,1.,1.,1.,1.,1.,1.,1.,1.,
1.,1.,1.,1.,1.,1.,1.,1.,1.,1.,1.,1.,1.,1.,1.,1.,1.,1.,1.,1.,1.,1.,1.,1.,
1.,1.,1.,1.,1.,1.))
REPRESENTATION_ITEM('')
);
#195=(
BOUNDED_CURVE()
B_SPLINE_CURVE(5,(#30503,#30504,#30505,#30506,#30507,#30508,#30509,#30510,
#30511,#30512,#30513,#30514,#30515,#30516,#30517,#30518,#30519,#30520,#30521,
#30522,#30523,#30524,#30525,#30526,#30527,#30528,#30529,#30530,#30531,#30532,
#30533,#30534,#30535,#30536,#30537,#30538,#30539,#30540,#30541,#30542,#30543,
#30544,#30545,#30546,#30547,#30548,#30549,#30550,#30551,#30552,#30553,#30554,
#30555,#30556,#30557,#30558,#30559,#30560,#30561,#30562,#30563,#30564,#30565,
#30566,#30567,#30568,#30569,#30570,#30571,#30572),.UNSPECIFIED.,.F.,.F.)
B_SPLINE_CURVE_WITH_KNOTS((6,1,1,1,1,1,1,1,1,1,1,1,1,1,1,1,1,1,1,1,1,1,
1,1,1,1,1,1,1,1,1,1,1,1,1,1,1,1,1,1,1,1,1,1,1,1,1,1,1,1,1,1,1,1,1,1,1,1,
1,1,1,1,1,1,1,6),(-1.,-0.984615384615383,-0.969230769230768,-0.953846153846152,
-0.938461538461537,-0.923076923076922,-0.907692307692306,-0.892307692307691,
-0.876923076923076,-0.86153846153846,-0.846153846153845,-0.83076923076923,
-0.815384615384614,-0.799999999999999,-0.784615384615384,-0.769230769230768,
-0.753846153846153,-0.738461538461538,-0.723076923076922,-0.707692307692307,
-0.692307692307692,-0.676923076923076,-0.661538461538461,-0.646153846153846,
-0.63076923076923,-0.615384615384615,-0.6,-0.584615384615384,-0.569230769230769,
-0.553846153846154,-0.538461538461538,-0.523076923076923,-0.507692307692308,
-0.492307692307692,-0.476923076923077,-0.461538461538462,-0.446153846153846,
-0.430769230769231,-0.415384615384615,-0.4,-0.384615384615385,-0.369230769230769,
-0.353846153846154,-0.338461538461538,-0.323076923076923,-0.307692307692308,
-0.292307692307692,-0.276923076923077,-0.261538461538462,-0.246153846153846,
-0.230769230769231,-0.215384615384615,-0.2,-0.184615384615385,-0.169230769230769,
-0.153846153846154,-0.138461538461538,-0.123076923076923,-0.107692307692308,
-0.0923076923076923,-0.0769230769230769,-0.0615384615384615,-0.0461538461538462,
-0.0307692307692308,-0.0153846153846154,0.),.UNSPECIFIED.)
CURVE()
GEOMETRIC_REPRESENTATION_ITEM()
RATIONAL_B_SPLINE_CURVE((1.,1.,1.,1.,1.,1.,1.,1.,1.,1.,1.,1.,1.,1.,1.,1.,
1.,1.,1.,1.,1.,1.,1.,1.,1.,1.,1.,1.,1.,1.,1.,1.,1.,1.,1.,1.,1.,1.,1.,1.,
1.,1.,1.,1.,1.,1.,1.,1.,1.,1.,1.,1.,1.,1.,1.,1.,1.,1.,1.,1.,1.,1.,1.,1.,
1.,1.,1.,1.,1.,1.))
REPRESENTATION_ITEM('')
);
#196=(
BOUNDED_CURVE()
B_SPLINE_CURVE(5,(#30719,#30720,#30721,#30722,#30723,#30724,#30725,#30726,
#30727,#30728,#30729,#30730,#30731,#30732,#30733,#30734,#30735,#30736,#30737,
#30738,#30739,#30740,#30741,#30742,#30743,#30744,#30745,#30746,#30747,#30748,
#30749,#30750,#30751,#30752,#30753,#30754,#30755,#30756,#30757,#30758,#30759,
#30760,#30761,#30762,#30763,#30764,#30765,#30766,#30767,#30768,#30769,#30770,
#30771,#30772,#30773,#30774,#30775,#30776,#30777,#30778,#30779,#30780,#30781,
#30782,#30783,#30784,#30785,#30786,#30787,#30788),.UNSPECIFIED.,.F.,.F.)
B_SPLINE_CURVE_WITH_KNOTS((6,1,1,1,1,1,1,1,1,1,1,1,1,1,1,1,1,1,1,1,1,1,
1,1,1,1,1,1,1,1,1,1,1,1,1,1,1,1,1,1,1,1,1,1,1,1,1,1,1,1,1,1,1,1,1,1,1,1,
1,1,1,1,1,1,1,6),(-1.,-0.984615384615383,-0.969230769230768,-0.953846153846152,
-0.938461538461537,-0.923076923076922,-0.907692307692306,-0.892307692307691,
-0.876923076923076,-0.86153846153846,-0.846153846153845,-0.83076923076923,
-0.815384615384614,-0.799999999999999,-0.784615384615384,-0.769230769230768,
-0.753846153846153,-0.738461538461538,-0.723076923076922,-0.707692307692307,
-0.692307692307692,-0.676923076923076,-0.661538461538461,-0.646153846153846,
-0.63076923076923,-0.615384615384615,-0.6,-0.584615384615384,-0.569230769230769,
-0.553846153846154,-0.538461538461538,-0.523076923076923,-0.507692307692308,
-0.492307692307692,-0.476923076923077,-0.461538461538462,-0.446153846153846,
-0.430769230769231,-0.415384615384615,-0.4,-0.384615384615385,-0.369230769230769,
-0.353846153846154,-0.338461538461538,-0.323076923076923,-0.307692307692308,
-0.292307692307692,-0.276923076923077,-0.261538461538462,-0.246153846153846,
-0.230769230769231,-0.215384615384615,-0.2,-0.184615384615385,-0.169230769230769,
-0.153846153846154,-0.138461538461538,-0.123076923076923,-0.107692307692308,
-0.0923076923076923,-0.0769230769230769,-0.0615384615384615,-0.0461538461538462,
-0.0307692307692308,-0.0153846153846154,0.),.UNSPECIFIED.)
CURVE()
GEOMETRIC_REPRESENTATION_ITEM()
RATIONAL_B_SPLINE_CURVE((1.,1.,1.,1.,1.,1.,1.,1.,1.,1.,1.,1.,1.,1.,1.,1.,
1.,1.,1.,1.,1.,1.,1.,1.,1.,1.,1.,1.,1.,1.,1.,1.,1.,1.,1.,1.,1.,1.,1.,1.,
1.,1.,1.,1.,1.,1.,1.,1.,1.,1.,1.,1.,1.,1.,1.,1.,1.,1.,1.,1.,1.,1.,1.,1.,
1.,1.,1.,1.,1.,1.))
REPRESENTATION_ITEM('')
);
#197=(
BOUNDED_CURVE()
B_SPLINE_CURVE(5,(#30935,#30936,#30937,#30938,#30939,#30940,#30941,#30942,
#30943,#30944,#30945,#30946,#30947,#30948,#30949,#30950,#30951,#30952,#30953,
#30954,#30955,#30956,#30957,#30958,#30959,#30960,#30961,#30962,#30963,#30964,
#30965,#30966,#30967,#30968,#30969,#30970,#30971,#30972,#30973,#30974,#30975,
#30976,#30977,#30978,#30979,#30980,#30981,#30982,#30983,#30984,#30985,#30986,
#30987,#30988,#30989,#30990,#30991,#30992,#30993,#30994,#30995,#30996,#30997,
#30998,#30999,#31000,#31001,#31002,#31003,#31004),.UNSPECIFIED.,.F.,.F.)
B_SPLINE_CURVE_WITH_KNOTS((6,1,1,1,1,1,1,1,1,1,1,1,1,1,1,1,1,1,1,1,1,1,
1,1,1,1,1,1,1,1,1,1,1,1,1,1,1,1,1,1,1,1,1,1,1,1,1,1,1,1,1,1,1,1,1,1,1,1,
1,1,1,1,1,1,1,6),(-1.,-0.984615384615383,-0.969230769230768,-0.953846153846152,
-0.938461538461537,-0.923076923076922,-0.907692307692306,-0.892307692307691,
-0.876923076923076,-0.86153846153846,-0.846153846153845,-0.83076923076923,
-0.815384615384614,-0.799999999999999,-0.784615384615384,-0.769230769230768,
-0.753846153846153,-0.738461538461538,-0.723076923076922,-0.707692307692307,
-0.692307692307692,-0.676923076923076,-0.661538461538461,-0.646153846153846,
-0.63076923076923,-0.615384615384615,-0.6,-0.584615384615384,-0.569230769230769,
-0.553846153846154,-0.538461538461538,-0.523076923076923,-0.507692307692308,
-0.492307692307692,-0.476923076923077,-0.461538461538462,-0.446153846153846,
-0.430769230769231,-0.415384615384615,-0.4,-0.384615384615385,-0.369230769230769,
-0.353846153846154,-0.338461538461538,-0.323076923076923,-0.307692307692308,
-0.292307692307692,-0.276923076923077,-0.261538461538462,-0.246153846153846,
-0.230769230769231,-0.215384615384615,-0.2,-0.184615384615385,-0.169230769230769,
-0.153846153846154,-0.138461538461538,-0.123076923076923,-0.107692307692308,
-0.0923076923076923,-0.0769230769230769,-0.0615384615384615,-0.0461538461538462,
-0.0307692307692308,-0.0153846153846154,0.),.UNSPECIFIED.)
CURVE()
GEOMETRIC_REPRESENTATION_ITEM()
RATIONAL_B_SPLINE_CURVE((1.,1.,1.,1.,1.,1.,1.,1.,1.,1.,1.,1.,1.,1.,1.,1.,
1.,1.,1.,1.,1.,1.,1.,1.,1.,1.,1.,1.,1.,1.,1.,1.,1.,1.,1.,1.,1.,1.,1.,1.,
1.,1.,1.,1.,1.,1.,1.,1.,1.,1.,1.,1.,1.,1.,1.,1.,1.,1.,1.,1.,1.,1.,1.,1.,
1.,1.,1.,1.,1.,1.))
REPRESENTATION_ITEM('')
);
#198=(
BOUNDED_CURVE()
B_SPLINE_CURVE(5,(#31151,#31152,#31153,#31154,#31155,#31156,#31157,#31158,
#31159,#31160,#31161,#31162,#31163,#31164,#31165,#31166,#31167,#31168,#31169,
#31170,#31171,#31172,#31173,#31174,#31175,#31176,#31177,#31178,#31179,#31180,
#31181,#31182,#31183,#31184,#31185,#31186,#31187,#31188,#31189,#31190,#31191,
#31192,#31193,#31194,#31195,#31196,#31197,#31198,#31199,#31200,#31201,#31202,
#31203,#31204,#31205,#31206,#31207,#31208,#31209,#31210,#31211,#31212,#31213,
#31214,#31215,#31216,#31217,#31218,#31219,#31220),.UNSPECIFIED.,.F.,.F.)
B_SPLINE_CURVE_WITH_KNOTS((6,1,1,1,1,1,1,1,1,1,1,1,1,1,1,1,1,1,1,1,1,1,
1,1,1,1,1,1,1,1,1,1,1,1,1,1,1,1,1,1,1,1,1,1,1,1,1,1,1,1,1,1,1,1,1,1,1,1,
1,1,1,1,1,1,1,6),(-1.,-0.984615384615383,-0.969230769230768,-0.953846153846152,
-0.938461538461537,-0.923076923076922,-0.907692307692306,-0.892307692307691,
-0.876923076923076,-0.86153846153846,-0.846153846153845,-0.83076923076923,
-0.815384615384614,-0.799999999999999,-0.784615384615384,-0.769230769230768,
-0.753846153846153,-0.738461538461538,-0.723076923076922,-0.707692307692307,
-0.692307692307692,-0.676923076923076,-0.661538461538461,-0.646153846153846,
-0.63076923076923,-0.615384615384615,-0.6,-0.584615384615384,-0.569230769230769,
-0.553846153846154,-0.538461538461538,-0.523076923076923,-0.507692307692308,
-0.492307692307692,-0.476923076923077,-0.461538461538462,-0.446153846153846,
-0.430769230769231,-0.415384615384615,-0.4,-0.384615384615385,-0.369230769230769,
-0.353846153846154,-0.338461538461538,-0.323076923076923,-0.307692307692308,
-0.292307692307692,-0.276923076923077,-0.261538461538462,-0.246153846153846,
-0.230769230769231,-0.215384615384615,-0.2,-0.184615384615385,-0.169230769230769,
-0.153846153846154,-0.138461538461538,-0.123076923076923,-0.107692307692308,
-0.0923076923076923,-0.0769230769230769,-0.0615384615384615,-0.0461538461538462,
-0.0307692307692308,-0.0153846153846154,0.),.UNSPECIFIED.)
CURVE()
GEOMETRIC_REPRESENTATION_ITEM()
RATIONAL_B_SPLINE_CURVE((1.,1.,1.,1.,1.,1.,1.,1.,1.,1.,1.,1.,1.,1.,1.,1.,
1.,1.,1.,1.,1.,1.,1.,1.,1.,1.,1.,1.,1.,1.,1.,1.,1.,1.,1.,1.,1.,1.,1.,1.,
1.,1.,1.,1.,1.,1.,1.,1.,1.,1.,1.,1.,1.,1.,1.,1.,1.,1.,1.,1.,1.,1.,1.,1.,
1.,1.,1.,1.,1.,1.))
REPRESENTATION_ITEM('')
);
#199=(
BOUNDED_CURVE()
B_SPLINE_CURVE(5,(#31367,#31368,#31369,#31370,#31371,#31372,#31373,#31374,
#31375,#31376,#31377,#31378,#31379,#31380,#31381,#31382,#31383,#31384,#31385,
#31386,#31387,#31388,#31389,#31390,#31391,#31392,#31393,#31394,#31395,#31396,
#31397,#31398,#31399,#31400,#31401,#31402,#31403,#31404,#31405,#31406,#31407,
#31408,#31409,#31410,#31411,#31412,#31413,#31414,#31415,#31416,#31417,#31418,
#31419,#31420,#31421,#31422,#31423,#31424,#31425,#31426,#31427,#31428,#31429,
#31430,#31431,#31432,#31433,#31434,#31435,#31436),.UNSPECIFIED.,.F.,.F.)
B_SPLINE_CURVE_WITH_KNOTS((6,1,1,1,1,1,1,1,1,1,1,1,1,1,1,1,1,1,1,1,1,1,
1,1,1,1,1,1,1,1,1,1,1,1,1,1,1,1,1,1,1,1,1,1,1,1,1,1,1,1,1,1,1,1,1,1,1,1,
1,1,1,1,1,1,1,6),(-1.,-0.984615384615383,-0.969230769230768,-0.953846153846152,
-0.938461538461537,-0.923076923076922,-0.907692307692306,-0.892307692307691,
-0.876923076923076,-0.86153846153846,-0.846153846153845,-0.83076923076923,
-0.815384615384614,-0.799999999999999,-0.784615384615384,-0.769230769230768,
-0.753846153846153,-0.738461538461538,-0.723076923076922,-0.707692307692307,
-0.692307692307692,-0.676923076923076,-0.661538461538461,-0.646153846153846,
-0.63076923076923,-0.615384615384615,-0.6,-0.584615384615384,-0.569230769230769,
-0.553846153846154,-0.538461538461538,-0.523076923076923,-0.507692307692308,
-0.492307692307692,-0.476923076923077,-0.461538461538462,-0.446153846153846,
-0.430769230769231,-0.415384615384615,-0.4,-0.384615384615385,-0.369230769230769,
-0.353846153846154,-0.338461538461538,-0.323076923076923,-0.307692307692308,
-0.292307692307692,-0.276923076923077,-0.261538461538462,-0.246153846153846,
-0.230769230769231,-0.215384615384615,-0.2,-0.184615384615385,-0.169230769230769,
-0.153846153846154,-0.138461538461538,-0.123076923076923,-0.107692307692308,
-0.0923076923076923,-0.0769230769230769,-0.0615384615384615,-0.0461538461538462,
-0.0307692307692308,-0.0153846153846154,0.),.UNSPECIFIED.)
CURVE()
GEOMETRIC_REPRESENTATION_ITEM()
RATIONAL_B_SPLINE_CURVE((1.,1.,1.,1.,1.,1.,1.,1.,1.,1.,1.,1.,1.,1.,1.,1.,
1.,1.,1.,1.,1.,1.,1.,1.,1.,1.,1.,1.,1.,1.,1.,1.,1.,1.,1.,1.,1.,1.,1.,1.,
1.,1.,1.,1.,1.,1.,1.,1.,1.,1.,1.,1.,1.,1.,1.,1.,1.,1.,1.,1.,1.,1.,1.,1.,
1.,1.,1.,1.,1.,1.))
REPRESENTATION_ITEM('')
);
#200=(
BOUNDED_CURVE()
B_SPLINE_CURVE(5,(#31583,#31584,#31585,#31586,#31587,#31588,#31589,#31590,
#31591,#31592,#31593,#31594,#31595,#31596,#31597,#31598,#31599,#31600,#31601,
#31602,#31603,#31604,#31605,#31606,#31607,#31608,#31609,#31610,#31611,#31612,
#31613,#31614,#31615,#31616,#31617,#31618,#31619,#31620,#31621,#31622,#31623,
#31624,#31625,#31626,#31627,#31628,#31629,#31630,#31631,#31632,#31633,#31634,
#31635,#31636,#31637,#31638,#31639,#31640,#31641,#31642,#31643,#31644,#31645,
#31646,#31647,#31648,#31649,#31650,#31651,#31652),.UNSPECIFIED.,.F.,.F.)
B_SPLINE_CURVE_WITH_KNOTS((6,1,1,1,1,1,1,1,1,1,1,1,1,1,1,1,1,1,1,1,1,1,
1,1,1,1,1,1,1,1,1,1,1,1,1,1,1,1,1,1,1,1,1,1,1,1,1,1,1,1,1,1,1,1,1,1,1,1,
1,1,1,1,1,1,1,6),(-1.,-0.984615384615383,-0.969230769230768,-0.953846153846152,
-0.938461538461537,-0.923076923076922,-0.907692307692306,-0.892307692307691,
-0.876923076923076,-0.86153846153846,-0.846153846153845,-0.83076923076923,
-0.815384615384614,-0.799999999999999,-0.784615384615384,-0.769230769230768,
-0.753846153846153,-0.738461538461538,-0.723076923076922,-0.707692307692307,
-0.692307692307692,-0.676923076923076,-0.661538461538461,-0.646153846153846,
-0.63076923076923,-0.615384615384615,-0.6,-0.584615384615384,-0.569230769230769,
-0.553846153846154,-0.538461538461538,-0.523076923076923,-0.507692307692308,
-0.492307692307692,-0.476923076923077,-0.461538461538462,-0.446153846153846,
-0.430769230769231,-0.415384615384615,-0.4,-0.384615384615385,-0.369230769230769,
-0.353846153846154,-0.338461538461538,-0.323076923076923,-0.307692307692308,
-0.292307692307692,-0.276923076923077,-0.261538461538462,-0.246153846153846,
-0.230769230769231,-0.215384615384615,-0.2,-0.184615384615385,-0.169230769230769,
-0.153846153846154,-0.138461538461538,-0.123076923076923,-0.107692307692308,
-0.0923076923076923,-0.0769230769230769,-0.0615384615384615,-0.0461538461538462,
-0.0307692307692308,-0.0153846153846154,0.),.UNSPECIFIED.)
CURVE()
GEOMETRIC_REPRESENTATION_ITEM()
RATIONAL_B_SPLINE_CURVE((1.,1.,1.,1.,1.,1.,1.,1.,1.,1.,1.,1.,1.,1.,1.,1.,
1.,1.,1.,1.,1.,1.,1.,1.,1.,1.,1.,1.,1.,1.,1.,1.,1.,1.,1.,1.,1.,1.,1.,1.,
1.,1.,1.,1.,1.,1.,1.,1.,1.,1.,1.,1.,1.,1.,1.,1.,1.,1.,1.,1.,1.,1.,1.,1.,
1.,1.,1.,1.,1.,1.))
REPRESENTATION_ITEM('')
);
#201=(
BOUNDED_CURVE()
B_SPLINE_CURVE(5,(#31799,#31800,#31801,#31802,#31803,#31804,#31805,#31806,
#31807,#31808,#31809,#31810,#31811,#31812,#31813,#31814,#31815,#31816,#31817,
#31818,#31819,#31820,#31821,#31822,#31823,#31824,#31825,#31826,#31827,#31828,
#31829,#31830,#31831,#31832,#31833,#31834,#31835,#31836,#31837,#31838,#31839,
#31840,#31841,#31842,#31843,#31844,#31845,#31846,#31847,#31848,#31849,#31850,
#31851,#31852,#31853,#31854,#31855,#31856,#31857,#31858,#31859,#31860,#31861,
#31862,#31863,#31864,#31865,#31866,#31867,#31868),.UNSPECIFIED.,.F.,.F.)
B_SPLINE_CURVE_WITH_KNOTS((6,1,1,1,1,1,1,1,1,1,1,1,1,1,1,1,1,1,1,1,1,1,
1,1,1,1,1,1,1,1,1,1,1,1,1,1,1,1,1,1,1,1,1,1,1,1,1,1,1,1,1,1,1,1,1,1,1,1,
1,1,1,1,1,1,1,6),(-1.,-0.984615384615383,-0.969230769230768,-0.953846153846152,
-0.938461538461537,-0.923076923076922,-0.907692307692306,-0.892307692307691,
-0.876923076923076,-0.86153846153846,-0.846153846153845,-0.83076923076923,
-0.815384615384614,-0.799999999999999,-0.784615384615384,-0.769230769230768,
-0.753846153846153,-0.738461538461538,-0.723076923076922,-0.707692307692307,
-0.692307692307692,-0.676923076923076,-0.661538461538461,-0.646153846153846,
-0.63076923076923,-0.615384615384615,-0.6,-0.584615384615384,-0.569230769230769,
-0.553846153846154,-0.538461538461538,-0.523076923076923,-0.507692307692308,
-0.492307692307692,-0.476923076923077,-0.461538461538462,-0.446153846153846,
-0.430769230769231,-0.415384615384615,-0.4,-0.384615384615385,-0.369230769230769,
-0.353846153846154,-0.338461538461538,-0.323076923076923,-0.307692307692308,
-0.292307692307692,-0.276923076923077,-0.261538461538462,-0.246153846153846,
-0.230769230769231,-0.215384615384615,-0.2,-0.184615384615385,-0.169230769230769,
-0.153846153846154,-0.138461538461538,-0.123076923076923,-0.107692307692308,
-0.0923076923076923,-0.0769230769230769,-0.0615384615384615,-0.0461538461538462,
-0.0307692307692308,-0.0153846153846154,0.),.UNSPECIFIED.)
CURVE()
GEOMETRIC_REPRESENTATION_ITEM()
RATIONAL_B_SPLINE_CURVE((1.,1.,1.,1.,1.,1.,1.,1.,1.,1.,1.,1.,1.,1.,1.,1.,
1.,1.,1.,1.,1.,1.,1.,1.,1.,1.,1.,1.,1.,1.,1.,1.,1.,1.,1.,1.,1.,1.,1.,1.,
1.,1.,1.,1.,1.,1.,1.,1.,1.,1.,1.,1.,1.,1.,1.,1.,1.,1.,1.,1.,1.,1.,1.,1.,
1.,1.,1.,1.,1.,1.))
REPRESENTATION_ITEM('')
);
#202=(
BOUNDED_CURVE()
B_SPLINE_CURVE(5,(#32015,#32016,#32017,#32018,#32019,#32020,#32021,#32022,
#32023,#32024,#32025,#32026,#32027,#32028,#32029,#32030,#32031,#32032,#32033,
#32034,#32035,#32036,#32037,#32038,#32039,#32040,#32041,#32042,#32043,#32044,
#32045,#32046,#32047,#32048,#32049,#32050,#32051,#32052,#32053,#32054,#32055,
#32056,#32057,#32058,#32059,#32060,#32061,#32062,#32063,#32064,#32065,#32066,
#32067,#32068,#32069,#32070,#32071,#32072,#32073,#32074,#32075,#32076,#32077,
#32078,#32079,#32080,#32081,#32082,#32083,#32084),.UNSPECIFIED.,.F.,.F.)
B_SPLINE_CURVE_WITH_KNOTS((6,1,1,1,1,1,1,1,1,1,1,1,1,1,1,1,1,1,1,1,1,1,
1,1,1,1,1,1,1,1,1,1,1,1,1,1,1,1,1,1,1,1,1,1,1,1,1,1,1,1,1,1,1,1,1,1,1,1,
1,1,1,1,1,1,1,6),(-1.,-0.984615384615383,-0.969230769230768,-0.953846153846152,
-0.938461538461537,-0.923076923076922,-0.907692307692306,-0.892307692307691,
-0.876923076923076,-0.86153846153846,-0.846153846153845,-0.83076923076923,
-0.815384615384614,-0.799999999999999,-0.784615384615384,-0.769230769230768,
-0.753846153846153,-0.738461538461538,-0.723076923076922,-0.707692307692307,
-0.692307692307692,-0.676923076923076,-0.661538461538461,-0.646153846153846,
-0.63076923076923,-0.615384615384615,-0.6,-0.584615384615384,-0.569230769230769,
-0.553846153846154,-0.538461538461538,-0.523076923076923,-0.507692307692308,
-0.492307692307692,-0.476923076923077,-0.461538461538462,-0.446153846153846,
-0.430769230769231,-0.415384615384615,-0.4,-0.384615384615385,-0.369230769230769,
-0.353846153846154,-0.338461538461538,-0.323076923076923,-0.307692307692308,
-0.292307692307692,-0.276923076923077,-0.261538461538462,-0.246153846153846,
-0.230769230769231,-0.215384615384615,-0.2,-0.184615384615385,-0.169230769230769,
-0.153846153846154,-0.138461538461538,-0.123076923076923,-0.107692307692308,
-0.0923076923076923,-0.0769230769230769,-0.0615384615384615,-0.0461538461538462,
-0.0307692307692308,-0.0153846153846154,0.),.UNSPECIFIED.)
CURVE()
GEOMETRIC_REPRESENTATION_ITEM()
RATIONAL_B_SPLINE_CURVE((1.,1.,1.,1.,1.,1.,1.,1.,1.,1.,1.,1.,1.,1.,1.,1.,
1.,1.,1.,1.,1.,1.,1.,1.,1.,1.,1.,1.,1.,1.,1.,1.,1.,1.,1.,1.,1.,1.,1.,1.,
1.,1.,1.,1.,1.,1.,1.,1.,1.,1.,1.,1.,1.,1.,1.,1.,1.,1.,1.,1.,1.,1.,1.,1.,
1.,1.,1.,1.,1.,1.))
REPRESENTATION_ITEM('')
);
#203=(
BOUNDED_CURVE()
B_SPLINE_CURVE(5,(#32231,#32232,#32233,#32234,#32235,#32236,#32237,#32238,
#32239,#32240,#32241,#32242,#32243,#32244,#32245,#32246,#32247,#32248,#32249,
#32250,#32251,#32252,#32253,#32254,#32255,#32256,#32257,#32258,#32259,#32260,
#32261,#32262,#32263,#32264,#32265,#32266,#32267,#32268,#32269,#32270,#32271,
#32272,#32273,#32274,#32275,#32276,#32277,#32278,#32279,#32280,#32281,#32282,
#32283,#32284,#32285,#32286,#32287,#32288,#32289,#32290,#32291,#32292,#32293,
#32294,#32295,#32296,#32297,#32298,#32299,#32300),.UNSPECIFIED.,.F.,.F.)
B_SPLINE_CURVE_WITH_KNOTS((6,1,1,1,1,1,1,1,1,1,1,1,1,1,1,1,1,1,1,1,1,1,
1,1,1,1,1,1,1,1,1,1,1,1,1,1,1,1,1,1,1,1,1,1,1,1,1,1,1,1,1,1,1,1,1,1,1,1,
1,1,1,1,1,1,1,6),(-1.,-0.984615384615383,-0.969230769230768,-0.953846153846152,
-0.938461538461537,-0.923076923076922,-0.907692307692306,-0.892307692307691,
-0.876923076923076,-0.86153846153846,-0.846153846153845,-0.83076923076923,
-0.815384615384614,-0.799999999999999,-0.784615384615384,-0.769230769230768,
-0.753846153846153,-0.738461538461538,-0.723076923076922,-0.707692307692307,
-0.692307692307692,-0.676923076923076,-0.661538461538461,-0.646153846153846,
-0.63076923076923,-0.615384615384615,-0.6,-0.584615384615384,-0.569230769230769,
-0.553846153846154,-0.538461538461538,-0.523076923076923,-0.507692307692308,
-0.492307692307692,-0.476923076923077,-0.461538461538462,-0.446153846153846,
-0.430769230769231,-0.415384615384615,-0.4,-0.384615384615385,-0.369230769230769,
-0.353846153846154,-0.338461538461538,-0.323076923076923,-0.307692307692308,
-0.292307692307692,-0.276923076923077,-0.261538461538462,-0.246153846153846,
-0.230769230769231,-0.215384615384615,-0.2,-0.184615384615385,-0.169230769230769,
-0.153846153846154,-0.138461538461538,-0.123076923076923,-0.107692307692308,
-0.0923076923076923,-0.0769230769230769,-0.0615384615384615,-0.0461538461538462,
-0.0307692307692308,-0.0153846153846154,0.),.UNSPECIFIED.)
CURVE()
GEOMETRIC_REPRESENTATION_ITEM()
RATIONAL_B_SPLINE_CURVE((1.,1.,1.,1.,1.,1.,1.,1.,1.,1.,1.,1.,1.,1.,1.,1.,
1.,1.,1.,1.,1.,1.,1.,1.,1.,1.,1.,1.,1.,1.,1.,1.,1.,1.,1.,1.,1.,1.,1.,1.,
1.,1.,1.,1.,1.,1.,1.,1.,1.,1.,1.,1.,1.,1.,1.,1.,1.,1.,1.,1.,1.,1.,1.,1.,
1.,1.,1.,1.,1.,1.))
REPRESENTATION_ITEM('')
);
#204=(
BOUNDED_CURVE()
B_SPLINE_CURVE(5,(#32447,#32448,#32449,#32450,#32451,#32452,#32453,#32454,
#32455,#32456,#32457,#32458,#32459,#32460,#32461,#32462,#32463,#32464,#32465,
#32466,#32467,#32468,#32469,#32470,#32471,#32472,#32473,#32474,#32475,#32476,
#32477,#32478,#32479,#32480,#32481,#32482,#32483,#32484,#32485,#32486,#32487,
#32488,#32489,#32490,#32491,#32492,#32493,#32494,#32495,#32496,#32497,#32498,
#32499,#32500,#32501,#32502,#32503,#32504,#32505,#32506,#32507,#32508,#32509,
#32510,#32511,#32512,#32513,#32514,#32515,#32516),.UNSPECIFIED.,.F.,.F.)
B_SPLINE_CURVE_WITH_KNOTS((6,1,1,1,1,1,1,1,1,1,1,1,1,1,1,1,1,1,1,1,1,1,
1,1,1,1,1,1,1,1,1,1,1,1,1,1,1,1,1,1,1,1,1,1,1,1,1,1,1,1,1,1,1,1,1,1,1,1,
1,1,1,1,1,1,1,6),(-1.,-0.984615384615383,-0.969230769230768,-0.953846153846152,
-0.938461538461537,-0.923076923076922,-0.907692307692306,-0.892307692307691,
-0.876923076923076,-0.86153846153846,-0.846153846153845,-0.83076923076923,
-0.815384615384614,-0.799999999999999,-0.784615384615384,-0.769230769230768,
-0.753846153846153,-0.738461538461538,-0.723076923076922,-0.707692307692307,
-0.692307692307692,-0.676923076923076,-0.661538461538461,-0.646153846153846,
-0.63076923076923,-0.615384615384615,-0.6,-0.584615384615384,-0.569230769230769,
-0.553846153846154,-0.538461538461538,-0.523076923076923,-0.507692307692308,
-0.492307692307692,-0.476923076923077,-0.461538461538462,-0.446153846153846,
-0.430769230769231,-0.415384615384615,-0.4,-0.384615384615385,-0.369230769230769,
-0.353846153846154,-0.338461538461538,-0.323076923076923,-0.307692307692308,
-0.292307692307692,-0.276923076923077,-0.261538461538462,-0.246153846153846,
-0.230769230769231,-0.215384615384615,-0.2,-0.184615384615385,-0.169230769230769,
-0.153846153846154,-0.138461538461538,-0.123076923076923,-0.107692307692308,
-0.0923076923076923,-0.0769230769230769,-0.0615384615384615,-0.0461538461538462,
-0.0307692307692308,-0.0153846153846154,0.),.UNSPECIFIED.)
CURVE()
GEOMETRIC_REPRESENTATION_ITEM()
RATIONAL_B_SPLINE_CURVE((1.,1.,1.,1.,1.,1.,1.,1.,1.,1.,1.,1.,1.,1.,1.,1.,
1.,1.,1.,1.,1.,1.,1.,1.,1.,1.,1.,1.,1.,1.,1.,1.,1.,1.,1.,1.,1.,1.,1.,1.,
1.,1.,1.,1.,1.,1.,1.,1.,1.,1.,1.,1.,1.,1.,1.,1.,1.,1.,1.,1.,1.,1.,1.,1.,
1.,1.,1.,1.,1.,1.))
REPRESENTATION_ITEM('')
);
#205=(
BOUNDED_CURVE()
B_SPLINE_CURVE(5,(#32663,#32664,#32665,#32666,#32667,#32668,#32669,#32670,
#32671,#32672,#32673,#32674,#32675,#32676,#32677,#32678,#32679,#32680,#32681,
#32682,#32683,#32684,#32685,#32686,#32687,#32688,#32689,#32690,#32691,#32692,
#32693,#32694,#32695,#32696,#32697,#32698,#32699,#32700,#32701,#32702,#32703,
#32704,#32705,#32706,#32707,#32708,#32709,#32710,#32711,#32712,#32713,#32714,
#32715,#32716,#32717,#32718,#32719,#32720,#32721,#32722,#32723,#32724,#32725,
#32726,#32727,#32728,#32729,#32730,#32731,#32732),.UNSPECIFIED.,.F.,.F.)
B_SPLINE_CURVE_WITH_KNOTS((6,1,1,1,1,1,1,1,1,1,1,1,1,1,1,1,1,1,1,1,1,1,
1,1,1,1,1,1,1,1,1,1,1,1,1,1,1,1,1,1,1,1,1,1,1,1,1,1,1,1,1,1,1,1,1,1,1,1,
1,1,1,1,1,1,1,6),(-1.,-0.984615384615383,-0.969230769230768,-0.953846153846152,
-0.938461538461537,-0.923076923076922,-0.907692307692306,-0.892307692307691,
-0.876923076923076,-0.86153846153846,-0.846153846153845,-0.83076923076923,
-0.815384615384614,-0.799999999999999,-0.784615384615384,-0.769230769230768,
-0.753846153846153,-0.738461538461538,-0.723076923076922,-0.707692307692307,
-0.692307692307692,-0.676923076923076,-0.661538461538461,-0.646153846153846,
-0.63076923076923,-0.615384615384615,-0.6,-0.584615384615384,-0.569230769230769,
-0.553846153846154,-0.538461538461538,-0.523076923076923,-0.507692307692308,
-0.492307692307692,-0.476923076923077,-0.461538461538462,-0.446153846153846,
-0.430769230769231,-0.415384615384615,-0.4,-0.384615384615385,-0.369230769230769,
-0.353846153846154,-0.338461538461538,-0.323076923076923,-0.307692307692308,
-0.292307692307692,-0.276923076923077,-0.261538461538462,-0.246153846153846,
-0.230769230769231,-0.215384615384615,-0.2,-0.184615384615385,-0.169230769230769,
-0.153846153846154,-0.138461538461538,-0.123076923076923,-0.107692307692308,
-0.0923076923076923,-0.0769230769230769,-0.0615384615384615,-0.0461538461538462,
-0.0307692307692308,-0.0153846153846154,0.),.UNSPECIFIED.)
CURVE()
GEOMETRIC_REPRESENTATION_ITEM()
RATIONAL_B_SPLINE_CURVE((1.,1.,1.,1.,1.,1.,1.,1.,1.,1.,1.,1.,1.,1.,1.,1.,
1.,1.,1.,1.,1.,1.,1.,1.,1.,1.,1.,1.,1.,1.,1.,1.,1.,1.,1.,1.,1.,1.,1.,1.,
1.,1.,1.,1.,1.,1.,1.,1.,1.,1.,1.,1.,1.,1.,1.,1.,1.,1.,1.,1.,1.,1.,1.,1.,
1.,1.,1.,1.,1.,1.))
REPRESENTATION_ITEM('')
);
#206=(
BOUNDED_CURVE()
B_SPLINE_CURVE(5,(#32879,#32880,#32881,#32882,#32883,#32884,#32885,#32886,
#32887,#32888,#32889,#32890,#32891,#32892,#32893,#32894,#32895,#32896,#32897,
#32898,#32899,#32900,#32901,#32902,#32903,#32904,#32905,#32906,#32907,#32908,
#32909,#32910,#32911,#32912,#32913,#32914,#32915,#32916,#32917,#32918,#32919,
#32920,#32921,#32922,#32923,#32924,#32925,#32926,#32927,#32928,#32929,#32930,
#32931,#32932,#32933,#32934,#32935,#32936,#32937,#32938,#32939,#32940,#32941,
#32942,#32943,#32944,#32945,#32946,#32947,#32948),.UNSPECIFIED.,.F.,.F.)
B_SPLINE_CURVE_WITH_KNOTS((6,1,1,1,1,1,1,1,1,1,1,1,1,1,1,1,1,1,1,1,1,1,
1,1,1,1,1,1,1,1,1,1,1,1,1,1,1,1,1,1,1,1,1,1,1,1,1,1,1,1,1,1,1,1,1,1,1,1,
1,1,1,1,1,1,1,6),(-1.,-0.984615384615383,-0.969230769230768,-0.953846153846152,
-0.938461538461537,-0.923076923076922,-0.907692307692306,-0.892307692307691,
-0.876923076923076,-0.86153846153846,-0.846153846153845,-0.83076923076923,
-0.815384615384614,-0.799999999999999,-0.784615384615384,-0.769230769230768,
-0.753846153846153,-0.738461538461538,-0.723076923076922,-0.707692307692307,
-0.692307692307692,-0.676923076923076,-0.661538461538461,-0.646153846153846,
-0.63076923076923,-0.615384615384615,-0.6,-0.584615384615384,-0.569230769230769,
-0.553846153846154,-0.538461538461538,-0.523076923076923,-0.507692307692308,
-0.492307692307692,-0.476923076923077,-0.461538461538462,-0.446153846153846,
-0.430769230769231,-0.415384615384615,-0.4,-0.384615384615385,-0.369230769230769,
-0.353846153846154,-0.338461538461538,-0.323076923076923,-0.307692307692308,
-0.292307692307692,-0.276923076923077,-0.261538461538462,-0.246153846153846,
-0.230769230769231,-0.215384615384615,-0.2,-0.184615384615385,-0.169230769230769,
-0.153846153846154,-0.138461538461538,-0.123076923076923,-0.107692307692308,
-0.0923076923076923,-0.0769230769230769,-0.0615384615384615,-0.0461538461538462,
-0.0307692307692308,-0.0153846153846154,0.),.UNSPECIFIED.)
CURVE()
GEOMETRIC_REPRESENTATION_ITEM()
RATIONAL_B_SPLINE_CURVE((1.,1.,1.,1.,1.,1.,1.,1.,1.,1.,1.,1.,1.,1.,1.,1.,
1.,1.,1.,1.,1.,1.,1.,1.,1.,1.,1.,1.,1.,1.,1.,1.,1.,1.,1.,1.,1.,1.,1.,1.,
1.,1.,1.,1.,1.,1.,1.,1.,1.,1.,1.,1.,1.,1.,1.,1.,1.,1.,1.,1.,1.,1.,1.,1.,
1.,1.,1.,1.,1.,1.))
REPRESENTATION_ITEM('')
);
#207=(
BOUNDED_CURVE()
B_SPLINE_CURVE(5,(#33095,#33096,#33097,#33098,#33099,#33100,#33101,#33102,
#33103,#33104,#33105,#33106,#33107,#33108,#33109,#33110,#33111,#33112,#33113,
#33114,#33115,#33116,#33117,#33118,#33119,#33120,#33121,#33122,#33123,#33124,
#33125,#33126,#33127,#33128,#33129,#33130,#33131,#33132,#33133,#33134,#33135,
#33136,#33137,#33138,#33139,#33140,#33141,#33142,#33143,#33144,#33145,#33146,
#33147,#33148,#33149,#33150,#33151,#33152,#33153,#33154,#33155,#33156,#33157,
#33158,#33159,#33160,#33161,#33162,#33163,#33164),.UNSPECIFIED.,.F.,.F.)
B_SPLINE_CURVE_WITH_KNOTS((6,1,1,1,1,1,1,1,1,1,1,1,1,1,1,1,1,1,1,1,1,1,
1,1,1,1,1,1,1,1,1,1,1,1,1,1,1,1,1,1,1,1,1,1,1,1,1,1,1,1,1,1,1,1,1,1,1,1,
1,1,1,1,1,1,1,6),(-1.,-0.984615384615383,-0.969230769230768,-0.953846153846152,
-0.938461538461537,-0.923076923076922,-0.907692307692306,-0.892307692307691,
-0.876923076923076,-0.86153846153846,-0.846153846153845,-0.83076923076923,
-0.815384615384614,-0.799999999999999,-0.784615384615384,-0.769230769230768,
-0.753846153846153,-0.738461538461538,-0.723076923076922,-0.707692307692307,
-0.692307692307692,-0.676923076923076,-0.661538461538461,-0.646153846153846,
-0.63076923076923,-0.615384615384615,-0.6,-0.584615384615384,-0.569230769230769,
-0.553846153846154,-0.538461538461538,-0.523076923076923,-0.507692307692308,
-0.492307692307692,-0.476923076923077,-0.461538461538462,-0.446153846153846,
-0.430769230769231,-0.415384615384615,-0.4,-0.384615384615385,-0.369230769230769,
-0.353846153846154,-0.338461538461538,-0.323076923076923,-0.307692307692308,
-0.292307692307692,-0.276923076923077,-0.261538461538462,-0.246153846153846,
-0.230769230769231,-0.215384615384615,-0.2,-0.184615384615385,-0.169230769230769,
-0.153846153846154,-0.138461538461538,-0.123076923076923,-0.107692307692308,
-0.0923076923076923,-0.0769230769230769,-0.0615384615384615,-0.0461538461538462,
-0.0307692307692308,-0.0153846153846154,0.),.UNSPECIFIED.)
CURVE()
GEOMETRIC_REPRESENTATION_ITEM()
RATIONAL_B_SPLINE_CURVE((1.,1.,1.,1.,1.,1.,1.,1.,1.,1.,1.,1.,1.,1.,1.,1.,
1.,1.,1.,1.,1.,1.,1.,1.,1.,1.,1.,1.,1.,1.,1.,1.,1.,1.,1.,1.,1.,1.,1.,1.,
1.,1.,1.,1.,1.,1.,1.,1.,1.,1.,1.,1.,1.,1.,1.,1.,1.,1.,1.,1.,1.,1.,1.,1.,
1.,1.,1.,1.,1.,1.))
REPRESENTATION_ITEM('')
);
#208=(
BOUNDED_CURVE()
B_SPLINE_CURVE(5,(#33311,#33312,#33313,#33314,#33315,#33316,#33317,#33318,
#33319,#33320,#33321,#33322,#33323,#33324,#33325,#33326,#33327,#33328,#33329,
#33330,#33331,#33332,#33333,#33334,#33335,#33336,#33337,#33338,#33339,#33340,
#33341,#33342,#33343,#33344,#33345,#33346,#33347,#33348,#33349,#33350,#33351,
#33352,#33353,#33354,#33355,#33356,#33357,#33358,#33359,#33360,#33361,#33362,
#33363,#33364,#33365,#33366,#33367,#33368,#33369,#33370,#33371,#33372,#33373,
#33374,#33375,#33376,#33377,#33378,#33379,#33380),.UNSPECIFIED.,.F.,.F.)
B_SPLINE_CURVE_WITH_KNOTS((6,1,1,1,1,1,1,1,1,1,1,1,1,1,1,1,1,1,1,1,1,1,
1,1,1,1,1,1,1,1,1,1,1,1,1,1,1,1,1,1,1,1,1,1,1,1,1,1,1,1,1,1,1,1,1,1,1,1,
1,1,1,1,1,1,1,6),(-1.,-0.984615384615383,-0.969230769230768,-0.953846153846152,
-0.938461538461537,-0.923076923076922,-0.907692307692306,-0.892307692307691,
-0.876923076923076,-0.86153846153846,-0.846153846153845,-0.83076923076923,
-0.815384615384614,-0.799999999999999,-0.784615384615384,-0.769230769230768,
-0.753846153846153,-0.738461538461538,-0.723076923076922,-0.707692307692307,
-0.692307692307692,-0.676923076923076,-0.661538461538461,-0.646153846153846,
-0.63076923076923,-0.615384615384615,-0.6,-0.584615384615384,-0.569230769230769,
-0.553846153846154,-0.538461538461538,-0.523076923076923,-0.507692307692308,
-0.492307692307692,-0.476923076923077,-0.461538461538462,-0.446153846153846,
-0.430769230769231,-0.415384615384615,-0.4,-0.384615384615385,-0.369230769230769,
-0.353846153846154,-0.338461538461538,-0.323076923076923,-0.307692307692308,
-0.292307692307692,-0.276923076923077,-0.261538461538462,-0.246153846153846,
-0.230769230769231,-0.215384615384615,-0.2,-0.184615384615385,-0.169230769230769,
-0.153846153846154,-0.138461538461538,-0.123076923076923,-0.107692307692308,
-0.0923076923076923,-0.0769230769230769,-0.0615384615384615,-0.0461538461538462,
-0.0307692307692308,-0.0153846153846154,0.),.UNSPECIFIED.)
CURVE()
GEOMETRIC_REPRESENTATION_ITEM()
RATIONAL_B_SPLINE_CURVE((1.,1.,1.,1.,1.,1.,1.,1.,1.,1.,1.,1.,1.,1.,1.,1.,
1.,1.,1.,1.,1.,1.,1.,1.,1.,1.,1.,1.,1.,1.,1.,1.,1.,1.,1.,1.,1.,1.,1.,1.,
1.,1.,1.,1.,1.,1.,1.,1.,1.,1.,1.,1.,1.,1.,1.,1.,1.,1.,1.,1.,1.,1.,1.,1.,
1.,1.,1.,1.,1.,1.))
REPRESENTATION_ITEM('')
);
#209=(
BOUNDED_CURVE()
B_SPLINE_CURVE(5,(#33527,#33528,#33529,#33530,#33531,#33532,#33533,#33534,
#33535,#33536,#33537,#33538,#33539,#33540,#33541,#33542,#33543,#33544,#33545,
#33546,#33547,#33548,#33549,#33550,#33551,#33552,#33553,#33554,#33555,#33556,
#33557,#33558,#33559,#33560,#33561,#33562,#33563,#33564,#33565,#33566,#33567,
#33568,#33569,#33570,#33571,#33572,#33573,#33574,#33575,#33576,#33577,#33578,
#33579,#33580,#33581,#33582,#33583,#33584,#33585,#33586,#33587,#33588,#33589,
#33590,#33591,#33592,#33593,#33594,#33595,#33596),.UNSPECIFIED.,.F.,.F.)
B_SPLINE_CURVE_WITH_KNOTS((6,1,1,1,1,1,1,1,1,1,1,1,1,1,1,1,1,1,1,1,1,1,
1,1,1,1,1,1,1,1,1,1,1,1,1,1,1,1,1,1,1,1,1,1,1,1,1,1,1,1,1,1,1,1,1,1,1,1,
1,1,1,1,1,1,1,6),(-1.,-0.984615384615383,-0.969230769230768,-0.953846153846152,
-0.938461538461537,-0.923076923076922,-0.907692307692306,-0.892307692307691,
-0.876923076923076,-0.86153846153846,-0.846153846153845,-0.83076923076923,
-0.815384615384614,-0.799999999999999,-0.784615384615384,-0.769230769230768,
-0.753846153846153,-0.738461538461538,-0.723076923076922,-0.707692307692307,
-0.692307692307692,-0.676923076923076,-0.661538461538461,-0.646153846153846,
-0.63076923076923,-0.615384615384615,-0.6,-0.584615384615384,-0.569230769230769,
-0.553846153846154,-0.538461538461538,-0.523076923076923,-0.507692307692308,
-0.492307692307692,-0.476923076923077,-0.461538461538462,-0.446153846153846,
-0.430769230769231,-0.415384615384615,-0.4,-0.384615384615385,-0.369230769230769,
-0.353846153846154,-0.338461538461538,-0.323076923076923,-0.307692307692308,
-0.292307692307692,-0.276923076923077,-0.261538461538462,-0.246153846153846,
-0.230769230769231,-0.215384615384615,-0.2,-0.184615384615385,-0.169230769230769,
-0.153846153846154,-0.138461538461538,-0.123076923076923,-0.107692307692308,
-0.0923076923076923,-0.0769230769230769,-0.0615384615384615,-0.0461538461538462,
-0.0307692307692308,-0.0153846153846154,0.),.UNSPECIFIED.)
CURVE()
GEOMETRIC_REPRESENTATION_ITEM()
RATIONAL_B_SPLINE_CURVE((1.,1.,1.,1.,1.,1.,1.,1.,1.,1.,1.,1.,1.,1.,1.,1.,
1.,1.,1.,1.,1.,1.,1.,1.,1.,1.,1.,1.,1.,1.,1.,1.,1.,1.,1.,1.,1.,1.,1.,1.,
1.,1.,1.,1.,1.,1.,1.,1.,1.,1.,1.,1.,1.,1.,1.,1.,1.,1.,1.,1.,1.,1.,1.,1.,
1.,1.,1.,1.,1.,1.))
REPRESENTATION_ITEM('')
);
#210=(
BOUNDED_CURVE()
B_SPLINE_CURVE(5,(#33743,#33744,#33745,#33746,#33747,#33748,#33749,#33750,
#33751,#33752,#33753,#33754,#33755,#33756,#33757,#33758,#33759,#33760,#33761,
#33762,#33763,#33764,#33765,#33766,#33767,#33768,#33769,#33770,#33771,#33772,
#33773,#33774,#33775,#33776,#33777,#33778,#33779,#33780,#33781,#33782,#33783,
#33784,#33785,#33786,#33787,#33788,#33789,#33790,#33791,#33792,#33793,#33794,
#33795,#33796,#33797,#33798,#33799,#33800,#33801,#33802,#33803,#33804,#33805,
#33806,#33807,#33808,#33809,#33810,#33811,#33812),.UNSPECIFIED.,.F.,.F.)
B_SPLINE_CURVE_WITH_KNOTS((6,1,1,1,1,1,1,1,1,1,1,1,1,1,1,1,1,1,1,1,1,1,
1,1,1,1,1,1,1,1,1,1,1,1,1,1,1,1,1,1,1,1,1,1,1,1,1,1,1,1,1,1,1,1,1,1,1,1,
1,1,1,1,1,1,1,6),(-1.,-0.984615384615383,-0.969230769230768,-0.953846153846152,
-0.938461538461537,-0.923076923076922,-0.907692307692306,-0.892307692307691,
-0.876923076923076,-0.86153846153846,-0.846153846153845,-0.83076923076923,
-0.815384615384614,-0.799999999999999,-0.784615384615384,-0.769230769230768,
-0.753846153846153,-0.738461538461538,-0.723076923076922,-0.707692307692307,
-0.692307692307692,-0.676923076923076,-0.661538461538461,-0.646153846153846,
-0.63076923076923,-0.615384615384615,-0.6,-0.584615384615384,-0.569230769230769,
-0.553846153846154,-0.538461538461538,-0.523076923076923,-0.507692307692308,
-0.492307692307692,-0.476923076923077,-0.461538461538462,-0.446153846153846,
-0.430769230769231,-0.415384615384615,-0.4,-0.384615384615385,-0.369230769230769,
-0.353846153846154,-0.338461538461538,-0.323076923076923,-0.307692307692308,
-0.292307692307692,-0.276923076923077,-0.261538461538462,-0.246153846153846,
-0.230769230769231,-0.215384615384615,-0.2,-0.184615384615385,-0.169230769230769,
-0.153846153846154,-0.138461538461538,-0.123076923076923,-0.107692307692308,
-0.0923076923076923,-0.0769230769230769,-0.0615384615384615,-0.0461538461538462,
-0.0307692307692308,-0.0153846153846154,0.),.UNSPECIFIED.)
CURVE()
GEOMETRIC_REPRESENTATION_ITEM()
RATIONAL_B_SPLINE_CURVE((1.,1.,1.,1.,1.,1.,1.,1.,1.,1.,1.,1.,1.,1.,1.,1.,
1.,1.,1.,1.,1.,1.,1.,1.,1.,1.,1.,1.,1.,1.,1.,1.,1.,1.,1.,1.,1.,1.,1.,1.,
1.,1.,1.,1.,1.,1.,1.,1.,1.,1.,1.,1.,1.,1.,1.,1.,1.,1.,1.,1.,1.,1.,1.,1.,
1.,1.,1.,1.,1.,1.))
REPRESENTATION_ITEM('')
);
#956=SHAPE_REPRESENTATION_RELATIONSHIP('SRR','None',#58156,#1006);
#1006=ADVANCED_BREP_SHAPE_REPRESENTATION('',(#1134),#57889);
#1071=STYLED_ITEM('',(#58479),#1134);
#1134=MANIFOLD_SOLID_BREP('Body1',#13633);
#1308=FACE_BOUND('',#3073,.T.);
#1309=FACE_BOUND('',#3077,.T.);
#1310=FACE_BOUND('',#3158,.T.);
#1578=PLANE('',#15129);
#1579=PLANE('',#15130);
#1580=PLANE('',#15131);
#1581=PLANE('',#15132);
#1582=PLANE('',#15159);
#1583=PLANE('',#15160);
#1584=PLANE('',#15163);
#1585=PLANE('',#15166);
#1586=PLANE('',#15169);
#1587=PLANE('',#15172);
#1588=PLANE('',#15175);
#1589=PLANE('',#15178);
#1590=PLANE('',#15181);
#1591=PLANE('',#15184);
#1592=PLANE('',#15187);
#1593=PLANE('',#15190);
#1594=PLANE('',#15193);
#1595=PLANE('',#15196);
#1596=PLANE('',#15199);
#1597=PLANE('',#15202);
#1598=PLANE('',#15205);
#1599=PLANE('',#15208);
#1600=PLANE('',#15211);
#1601=PLANE('',#15214);
#1602=PLANE('',#15217);
#1603=PLANE('',#15218);
#2139=FACE_OUTER_BOUND('',#3069,.T.);
#2140=FACE_OUTER_BOUND('',#3070,.T.);
#2141=FACE_OUTER_BOUND('',#3071,.T.);
#2142=FACE_OUTER_BOUND('',#3072,.T.);
#2143=FACE_OUTER_BOUND('',#3074,.T.);
#2144=FACE_OUTER_BOUND('',#3075,.T.);
#2145=FACE_OUTER_BOUND('',#3076,.T.);
#2146=FACE_OUTER_BOUND('',#3078,.T.);
#2147=FACE_OUTER_BOUND('',#3079,.T.);
#2148=FACE_OUTER_BOUND('',#3080,.T.);
#2149=FACE_OUTER_BOUND('',#3081,.T.);
#2150=FACE_OUTER_BOUND('',#3082,.T.);
#2151=FACE_OUTER_BOUND('',#3083,.T.);
#2152=FACE_OUTER_BOUND('',#3084,.T.);
#2153=FACE_OUTER_BOUND('',#3085,.T.);
#2154=FACE_OUTER_BOUND('',#3086,.T.);
#2155=FACE_OUTER_BOUND('',#3087,.T.);
#2156=FACE_OUTER_BOUND('',#3088,.T.);
#2157=FACE_OUTER_BOUND('',#3089,.T.);
#2158=FACE_OUTER_BOUND('',#3090,.T.);
#2159=FACE_OUTER_BOUND('',#3091,.T.);
#2160=FACE_OUTER_BOUND('',#3092,.T.);
#2161=FACE_OUTER_BOUND('',#3093,.T.);
#2162=FACE_OUTER_BOUND('',#3094,.T.);
#2163=FACE_OUTER_BOUND('',#3095,.T.);
#2164=FACE_OUTER_BOUND('',#3096,.T.);
#2165=FACE_OUTER_BOUND('',#3097,.T.);
#2166=FACE_OUTER_BOUND('',#3098,.T.);
#2167=FACE_OUTER_BOUND('',#3099,.T.);
#2168=FACE_OUTER_BOUND('',#3100,.T.);
#2169=FACE_OUTER_BOUND('',#3101,.T.);
#2170=FACE_OUTER_BOUND('',#3102,.T.);
#2171=FACE_OUTER_BOUND('',#3103,.T.);
#2172=FACE_OUTER_BOUND('',#3104,.T.);
#2173=FACE_OUTER_BOUND('',#3105,.T.);
#2174=FACE_OUTER_BOUND('',#3106,.T.);
#2175=FACE_OUTER_BOUND('',#3107,.T.);
#2176=FACE_OUTER_BOUND('',#3108,.T.);
#2177=FACE_OUTER_BOUND('',#3109,.T.);
#2178=FACE_OUTER_BOUND('',#3110,.T.);
#2179=FACE_OUTER_BOUND('',#3111,.T.);
#2180=FACE_OUTER_BOUND('',#3112,.T.);
#2181=FACE_OUTER_BOUND('',#3113,.T.);
#2182=FACE_OUTER_BOUND('',#3114,.T.);
#2183=FACE_OUTER_BOUND('',#3115,.T.);
#2184=FACE_OUTER_BOUND('',#3116,.T.);
#2185=FACE_OUTER_BOUND('',#3117,.T.);
#2186=FACE_OUTER_BOUND('',#3118,.T.);
#2187=FACE_OUTER_BOUND('',#3119,.T.);
#2188=FACE_OUTER_BOUND('',#3120,.T.);
#2189=FACE_OUTER_BOUND('',#3121,.T.);
#2190=FACE_OUTER_BOUND('',#3122,.T.);
#2191=FACE_OUTER_BOUND('',#3123,.T.);
#2192=FACE_OUTER_BOUND('',#3124,.T.);
#2193=FACE_OUTER_BOUND('',#3125,.T.);
#2194=FACE_OUTER_BOUND('',#3126,.T.);
#2195=FACE_OUTER_BOUND('',#3127,.T.);
#2196=FACE_OUTER_BOUND('',#3128,.T.);
#2197=FACE_OUTER_BOUND('',#3129,.T.);
#2198=FACE_OUTER_BOUND('',#3130,.T.);
#2199=FACE_OUTER_BOUND('',#3131,.T.);
#2200=FACE_OUTER_BOUND('',#3132,.T.);
#2201=FACE_OUTER_BOUND('',#3133,.T.);
#2202=FACE_OUTER_BOUND('',#3134,.T.);
#2203=FACE_OUTER_BOUND('',#3135,.T.);
#2204=FACE_OUTER_BOUND('',#3136,.T.);
#2205=FACE_OUTER_BOUND('',#3137,.T.);
#2206=FACE_OUTER_BOUND('',#3138,.T.);
#2207=FACE_OUTER_BOUND('',#3139,.T.);
#2208=FACE_OUTER_BOUND('',#3140,.T.);
#2209=FACE_OUTER_BOUND('',#3141,.T.);
#2210=FACE_OUTER_BOUND('',#3142,.T.);
#2211=FACE_OUTER_BOUND('',#3143,.T.);
#2212=FACE_OUTER_BOUND('',#3144,.T.);
#2213=FACE_OUTER_BOUND('',#3145,.T.);
#2214=FACE_OUTER_BOUND('',#3146,.T.);
#2215=FACE_OUTER_BOUND('',#3147,.T.);
#2216=FACE_OUTER_BOUND('',#3148,.T.);
#2217=FACE_OUTER_BOUND('',#3149,.T.);
#2218=FACE_OUTER_BOUND('',#3150,.T.);
#2219=FACE_OUTER_BOUND('',#3151,.T.);
#2220=FACE_OUTER_BOUND('',#3152,.T.);
#2221=FACE_OUTER_BOUND('',#3153,.T.);
#2222=FACE_OUTER_BOUND('',#3154,.T.);
#2223=FACE_OUTER_BOUND('',#3155,.T.);
#2224=FACE_OUTER_BOUND('',#3156,.T.);
#2225=FACE_OUTER_BOUND('',#3157,.T.);
#2226=FACE_OUTER_BOUND('',#3159,.T.);
#3069=EDGE_LOOP('',(#10849,#10850,#10851,#10852));
#3070=EDGE_LOOP('',(#10853,#10854,#10855,#10856));
#3071=EDGE_LOOP('',(#10857,#10858,#10859,#10860));
#3072=EDGE_LOOP('',(#10861,#10862,#10863,#10864,#10865,#10866,#10867,#10868,
#10869,#10870,#10871,#10872,#10873,#10874,#10875,#10876,#10877,#10878,#10879,
#10880,#10881,#10882,#10883,#10884,#10885,#10886,#10887,#10888,#10889,#10890,
#10891,#10892,#10893,#10894,#10895,#10896,#10897,#10898,#10899,#10900,#10901,
#10902,#10903,#10904,#10905,#10906,#10907,#10908,#10909,#10910,#10911,#10912,
#10913,#10914,#10915,#10916,#10917,#10918,#10919,#10920,#10921,#10922,#10923,
#10924,#10925,#10926,#10927,#10928,#10929,#10930,#10931,#10932,#10933,#10934,
#10935,#10936,#10937,#10938,#10939,#10940));
#3073=EDGE_LOOP('',(#10941,#10942,#10943,#10944));
#3074=EDGE_LOOP('',(#10945,#10946,#10947,#10948));
#3075=EDGE_LOOP('',(#10949,#10950,#10951,#10952));
#3076=EDGE_LOOP('',(#10953));
#3077=EDGE_LOOP('',(#10954,#10955,#10956,#10957));
#3078=EDGE_LOOP('',(#10958,#10959,#10960,#10961));
#3079=EDGE_LOOP('',(#10962,#10963,#10964,#10965));
#3080=EDGE_LOOP('',(#10966,#10967,#10968,#10969));
#3081=EDGE_LOOP('',(#10970,#10971,#10972,#10973));
#3082=EDGE_LOOP('',(#10974,#10975,#10976,#10977));
#3083=EDGE_LOOP('',(#10978,#10979,#10980,#10981));
#3084=EDGE_LOOP('',(#10982,#10983,#10984,#10985));
#3085=EDGE_LOOP('',(#10986,#10987,#10988,#10989));
#3086=EDGE_LOOP('',(#10990,#10991,#10992,#10993));
#3087=EDGE_LOOP('',(#10994,#10995,#10996,#10997));
#3088=EDGE_LOOP('',(#10998,#10999,#11000,#11001));
#3089=EDGE_LOOP('',(#11002,#11003,#11004,#11005));
#3090=EDGE_LOOP('',(#11006,#11007,#11008,#11009));
#3091=EDGE_LOOP('',(#11010,#11011,#11012,#11013));
#3092=EDGE_LOOP('',(#11014,#11015,#11016,#11017));
#3093=EDGE_LOOP('',(#11018,#11019,#11020,#11021));
#3094=EDGE_LOOP('',(#11022,#11023,#11024,#11025));
#3095=EDGE_LOOP('',(#11026,#11027,#11028,#11029));
#3096=EDGE_LOOP('',(#11030,#11031,#11032,#11033));
#3097=EDGE_LOOP('',(#11034,#11035,#11036,#11037));
#3098=EDGE_LOOP('',(#11038,#11039,#11040,#11041));
#3099=EDGE_LOOP('',(#11042,#11043,#11044,#11045));
#3100=EDGE_LOOP('',(#11046,#11047,#11048,#11049));
#3101=EDGE_LOOP('',(#11050,#11051,#11052,#11053));
#3102=EDGE_LOOP('',(#11054,#11055,#11056,#11057));
#3103=EDGE_LOOP('',(#11058,#11059,#11060,#11061));
#3104=EDGE_LOOP('',(#11062,#11063,#11064,#11065));
#3105=EDGE_LOOP('',(#11066,#11067,#11068,#11069));
#3106=EDGE_LOOP('',(#11070,#11071,#11072,#11073));
#3107=EDGE_LOOP('',(#11074,#11075,#11076,#11077));
#3108=EDGE_LOOP('',(#11078,#11079,#11080,#11081));
#3109=EDGE_LOOP('',(#11082,#11083,#11084,#11085));
#3110=EDGE_LOOP('',(#11086,#11087,#11088,#11089));
#3111=EDGE_LOOP('',(#11090,#11091,#11092,#11093));
#3112=EDGE_LOOP('',(#11094,#11095,#11096,#11097));
#3113=EDGE_LOOP('',(#11098,#11099,#11100,#11101));
#3114=EDGE_LOOP('',(#11102,#11103,#11104,#11105));
#3115=EDGE_LOOP('',(#11106,#11107,#11108,#11109));
#3116=EDGE_LOOP('',(#11110,#11111,#11112,#11113));
#3117=EDGE_LOOP('',(#11114,#11115,#11116,#11117));
#3118=EDGE_LOOP('',(#11118,#11119,#11120,#11121));
#3119=EDGE_LOOP('',(#11122,#11123,#11124,#11125));
#3120=EDGE_LOOP('',(#11126,#11127,#11128,#11129));
#3121=EDGE_LOOP('',(#11130,#11131,#11132,#11133));
#3122=EDGE_LOOP('',(#11134,#11135,#11136,#11137));
#3123=EDGE_LOOP('',(#11138,#11139,#11140,#11141));
#3124=EDGE_LOOP('',(#11142,#11143,#11144,#11145));
#3125=EDGE_LOOP('',(#11146,#11147,#11148,#11149));
#3126=EDGE_LOOP('',(#11150,#11151,#11152,#11153));
#3127=EDGE_LOOP('',(#11154,#11155,#11156,#11157));
#3128=EDGE_LOOP('',(#11158,#11159,#11160,#11161));
#3129=EDGE_LOOP('',(#11162,#11163,#11164,#11165));
#3130=EDGE_LOOP('',(#11166,#11167,#11168,#11169));
#3131=EDGE_LOOP('',(#11170,#11171,#11172,#11173));
#3132=EDGE_LOOP('',(#11174,#11175,#11176,#11177));
#3133=EDGE_LOOP('',(#11178,#11179,#11180,#11181));
#3134=EDGE_LOOP('',(#11182,#11183,#11184,#11185));
#3135=EDGE_LOOP('',(#11186,#11187,#11188,#11189));
#3136=EDGE_LOOP('',(#11190,#11191,#11192,#11193));
#3137=EDGE_LOOP('',(#11194,#11195,#11196,#11197));
#3138=EDGE_LOOP('',(#11198,#11199,#11200,#11201));
#3139=EDGE_LOOP('',(#11202,#11203,#11204,#11205));
#3140=EDGE_LOOP('',(#11206,#11207,#11208,#11209));
#3141=EDGE_LOOP('',(#11210,#11211,#11212,#11213));
#3142=EDGE_LOOP('',(#11214,#11215,#11216,#11217));
#3143=EDGE_LOOP('',(#11218,#11219,#11220,#11221));
#3144=EDGE_LOOP('',(#11222,#11223,#11224,#11225));
#3145=EDGE_LOOP('',(#11226,#11227,#11228,#11229));
#3146=EDGE_LOOP('',(#11230,#11231,#11232,#11233));
#3147=EDGE_LOOP('',(#11234,#11235,#11236,#11237));
#3148=EDGE_LOOP('',(#11238,#11239,#11240,#11241));
#3149=EDGE_LOOP('',(#11242,#11243,#11244,#11245));
#3150=EDGE_LOOP('',(#11246,#11247,#11248,#11249));
#3151=EDGE_LOOP('',(#11250,#11251,#11252,#11253));
#3152=EDGE_LOOP('',(#11254,#11255,#11256,#11257));
#3153=EDGE_LOOP('',(#11258,#11259,#11260,#11261));
#3154=EDGE_LOOP('',(#11262,#11263,#11264,#11265));
#3155=EDGE_LOOP('',(#11266,#11267,#11268,#11269));
#3156=EDGE_LOOP('',(#11270,#11271,#11272,#11273));
#3157=EDGE_LOOP('',(#11274,#11275,#11276,#11277,#11278,#11279,#11280,#11281,
#11282,#11283,#11284,#11285,#11286,#11287,#11288,#11289,#11290,#11291,#11292,
#11293,#11294,#11295,#11296,#11297,#11298,#11299,#11300,#11301,#11302,#11303,
#11304,#11305,#11306,#11307,#11308,#11309,#11310,#11311,#11312,#11313,#11314,
#11315,#11316,#11317,#11318,#11319,#11320,#11321,#11322,#11323,#11324,#11325,
#11326,#11327,#11328,#11329,#11330,#11331,#11332,#11333,#11334,#11335,#11336,
#11337,#11338,#11339,#11340,#11341,#11342,#11343,#11344,#11345,#11346,#11347,
#11348,#11349,#11350,#11351,#11352,#11353));
#3158=EDGE_LOOP('',(#11354));
#3159=EDGE_LOOP('',(#11355,#11356,#11357,#11358));
#3920=LINE('',#22227,#4809);
#3921=LINE('',#22229,#4810);
#3922=LINE('',#22231,#4811);
#3923=LINE('',#22232,#4812);
#3924=LINE('',#22235,#4813);
#3925=LINE('',#22237,#4814);
#3926=LINE('',#22238,#4815);
#3927=LINE('',#22241,#4816);
#3928=LINE('',#22243,#4817);
#3929=LINE('',#22244,#4818);
#3930=LINE('',#22321,#4819);
#3931=LINE('',#22467,#4820);
#3932=LINE('',#22613,#4821);
#3933=LINE('',#22759,#4822);
#3934=LINE('',#22905,#4823);
#3935=LINE('',#23051,#4824);
#3936=LINE('',#23197,#4825);
#3937=LINE('',#23343,#4826);
#3938=LINE('',#23489,#4827);
#3939=LINE('',#23635,#4828);
#3940=LINE('',#23781,#4829);
#3941=LINE('',#23927,#4830);
#3942=LINE('',#24073,#4831);
#3943=LINE('',#24219,#4832);
#3944=LINE('',#24365,#4833);
#3945=LINE('',#24511,#4834);
#3946=LINE('',#24657,#4835);
#3947=LINE('',#24803,#4836);
#3948=LINE('',#24949,#4837);
#3949=LINE('',#25095,#4838);
#3950=LINE('',#25173,#4839);
#3951=LINE('',#25317,#4840);
#3952=LINE('',#25389,#4841);
#3953=LINE('',#25392,#4842);
#3954=LINE('',#25393,#4843);
#3955=LINE('',#25605,#4844);
#3956=LINE('',#25609,#4845);
#3957=LINE('',#25821,#4846);
#3958=LINE('',#25824,#4847);
#3959=LINE('',#25825,#4848);
#3960=LINE('',#26037,#4849);
#3961=LINE('',#26041,#4850);
#3962=LINE('',#26253,#4851);
#3963=LINE('',#26256,#4852);
#3964=LINE('',#26257,#4853);
#3965=LINE('',#26469,#4854);
#3966=LINE('',#26473,#4855);
#3967=LINE('',#26685,#4856);
#3968=LINE('',#26688,#4857);
#3969=LINE('',#26689,#4858);
#3970=LINE('',#26901,#4859);
#3971=LINE('',#26905,#4860);
#3972=LINE('',#27117,#4861);
#3973=LINE('',#27120,#4862);
#3974=LINE('',#27121,#4863);
#3975=LINE('',#27333,#4864);
#3976=LINE('',#27337,#4865);
#3977=LINE('',#27549,#4866);
#3978=LINE('',#27552,#4867);
#3979=LINE('',#27553,#4868);
#3980=LINE('',#27765,#4869);
#3981=LINE('',#27769,#4870);
#3982=LINE('',#27981,#4871);
#3983=LINE('',#27984,#4872);
#3984=LINE('',#27985,#4873);
#3985=LINE('',#28197,#4874);
#3986=LINE('',#28201,#4875);
#3987=LINE('',#28413,#4876);
#3988=LINE('',#28416,#4877);
#3989=LINE('',#28417,#4878);
#3990=LINE('',#28629,#4879);
#3991=LINE('',#28633,#4880);
#3992=LINE('',#28845,#4881);
#3993=LINE('',#28848,#4882);
#3994=LINE('',#28849,#4883);
#3995=LINE('',#29061,#4884);
#3996=LINE('',#29065,#4885);
#3997=LINE('',#29277,#4886);
#3998=LINE('',#29280,#4887);
#3999=LINE('',#29281,#4888);
#4000=LINE('',#29493,#4889);
#4001=LINE('',#29497,#4890);
#4002=LINE('',#29709,#4891);
#4003=LINE('',#29712,#4892);
#4004=LINE('',#29713,#4893);
#4005=LINE('',#29925,#4894);
#4006=LINE('',#29929,#4895);
#4007=LINE('',#30141,#4896);
#4008=LINE('',#30144,#4897);
#4009=LINE('',#30145,#4898);
#4010=LINE('',#30357,#4899);
#4011=LINE('',#30361,#4900);
#4012=LINE('',#30573,#4901);
#4013=LINE('',#30576,#4902);
#4014=LINE('',#30577,#4903);
#4015=LINE('',#30789,#4904);
#4016=LINE('',#30793,#4905);
#4017=LINE('',#31005,#4906);
#4018=LINE('',#31008,#4907);
#4019=LINE('',#31009,#4908);
#4020=LINE('',#31221,#4909);
#4021=LINE('',#31225,#4910);
#4022=LINE('',#31437,#4911);
#4023=LINE('',#31440,#4912);
#4024=LINE('',#31441,#4913);
#4025=LINE('',#31653,#4914);
#4026=LINE('',#31657,#4915);
#4027=LINE('',#31869,#4916);
#4028=LINE('',#31872,#4917);
#4029=LINE('',#31873,#4918);
#4030=LINE('',#32085,#4919);
#4031=LINE('',#32089,#4920);
#4032=LINE('',#32301,#4921);
#4033=LINE('',#32304,#4922);
#4034=LINE('',#32305,#4923);
#4035=LINE('',#32517,#4924);
#4036=LINE('',#32521,#4925);
#4037=LINE('',#32733,#4926);
#4038=LINE('',#32736,#4927);
#4039=LINE('',#32737,#4928);
#4040=LINE('',#32949,#4929);
#4041=LINE('',#32953,#4930);
#4042=LINE('',#33165,#4931);
#4043=LINE('',#33168,#4932);
#4044=LINE('',#33169,#4933);
#4045=LINE('',#33381,#4934);
#4046=LINE('',#33385,#4935);
#4047=LINE('',#33597,#4936);
#4048=LINE('',#33600,#4937);
#4049=LINE('',#33601,#4938);
#4050=LINE('',#33813,#4939);
#4809=VECTOR('',#17957,1.);
#4810=VECTOR('',#17958,1.);
#4811=VECTOR('',#17959,1.);
#4812=VECTOR('',#17960,1.);
#4813=VECTOR('',#17963,1.);
#4814=VECTOR('',#17964,1.);
#4815=VECTOR('',#17965,1.);
#4816=VECTOR('',#17968,1.);
#4817=VECTOR('',#17969,1.);
#4818=VECTOR('',#17970,1.);
#4819=VECTOR('',#17975,1.);
#4820=VECTOR('',#17978,1.);
#4821=VECTOR('',#17981,1.);
#4822=VECTOR('',#17984,1.);
#4823=VECTOR('',#17987,1.);
#4824=VECTOR('',#17990,1.);
#4825=VECTOR('',#17993,1.);
#4826=VECTOR('',#17996,1.);
#4827=VECTOR('',#17999,1.);
#4828=VECTOR('',#18002,1.);
#4829=VECTOR('',#18005,1.);
#4830=VECTOR('',#18008,1.);
#4831=VECTOR('',#18011,1.);
#4832=VECTOR('',#18014,1.);
#4833=VECTOR('',#18017,1.);
#4834=VECTOR('',#18020,1.);
#4835=VECTOR('',#18023,1.);
#4836=VECTOR('',#18026,1.);
#4837=VECTOR('',#18029,1.);
#4838=VECTOR('',#18032,1.);
#4839=VECTOR('',#18043,1.4);
#4840=VECTOR('',#18048,1.);
#4841=VECTOR('',#18049,1.);
#4842=VECTOR('',#18052,1.);
#4843=VECTOR('',#18053,1.);
#4844=VECTOR('',#18054,1.);
#4845=VECTOR('',#18059,1.);
#4846=VECTOR('',#18060,1.);
#4847=VECTOR('',#18063,1.);
#4848=VECTOR('',#18064,1.);
#4849=VECTOR('',#18065,1.);
#4850=VECTOR('',#18070,1.);
#4851=VECTOR('',#18071,1.);
#4852=VECTOR('',#18074,1.);
#4853=VECTOR('',#18075,1.);
#4854=VECTOR('',#18076,1.);
#4855=VECTOR('',#18081,1.);
#4856=VECTOR('',#18082,1.);
#4857=VECTOR('',#18085,1.);
#4858=VECTOR('',#18086,1.);
#4859=VECTOR('',#18087,1.);
#4860=VECTOR('',#18092,1.);
#4861=VECTOR('',#18093,1.);
#4862=VECTOR('',#18096,1.);
#4863=VECTOR('',#18097,1.);
#4864=VECTOR('',#18098,1.);
#4865=VECTOR('',#18103,1.);
#4866=VECTOR('',#18104,1.);
#4867=VECTOR('',#18107,1.);
#4868=VECTOR('',#18108,1.);
#4869=VECTOR('',#18109,1.);
#4870=VECTOR('',#18114,1.);
#4871=VECTOR('',#18115,1.);
#4872=VECTOR('',#18118,1.);
#4873=VECTOR('',#18119,1.);
#4874=VECTOR('',#18120,1.);
#4875=VECTOR('',#18125,1.);
#4876=VECTOR('',#18126,1.);
#4877=VECTOR('',#18129,1.);
#4878=VECTOR('',#18130,1.);
#4879=VECTOR('',#18131,1.);
#4880=VECTOR('',#18136,1.);
#4881=VECTOR('',#18137,1.);
#4882=VECTOR('',#18140,1.);
#4883=VECTOR('',#18141,1.);
#4884=VECTOR('',#18142,1.);
#4885=VECTOR('',#18147,1.);
#4886=VECTOR('',#18148,1.);
#4887=VECTOR('',#18151,1.);
#4888=VECTOR('',#18152,1.);
#4889=VECTOR('',#18153,1.);
#4890=VECTOR('',#18158,1.);
#4891=VECTOR('',#18159,1.);
#4892=VECTOR('',#18162,1.);
#4893=VECTOR('',#18163,1.);
#4894=VECTOR('',#18164,1.);
#4895=VECTOR('',#18169,1.);
#4896=VECTOR('',#18170,1.);
#4897=VECTOR('',#18173,1.);
#4898=VECTOR('',#18174,1.);
#4899=VECTOR('',#18175,1.);
#4900=VECTOR('',#18180,1.);
#4901=VECTOR('',#18181,1.);
#4902=VECTOR('',#18184,1.);
#4903=VECTOR('',#18185,1.);
#4904=VECTOR('',#18186,1.);
#4905=VECTOR('',#18191,1.);
#4906=VECTOR('',#18192,1.);
#4907=VECTOR('',#18195,1.);
#4908=VECTOR('',#18196,1.);
#4909=VECTOR('',#18197,1.);
#4910=VECTOR('',#18202,1.);
#4911=VECTOR('',#18203,1.);
#4912=VECTOR('',#18206,1.);
#4913=VECTOR('',#18207,1.);
#4914=VECTOR('',#18208,1.);
#4915=VECTOR('',#18213,1.);
#4916=VECTOR('',#18214,1.);
#4917=VECTOR('',#18217,1.);
#4918=VECTOR('',#18218,1.);
#4919=VECTOR('',#18219,1.);
#4920=VECTOR('',#18224,1.);
#4921=VECTOR('',#18225,1.);
#4922=VECTOR('',#18228,1.);
#4923=VECTOR('',#18229,1.);
#4924=VECTOR('',#18230,1.);
#4925=VECTOR('',#18235,1.);
#4926=VECTOR('',#18236,1.);
#4927=VECTOR('',#18239,1.);
#4928=VECTOR('',#18240,1.);
#4929=VECTOR('',#18241,1.);
#4930=VECTOR('',#18246,1.);
#4931=VECTOR('',#18247,1.);
#4932=VECTOR('',#18250,1.);
#4933=VECTOR('',#18251,1.);
#4934=VECTOR('',#18252,1.);
#4935=VECTOR('',#18257,1.);
#4936=VECTOR('',#18258,1.);
#4937=VECTOR('',#18261,1.);
#4938=VECTOR('',#18262,1.);
#4939=VECTOR('',#18263,1.);
#5617=CIRCLE('',#15133,1.75);
#5618=CIRCLE('',#15134,1.75);
#5619=CIRCLE('',#15135,1.75);
#5620=CIRCLE('',#15136,1.75);
#5621=CIRCLE('',#15137,1.75);
#5622=CIRCLE('',#15138,1.75);
#5623=CIRCLE('',#15139,1.75);
#5624=CIRCLE('',#15140,1.75);
#5625=CIRCLE('',#15141,1.75);
#5626=CIRCLE('',#15142,1.75);
#5627=CIRCLE('',#15143,1.75);
#5628=CIRCLE('',#15144,1.75);
#5629=CIRCLE('',#15145,1.75);
#5630=CIRCLE('',#15146,1.75);
#5631=CIRCLE('',#15147,1.75);
#5632=CIRCLE('',#15148,1.75);
#5633=CIRCLE('',#15149,1.75);
#5634=CIRCLE('',#15150,1.75);
#5635=CIRCLE('',#15151,1.75);
#5636=CIRCLE('',#15152,1.75);
#5637=CIRCLE('',#15153,0.6);
#5638=CIRCLE('',#15155,0.6);
#5639=CIRCLE('',#15157,1.4);
#5640=CIRCLE('',#15158,1.4);
#5641=CIRCLE('',#15162,1.75);
#5642=CIRCLE('',#15165,1.75);
#5643=CIRCLE('',#15168,1.75);
#5644=CIRCLE('',#15171,1.75);
#5645=CIRCLE('',#15174,1.75);
#5646=CIRCLE('',#15177,1.75);
#5647=CIRCLE('',#15180,1.75);
#5648=CIRCLE('',#15183,1.75);
#5649=CIRCLE('',#15186,1.75);
#5650=CIRCLE('',#15189,1.75);
#5651=CIRCLE('',#15192,1.75);
#5652=CIRCLE('',#15195,1.75);
#5653=CIRCLE('',#15198,1.75);
#5654=CIRCLE('',#15201,1.75);
#5655=CIRCLE('',#15204,1.75);
#5656=CIRCLE('',#15207,1.75);
#5657=CIRCLE('',#15210,1.75);
#5658=CIRCLE('',#15213,1.75);
#5659=CIRCLE('',#15216,1.75);
#5660=CIRCLE('',#15219,1.75);
#6448=VERTEX_POINT('',#22225);
#6449=VERTEX_POINT('',#22226);
#6450=VERTEX_POINT('',#22228);
#6451=VERTEX_POINT('',#22230);
#6452=VERTEX_POINT('',#22234);
#6453=VERTEX_POINT('',#22236);
#6454=VERTEX_POINT('',#22240);
#6455=VERTEX_POINT('',#22242);
#6456=VERTEX_POINT('',#22246);
#6457=VERTEX_POINT('',#22247);
#6458=VERTEX_POINT('',#22249);
#6459=VERTEX_POINT('',#22320);
#6460=VERTEX_POINT('',#22322);
#6461=VERTEX_POINT('',#22393);
#6462=VERTEX_POINT('',#22395);
#6463=VERTEX_POINT('',#22466);
#6464=VERTEX_POINT('',#22468);
#6465=VERTEX_POINT('',#22539);
#6466=VERTEX_POINT('',#22541);
#6467=VERTEX_POINT('',#22612);
#6468=VERTEX_POINT('',#22614);
#6469=VERTEX_POINT('',#22685);
#6470=VERTEX_POINT('',#22687);
#6471=VERTEX_POINT('',#22758);
#6472=VERTEX_POINT('',#22760);
#6473=VERTEX_POINT('',#22831);
#6474=VERTEX_POINT('',#22833);
#6475=VERTEX_POINT('',#22904);
#6476=VERTEX_POINT('',#22906);
#6477=VERTEX_POINT('',#22977);
#6478=VERTEX_POINT('',#22979);
#6479=VERTEX_POINT('',#23050);
#6480=VERTEX_POINT('',#23052);
#6481=VERTEX_POINT('',#23123);
#6482=VERTEX_POINT('',#23125);
#6483=VERTEX_POINT('',#23196);
#6484=VERTEX_POINT('',#23198);
#6485=VERTEX_POINT('',#23269);
#6486=VERTEX_POINT('',#23271);
#6487=VERTEX_POINT('',#23342);
#6488=VERTEX_POINT('',#23344);
#6489=VERTEX_POINT('',#23415);
#6490=VERTEX_POINT('',#23417);
#6491=VERTEX_POINT('',#23488);
#6492=VERTEX_POINT('',#23490);
#6493=VERTEX_POINT('',#23561);
#6494=VERTEX_POINT('',#23563);
#6495=VERTEX_POINT('',#23634);
#6496=VERTEX_POINT('',#23636);
#6497=VERTEX_POINT('',#23707);
#6498=VERTEX_POINT('',#23709);
#6499=VERTEX_POINT('',#23780);
#6500=VERTEX_POINT('',#23782);
#6501=VERTEX_POINT('',#23853);
#6502=VERTEX_POINT('',#23855);
#6503=VERTEX_POINT('',#23926);
#6504=VERTEX_POINT('',#23928);
#6505=VERTEX_POINT('',#23999);
#6506=VERTEX_POINT('',#24001);
#6507=VERTEX_POINT('',#24072);
#6508=VERTEX_POINT('',#24074);
#6509=VERTEX_POINT('',#24145);
#6510=VERTEX_POINT('',#24147);
#6511=VERTEX_POINT('',#24218);
#6512=VERTEX_POINT('',#24220);
#6513=VERTEX_POINT('',#24291);
#6514=VERTEX_POINT('',#24293);
#6515=VERTEX_POINT('',#24364);
#6516=VERTEX_POINT('',#24366);
#6517=VERTEX_POINT('',#24437);
#6518=VERTEX_POINT('',#24439);
#6519=VERTEX_POINT('',#24510);
#6520=VERTEX_POINT('',#24512);
#6521=VERTEX_POINT('',#24583);
#6522=VERTEX_POINT('',#24585);
#6523=VERTEX_POINT('',#24656);
#6524=VERTEX_POINT('',#24658);
#6525=VERTEX_POINT('',#24729);
#6526=VERTEX_POINT('',#24731);
#6527=VERTEX_POINT('',#24802);
#6528=VERTEX_POINT('',#24804);
#6529=VERTEX_POINT('',#24875);
#6530=VERTEX_POINT('',#24877);
#6531=VERTEX_POINT('',#24948);
#6532=VERTEX_POINT('',#24950);
#6533=VERTEX_POINT('',#25021);
#6534=VERTEX_POINT('',#25023);
#6535=VERTEX_POINT('',#25094);
#6536=VERTEX_POINT('',#25170);
#6537=VERTEX_POINT('',#25172);
#6538=VERTEX_POINT('',#25316);
#6539=VERTEX_POINT('',#25318);
#6540=VERTEX_POINT('',#25391);
#6541=VERTEX_POINT('',#25534);
#6542=VERTEX_POINT('',#25607);
#6543=VERTEX_POINT('',#25750);
#6544=VERTEX_POINT('',#25823);
#6545=VERTEX_POINT('',#25966);
#6546=VERTEX_POINT('',#26039);
#6547=VERTEX_POINT('',#26182);
#6548=VERTEX_POINT('',#26255);
#6549=VERTEX_POINT('',#26398);
#6550=VERTEX_POINT('',#26471);
#6551=VERTEX_POINT('',#26614);
#6552=VERTEX_POINT('',#26687);
#6553=VERTEX_POINT('',#26830);
#6554=VERTEX_POINT('',#26903);
#6555=VERTEX_POINT('',#27046);
#6556=VERTEX_POINT('',#27119);
#6557=VERTEX_POINT('',#27262);
#6558=VERTEX_POINT('',#27335);
#6559=VERTEX_POINT('',#27478);
#6560=VERTEX_POINT('',#27551);
#6561=VERTEX_POINT('',#27694);
#6562=VERTEX_POINT('',#27767);
#6563=VERTEX_POINT('',#27910);
#6564=VERTEX_POINT('',#27983);
#6565=VERTEX_POINT('',#28126);
#6566=VERTEX_POINT('',#28199);
#6567=VERTEX_POINT('',#28342);
#6568=VERTEX_POINT('',#28415);
#6569=VERTEX_POINT('',#28558);
#6570=VERTEX_POINT('',#28631);
#6571=VERTEX_POINT('',#28774);
#6572=VERTEX_POINT('',#28847);
#6573=VERTEX_POINT('',#28990);
#6574=VERTEX_POINT('',#29063);
#6575=VERTEX_POINT('',#29206);
#6576=VERTEX_POINT('',#29279);
#6577=VERTEX_POINT('',#29422);
#6578=VERTEX_POINT('',#29495);
#6579=VERTEX_POINT('',#29638);
#6580=VERTEX_POINT('',#29711);
#6581=VERTEX_POINT('',#29854);
#6582=VERTEX_POINT('',#29927);
#6583=VERTEX_POINT('',#30070);
#6584=VERTEX_POINT('',#30143);
#6585=VERTEX_POINT('',#30286);
#6586=VERTEX_POINT('',#30359);
#6587=VERTEX_POINT('',#30502);
#6588=VERTEX_POINT('',#30575);
#6589=VERTEX_POINT('',#30718);
#6590=VERTEX_POINT('',#30791);
#6591=VERTEX_POINT('',#30934);
#6592=VERTEX_POINT('',#31007);
#6593=VERTEX_POINT('',#31150);
#6594=VERTEX_POINT('',#31223);
#6595=VERTEX_POINT('',#31366);
#6596=VERTEX_POINT('',#31439);
#6597=VERTEX_POINT('',#31582);
#6598=VERTEX_POINT('',#31655);
#6599=VERTEX_POINT('',#31798);
#6600=VERTEX_POINT('',#31871);
#6601=VERTEX_POINT('',#32014);
#6602=VERTEX_POINT('',#32087);
#6603=VERTEX_POINT('',#32230);
#6604=VERTEX_POINT('',#32303);
#6605=VERTEX_POINT('',#32446);
#6606=VERTEX_POINT('',#32519);
#6607=VERTEX_POINT('',#32662);
#6608=VERTEX_POINT('',#32735);
#6609=VERTEX_POINT('',#32878);
#6610=VERTEX_POINT('',#32951);
#6611=VERTEX_POINT('',#33094);
#6612=VERTEX_POINT('',#33167);
#6613=VERTEX_POINT('',#33310);
#6614=VERTEX_POINT('',#33383);
#6615=VERTEX_POINT('',#33526);
#6616=VERTEX_POINT('',#33599);
#6617=VERTEX_POINT('',#33742);
#8011=EDGE_CURVE('',#6448,#6449,#3920,.T.);
#8012=EDGE_CURVE('',#6450,#6448,#3921,.T.);
#8013=EDGE_CURVE('',#6451,#6450,#3922,.T.);
#8014=EDGE_CURVE('',#6449,#6451,#3923,.T.);
#8015=EDGE_CURVE('',#6452,#6448,#3924,.T.);
#8016=EDGE_CURVE('',#6452,#6453,#3925,.T.);
#8017=EDGE_CURVE('',#6450,#6453,#3926,.T.);
#8018=EDGE_CURVE('',#6454,#6452,#3927,.T.);
#8019=EDGE_CURVE('',#6455,#6454,#3928,.T.);
#8020=EDGE_CURVE('',#6453,#6455,#3929,.T.);
#8021=EDGE_CURVE('',#6456,#6457,#5617,.T.);
#8022=EDGE_CURVE('',#6457,#6458,#131,.T.);
#8023=EDGE_CURVE('',#6458,#6459,#3930,.T.);
#8024=EDGE_CURVE('',#6459,#6460,#132,.T.);
#8025=EDGE_CURVE('',#6460,#6461,#5618,.T.);
#8026=EDGE_CURVE('',#6461,#6462,#133,.T.);
#8027=EDGE_CURVE('',#6462,#6463,#3931,.T.);
#8028=EDGE_CURVE('',#6463,#6464,#134,.T.);
#8029=EDGE_CURVE('',#6464,#6465,#5619,.T.);
#8030=EDGE_CURVE('',#6465,#6466,#135,.T.);
#8031=EDGE_CURVE('',#6466,#6467,#3932,.T.);
#8032=EDGE_CURVE('',#6467,#6468,#136,.T.);
#8033=EDGE_CURVE('',#6468,#6469,#5620,.T.);
#8034=EDGE_CURVE('',#6469,#6470,#137,.T.);
#8035=EDGE_CURVE('',#6470,#6471,#3933,.T.);
#8036=EDGE_CURVE('',#6471,#6472,#138,.T.);
#8037=EDGE_CURVE('',#6472,#6473,#5621,.T.);
#8038=EDGE_CURVE('',#6473,#6474,#139,.T.);
#8039=EDGE_CURVE('',#6474,#6475,#3934,.T.);
#8040=EDGE_CURVE('',#6475,#6476,#140,.T.);
#8041=EDGE_CURVE('',#6476,#6477,#5622,.T.);
#8042=EDGE_CURVE('',#6477,#6478,#141,.T.);
#8043=EDGE_CURVE('',#6478,#6479,#3935,.T.);
#8044=EDGE_CURVE('',#6479,#6480,#142,.T.);
#8045=EDGE_CURVE('',#6480,#6481,#5623,.T.);
#8046=EDGE_CURVE('',#6481,#6482,#143,.T.);
#8047=EDGE_CURVE('',#6482,#6483,#3936,.T.);
#8048=EDGE_CURVE('',#6483,#6484,#144,.T.);
#8049=EDGE_CURVE('',#6484,#6485,#5624,.T.);
#8050=EDGE_CURVE('',#6485,#6486,#145,.T.);
#8051=EDGE_CURVE('',#6486,#6487,#3937,.T.);
#8052=EDGE_CURVE('',#6487,#6488,#146,.T.);
#8053=EDGE_CURVE('',#6488,#6489,#5625,.T.);
#8054=EDGE_CURVE('',#6489,#6490,#147,.T.);
#8055=EDGE_CURVE('',#6490,#6491,#3938,.T.);
#8056=EDGE_CURVE('',#6491,#6492,#148,.T.);
#8057=EDGE_CURVE('',#6492,#6493,#5626,.T.);
#8058=EDGE_CURVE('',#6493,#6494,#149,.T.);
#8059=EDGE_CURVE('',#6494,#6495,#3939,.T.);
#8060=EDGE_CURVE('',#6495,#6496,#150,.T.);
#8061=EDGE_CURVE('',#6496,#6497,#5627,.T.);
#8062=EDGE_CURVE('',#6497,#6498,#151,.T.);
#8063=EDGE_CURVE('',#6498,#6499,#3940,.T.);
#8064=EDGE_CURVE('',#6499,#6500,#152,.T.);
#8065=EDGE_CURVE('',#6500,#6501,#5628,.T.);
#8066=EDGE_CURVE('',#6501,#6502,#153,.T.);
#8067=EDGE_CURVE('',#6502,#6503,#3941,.T.);
#8068=EDGE_CURVE('',#6503,#6504,#154,.T.);
#8069=EDGE_CURVE('',#6504,#6505,#5629,.T.);
#8070=EDGE_CURVE('',#6505,#6506,#155,.T.);
#8071=EDGE_CURVE('',#6506,#6507,#3942,.T.);
#8072=EDGE_CURVE('',#6507,#6508,#156,.T.);
#8073=EDGE_CURVE('',#6508,#6509,#5630,.T.);
#8074=EDGE_CURVE('',#6509,#6510,#157,.T.);
#8075=EDGE_CURVE('',#6510,#6511,#3943,.T.);
#8076=EDGE_CURVE('',#6511,#6512,#158,.T.);
#8077=EDGE_CURVE('',#6512,#6513,#5631,.T.);
#8078=EDGE_CURVE('',#6513,#6514,#159,.T.);
#8079=EDGE_CURVE('',#6514,#6515,#3944,.T.);
#8080=EDGE_CURVE('',#6515,#6516,#160,.T.);
#8081=EDGE_CURVE('',#6516,#6517,#5632,.T.);
#8082=EDGE_CURVE('',#6517,#6518,#161,.T.);
#8083=EDGE_CURVE('',#6518,#6519,#3945,.T.);
#8084=EDGE_CURVE('',#6519,#6520,#162,.T.);
#8085=EDGE_CURVE('',#6520,#6521,#5633,.T.);
#8086=EDGE_CURVE('',#6521,#6522,#163,.T.);
#8087=EDGE_CURVE('',#6522,#6523,#3946,.T.);
#8088=EDGE_CURVE('',#6523,#6524,#164,.T.);
#8089=EDGE_CURVE('',#6524,#6525,#5634,.T.);
#8090=EDGE_CURVE('',#6525,#6526,#165,.T.);
#8091=EDGE_CURVE('',#6526,#6527,#3947,.T.);
#8092=EDGE_CURVE('',#6527,#6528,#166,.T.);
#8093=EDGE_CURVE('',#6528,#6529,#5635,.T.);
#8094=EDGE_CURVE('',#6529,#6530,#167,.T.);
#8095=EDGE_CURVE('',#6530,#6531,#3948,.T.);
#8096=EDGE_CURVE('',#6531,#6532,#168,.T.);
#8097=EDGE_CURVE('',#6532,#6533,#5636,.T.);
#8098=EDGE_CURVE('',#6533,#6534,#169,.T.);
#8099=EDGE_CURVE('',#6534,#6535,#3949,.T.);
#8100=EDGE_CURVE('',#6535,#6456,#170,.T.);
#8101=EDGE_CURVE('',#6455,#6451,#5637,.T.);
#8102=EDGE_CURVE('',#6449,#6454,#5638,.T.);
#8103=EDGE_CURVE('',#6536,#6536,#5639,.T.);
#8104=EDGE_CURVE('',#6536,#6537,#3950,.T.);
#8105=EDGE_CURVE('',#6537,#6537,#5640,.T.);
#8106=EDGE_CURVE('',#6538,#6533,#3951,.T.);
#8107=EDGE_CURVE('',#6539,#6538,#171,.T.);
#8108=EDGE_CURVE('',#6534,#6539,#3952,.T.);
#8109=EDGE_CURVE('',#6540,#6539,#3953,.T.);
#8110=EDGE_CURVE('',#6535,#6540,#3954,.T.);
#8111=EDGE_CURVE('',#6541,#6540,#172,.T.);
#8112=EDGE_CURVE('',#6456,#6541,#3955,.T.);
#8113=EDGE_CURVE('',#6542,#6541,#5641,.T.);
#8114=EDGE_CURVE('',#6542,#6457,#3956,.T.);
#8115=EDGE_CURVE('',#6543,#6542,#173,.T.);
#8116=EDGE_CURVE('',#6458,#6543,#3957,.T.);
#8117=EDGE_CURVE('',#6544,#6543,#3958,.T.);
#8118=EDGE_CURVE('',#6459,#6544,#3959,.T.);
#8119=EDGE_CURVE('',#6545,#6544,#174,.T.);
#8120=EDGE_CURVE('',#6460,#6545,#3960,.T.);
#8121=EDGE_CURVE('',#6546,#6545,#5642,.T.);
#8122=EDGE_CURVE('',#6546,#6461,#3961,.T.);
#8123=EDGE_CURVE('',#6547,#6546,#175,.T.);
#8124=EDGE_CURVE('',#6462,#6547,#3962,.T.);
#8125=EDGE_CURVE('',#6548,#6547,#3963,.T.);
#8126=EDGE_CURVE('',#6463,#6548,#3964,.T.);
#8127=EDGE_CURVE('',#6549,#6548,#176,.T.);
#8128=EDGE_CURVE('',#6464,#6549,#3965,.T.);
#8129=EDGE_CURVE('',#6550,#6549,#5643,.T.);
#8130=EDGE_CURVE('',#6550,#6465,#3966,.T.);
#8131=EDGE_CURVE('',#6551,#6550,#177,.T.);
#8132=EDGE_CURVE('',#6466,#6551,#3967,.T.);
#8133=EDGE_CURVE('',#6552,#6551,#3968,.T.);
#8134=EDGE_CURVE('',#6467,#6552,#3969,.T.);
#8135=EDGE_CURVE('',#6553,#6552,#178,.T.);
#8136=EDGE_CURVE('',#6468,#6553,#3970,.T.);
#8137=EDGE_CURVE('',#6554,#6553,#5644,.T.);
#8138=EDGE_CURVE('',#6554,#6469,#3971,.T.);
#8139=EDGE_CURVE('',#6555,#6554,#179,.T.);
#8140=EDGE_CURVE('',#6470,#6555,#3972,.T.);
#8141=EDGE_CURVE('',#6556,#6555,#3973,.T.);
#8142=EDGE_CURVE('',#6471,#6556,#3974,.T.);
#8143=EDGE_CURVE('',#6557,#6556,#180,.T.);
#8144=EDGE_CURVE('',#6472,#6557,#3975,.T.);
#8145=EDGE_CURVE('',#6558,#6557,#5645,.T.);
#8146=EDGE_CURVE('',#6558,#6473,#3976,.T.);
#8147=EDGE_CURVE('',#6559,#6558,#181,.T.);
#8148=EDGE_CURVE('',#6474,#6559,#3977,.T.);
#8149=EDGE_CURVE('',#6560,#6559,#3978,.T.);
#8150=EDGE_CURVE('',#6475,#6560,#3979,.T.);
#8151=EDGE_CURVE('',#6561,#6560,#182,.T.);
#8152=EDGE_CURVE('',#6476,#6561,#3980,.T.);
#8153=EDGE_CURVE('',#6562,#6561,#5646,.T.);
#8154=EDGE_CURVE('',#6562,#6477,#3981,.T.);
#8155=EDGE_CURVE('',#6563,#6562,#183,.T.);
#8156=EDGE_CURVE('',#6478,#6563,#3982,.T.);
#8157=EDGE_CURVE('',#6564,#6563,#3983,.T.);
#8158=EDGE_CURVE('',#6479,#6564,#3984,.T.);
#8159=EDGE_CURVE('',#6565,#6564,#184,.T.);
#8160=EDGE_CURVE('',#6480,#6565,#3985,.T.);
#8161=EDGE_CURVE('',#6566,#6565,#5647,.T.);
#8162=EDGE_CURVE('',#6566,#6481,#3986,.T.);
#8163=EDGE_CURVE('',#6567,#6566,#185,.T.);
#8164=EDGE_CURVE('',#6482,#6567,#3987,.T.);
#8165=EDGE_CURVE('',#6568,#6567,#3988,.T.);
#8166=EDGE_CURVE('',#6483,#6568,#3989,.T.);
#8167=EDGE_CURVE('',#6569,#6568,#186,.T.);
#8168=EDGE_CURVE('',#6484,#6569,#3990,.T.);
#8169=EDGE_CURVE('',#6570,#6569,#5648,.T.);
#8170=EDGE_CURVE('',#6570,#6485,#3991,.T.);
#8171=EDGE_CURVE('',#6571,#6570,#187,.T.);
#8172=EDGE_CURVE('',#6486,#6571,#3992,.T.);
#8173=EDGE_CURVE('',#6572,#6571,#3993,.T.);
#8174=EDGE_CURVE('',#6487,#6572,#3994,.T.);
#8175=EDGE_CURVE('',#6573,#6572,#188,.T.);
#8176=EDGE_CURVE('',#6488,#6573,#3995,.T.);
#8177=EDGE_CURVE('',#6574,#6573,#5649,.T.);
#8178=EDGE_CURVE('',#6574,#6489,#3996,.T.);
#8179=EDGE_CURVE('',#6575,#6574,#189,.T.);
#8180=EDGE_CURVE('',#6490,#6575,#3997,.T.);
#8181=EDGE_CURVE('',#6576,#6575,#3998,.T.);
#8182=EDGE_CURVE('',#6491,#6576,#3999,.T.);
#8183=EDGE_CURVE('',#6577,#6576,#190,.T.);
#8184=EDGE_CURVE('',#6492,#6577,#4000,.T.);
#8185=EDGE_CURVE('',#6578,#6577,#5650,.T.);
#8186=EDGE_CURVE('',#6578,#6493,#4001,.T.);
#8187=EDGE_CURVE('',#6579,#6578,#191,.T.);
#8188=EDGE_CURVE('',#6494,#6579,#4002,.T.);
#8189=EDGE_CURVE('',#6580,#6579,#4003,.T.);
#8190=EDGE_CURVE('',#6495,#6580,#4004,.T.);
#8191=EDGE_CURVE('',#6581,#6580,#192,.T.);
#8192=EDGE_CURVE('',#6496,#6581,#4005,.T.);
#8193=EDGE_CURVE('',#6582,#6581,#5651,.T.);
#8194=EDGE_CURVE('',#6582,#6497,#4006,.T.);
#8195=EDGE_CURVE('',#6583,#6582,#193,.T.);
#8196=EDGE_CURVE('',#6498,#6583,#4007,.T.);
#8197=EDGE_CURVE('',#6584,#6583,#4008,.T.);
#8198=EDGE_CURVE('',#6499,#6584,#4009,.T.);
#8199=EDGE_CURVE('',#6585,#6584,#194,.T.);
#8200=EDGE_CURVE('',#6500,#6585,#4010,.T.);
#8201=EDGE_CURVE('',#6586,#6585,#5652,.T.);
#8202=EDGE_CURVE('',#6586,#6501,#4011,.T.);
#8203=EDGE_CURVE('',#6587,#6586,#195,.T.);
#8204=EDGE_CURVE('',#6502,#6587,#4012,.T.);
#8205=EDGE_CURVE('',#6588,#6587,#4013,.T.);
#8206=EDGE_CURVE('',#6503,#6588,#4014,.T.);
#8207=EDGE_CURVE('',#6589,#6588,#196,.T.);
#8208=EDGE_CURVE('',#6504,#6589,#4015,.T.);
#8209=EDGE_CURVE('',#6590,#6589,#5653,.T.);
#8210=EDGE_CURVE('',#6590,#6505,#4016,.T.);
#8211=EDGE_CURVE('',#6591,#6590,#197,.T.);
#8212=EDGE_CURVE('',#6506,#6591,#4017,.T.);
#8213=EDGE_CURVE('',#6592,#6591,#4018,.T.);
#8214=EDGE_CURVE('',#6507,#6592,#4019,.T.);
#8215=EDGE_CURVE('',#6593,#6592,#198,.T.);
#8216=EDGE_CURVE('',#6508,#6593,#4020,.T.);
#8217=EDGE_CURVE('',#6594,#6593,#5654,.T.);
#8218=EDGE_CURVE('',#6594,#6509,#4021,.T.);
#8219=EDGE_CURVE('',#6595,#6594,#199,.T.);
#8220=EDGE_CURVE('',#6510,#6595,#4022,.T.);
#8221=EDGE_CURVE('',#6596,#6595,#4023,.T.);
#8222=EDGE_CURVE('',#6511,#6596,#4024,.T.);
#8223=EDGE_CURVE('',#6597,#6596,#200,.T.);
#8224=EDGE_CURVE('',#6512,#6597,#4025,.T.);
#8225=EDGE_CURVE('',#6598,#6597,#5655,.T.);
#8226=EDGE_CURVE('',#6598,#6513,#4026,.T.);
#8227=EDGE_CURVE('',#6599,#6598,#201,.T.);
#8228=EDGE_CURVE('',#6514,#6599,#4027,.T.);
#8229=EDGE_CURVE('',#6600,#6599,#4028,.T.);
#8230=EDGE_CURVE('',#6515,#6600,#4029,.T.);
#8231=EDGE_CURVE('',#6601,#6600,#202,.T.);
#8232=EDGE_CURVE('',#6516,#6601,#4030,.T.);
#8233=EDGE_CURVE('',#6602,#6601,#5656,.T.);
#8234=EDGE_CURVE('',#6602,#6517,#4031,.T.);
#8235=EDGE_CURVE('',#6603,#6602,#203,.T.);
#8236=EDGE_CURVE('',#6518,#6603,#4032,.T.);
#8237=EDGE_CURVE('',#6604,#6603,#4033,.T.);
#8238=EDGE_CURVE('',#6519,#6604,#4034,.T.);
#8239=EDGE_CURVE('',#6605,#6604,#204,.T.);
#8240=EDGE_CURVE('',#6520,#6605,#4035,.T.);
#8241=EDGE_CURVE('',#6606,#6605,#5657,.T.);
#8242=EDGE_CURVE('',#6606,#6521,#4036,.T.);
#8243=EDGE_CURVE('',#6607,#6606,#205,.T.);
#8244=EDGE_CURVE('',#6522,#6607,#4037,.T.);
#8245=EDGE_CURVE('',#6608,#6607,#4038,.T.);
#8246=EDGE_CURVE('',#6523,#6608,#4039,.T.);
#8247=EDGE_CURVE('',#6609,#6608,#206,.T.);
#8248=EDGE_CURVE('',#6524,#6609,#4040,.T.);
#8249=EDGE_CURVE('',#6610,#6609,#5658,.T.);
#8250=EDGE_CURVE('',#6610,#6525,#4041,.T.);
#8251=EDGE_CURVE('',#6611,#6610,#207,.T.);
#8252=EDGE_CURVE('',#6526,#6611,#4042,.T.);
#8253=EDGE_CURVE('',#6612,#6611,#4043,.T.);
#8254=EDGE_CURVE('',#6527,#6612,#4044,.T.);
#8255=EDGE_CURVE('',#6613,#6612,#208,.T.);
#8256=EDGE_CURVE('',#6528,#6613,#4045,.T.);
#8257=EDGE_CURVE('',#6614,#6613,#5659,.T.);
#8258=EDGE_CURVE('',#6614,#6529,#4046,.T.);
#8259=EDGE_CURVE('',#6615,#6614,#209,.T.);
#8260=EDGE_CURVE('',#6530,#6615,#4047,.T.);
#8261=EDGE_CURVE('',#6616,#6615,#4048,.T.);
#8262=EDGE_CURVE('',#6531,#6616,#4049,.T.);
#8263=EDGE_CURVE('',#6617,#6616,#210,.T.);
#8264=EDGE_CURVE('',#6532,#6617,#4050,.T.);
#8265=EDGE_CURVE('',#6538,#6617,#5660,.T.);
#10849=ORIENTED_EDGE('',*,*,#8011,.F.);
#10850=ORIENTED_EDGE('',*,*,#8012,.F.);
#10851=ORIENTED_EDGE('',*,*,#8013,.F.);
#10852=ORIENTED_EDGE('',*,*,#8014,.F.);
#10853=ORIENTED_EDGE('',*,*,#8015,.F.);
#10854=ORIENTED_EDGE('',*,*,#8016,.T.);
#10855=ORIENTED_EDGE('',*,*,#8017,.F.);
#10856=ORIENTED_EDGE('',*,*,#8012,.T.);
#10857=ORIENTED_EDGE('',*,*,#8018,.F.);
#10858=ORIENTED_EDGE('',*,*,#8019,.F.);
#10859=ORIENTED_EDGE('',*,*,#8020,.F.);
#10860=ORIENTED_EDGE('',*,*,#8016,.F.);
#10861=ORIENTED_EDGE('',*,*,#8021,.T.);
#10862=ORIENTED_EDGE('',*,*,#8022,.T.);
#10863=ORIENTED_EDGE('',*,*,#8023,.T.);
#10864=ORIENTED_EDGE('',*,*,#8024,.T.);
#10865=ORIENTED_EDGE('',*,*,#8025,.T.);
#10866=ORIENTED_EDGE('',*,*,#8026,.T.);
#10867=ORIENTED_EDGE('',*,*,#8027,.T.);
#10868=ORIENTED_EDGE('',*,*,#8028,.T.);
#10869=ORIENTED_EDGE('',*,*,#8029,.T.);
#10870=ORIENTED_EDGE('',*,*,#8030,.T.);
#10871=ORIENTED_EDGE('',*,*,#8031,.T.);
#10872=ORIENTED_EDGE('',*,*,#8032,.T.);
#10873=ORIENTED_EDGE('',*,*,#8033,.T.);
#10874=ORIENTED_EDGE('',*,*,#8034,.T.);
#10875=ORIENTED_EDGE('',*,*,#8035,.T.);
#10876=ORIENTED_EDGE('',*,*,#8036,.T.);
#10877=ORIENTED_EDGE('',*,*,#8037,.T.);
#10878=ORIENTED_EDGE('',*,*,#8038,.T.);
#10879=ORIENTED_EDGE('',*,*,#8039,.T.);
#10880=ORIENTED_EDGE('',*,*,#8040,.T.);
#10881=ORIENTED_EDGE('',*,*,#8041,.T.);
#10882=ORIENTED_EDGE('',*,*,#8042,.T.);
#10883=ORIENTED_EDGE('',*,*,#8043,.T.);
#10884=ORIENTED_EDGE('',*,*,#8044,.T.);
#10885=ORIENTED_EDGE('',*,*,#8045,.T.);
#10886=ORIENTED_EDGE('',*,*,#8046,.T.);
#10887=ORIENTED_EDGE('',*,*,#8047,.T.);
#10888=ORIENTED_EDGE('',*,*,#8048,.T.);
#10889=ORIENTED_EDGE('',*,*,#8049,.T.);
#10890=ORIENTED_EDGE('',*,*,#8050,.T.);
#10891=ORIENTED_EDGE('',*,*,#8051,.T.);
#10892=ORIENTED_EDGE('',*,*,#8052,.T.);
#10893=ORIENTED_EDGE('',*,*,#8053,.T.);
#10894=ORIENTED_EDGE('',*,*,#8054,.T.);
#10895=ORIENTED_EDGE('',*,*,#8055,.T.);
#10896=ORIENTED_EDGE('',*,*,#8056,.T.);
#10897=ORIENTED_EDGE('',*,*,#8057,.T.);
#10898=ORIENTED_EDGE('',*,*,#8058,.T.);
#10899=ORIENTED_EDGE('',*,*,#8059,.T.);
#10900=ORIENTED_EDGE('',*,*,#8060,.T.);
#10901=ORIENTED_EDGE('',*,*,#8061,.T.);
#10902=ORIENTED_EDGE('',*,*,#8062,.T.);
#10903=ORIENTED_EDGE('',*,*,#8063,.T.);
#10904=ORIENTED_EDGE('',*,*,#8064,.T.);
#10905=ORIENTED_EDGE('',*,*,#8065,.T.);
#10906=ORIENTED_EDGE('',*,*,#8066,.T.);
#10907=ORIENTED_EDGE('',*,*,#8067,.T.);
#10908=ORIENTED_EDGE('',*,*,#8068,.T.);
#10909=ORIENTED_EDGE('',*,*,#8069,.T.);
#10910=ORIENTED_EDGE('',*,*,#8070,.T.);
#10911=ORIENTED_EDGE('',*,*,#8071,.T.);
#10912=ORIENTED_EDGE('',*,*,#8072,.T.);
#10913=ORIENTED_EDGE('',*,*,#8073,.T.);
#10914=ORIENTED_EDGE('',*,*,#8074,.T.);
#10915=ORIENTED_EDGE('',*,*,#8075,.T.);
#10916=ORIENTED_EDGE('',*,*,#8076,.T.);
#10917=ORIENTED_EDGE('',*,*,#8077,.T.);
#10918=ORIENTED_EDGE('',*,*,#8078,.T.);
#10919=ORIENTED_EDGE('',*,*,#8079,.T.);
#10920=ORIENTED_EDGE('',*,*,#8080,.T.);
#10921=ORIENTED_EDGE('',*,*,#8081,.T.);
#10922=ORIENTED_EDGE('',*,*,#8082,.T.);
#10923=ORIENTED_EDGE('',*,*,#8083,.T.);
#10924=ORIENTED_EDGE('',*,*,#8084,.T.);
#10925=ORIENTED_EDGE('',*,*,#8085,.T.);
#10926=ORIENTED_EDGE('',*,*,#8086,.T.);
#10927=ORIENTED_EDGE('',*,*,#8087,.T.);
#10928=ORIENTED_EDGE('',*,*,#8088,.T.);
#10929=ORIENTED_EDGE('',*,*,#8089,.T.);
#10930=ORIENTED_EDGE('',*,*,#8090,.T.);
#10931=ORIENTED_EDGE('',*,*,#8091,.T.);
#10932=ORIENTED_EDGE('',*,*,#8092,.T.);
#10933=ORIENTED_EDGE('',*,*,#8093,.T.);
#10934=ORIENTED_EDGE('',*,*,#8094,.T.);
#10935=ORIENTED_EDGE('',*,*,#8095,.T.);
#10936=ORIENTED_EDGE('',*,*,#8096,.T.);
#10937=ORIENTED_EDGE('',*,*,#8097,.T.);
#10938=ORIENTED_EDGE('',*,*,#8098,.T.);
#10939=ORIENTED_EDGE('',*,*,#8099,.T.);
#10940=ORIENTED_EDGE('',*,*,#8100,.T.);
#10941=ORIENTED_EDGE('',*,*,#8013,.T.);
#10942=ORIENTED_EDGE('',*,*,#8017,.T.);
#10943=ORIENTED_EDGE('',*,*,#8020,.T.);
#10944=ORIENTED_EDGE('',*,*,#8101,.T.);
#10945=ORIENTED_EDGE('',*,*,#8014,.T.);
#10946=ORIENTED_EDGE('',*,*,#8101,.F.);
#10947=ORIENTED_EDGE('',*,*,#8019,.T.);
#10948=ORIENTED_EDGE('',*,*,#8102,.F.);
#10949=ORIENTED_EDGE('',*,*,#8103,.F.);
#10950=ORIENTED_EDGE('',*,*,#8104,.T.);
#10951=ORIENTED_EDGE('',*,*,#8105,.F.);
#10952=ORIENTED_EDGE('',*,*,#8104,.F.);
#10953=ORIENTED_EDGE('',*,*,#8103,.T.);
#10954=ORIENTED_EDGE('',*,*,#8011,.T.);
#10955=ORIENTED_EDGE('',*,*,#8102,.T.);
#10956=ORIENTED_EDGE('',*,*,#8018,.T.);
#10957=ORIENTED_EDGE('',*,*,#8015,.T.);
#10958=ORIENTED_EDGE('',*,*,#8106,.F.);
#10959=ORIENTED_EDGE('',*,*,#8107,.F.);
#10960=ORIENTED_EDGE('',*,*,#8108,.F.);
#10961=ORIENTED_EDGE('',*,*,#8098,.F.);
#10962=ORIENTED_EDGE('',*,*,#8108,.T.);
#10963=ORIENTED_EDGE('',*,*,#8109,.F.);
#10964=ORIENTED_EDGE('',*,*,#8110,.F.);
#10965=ORIENTED_EDGE('',*,*,#8099,.F.);
#10966=ORIENTED_EDGE('',*,*,#8110,.T.);
#10967=ORIENTED_EDGE('',*,*,#8111,.F.);
#10968=ORIENTED_EDGE('',*,*,#8112,.F.);
#10969=ORIENTED_EDGE('',*,*,#8100,.F.);
#10970=ORIENTED_EDGE('',*,*,#8112,.T.);
#10971=ORIENTED_EDGE('',*,*,#8113,.F.);
#10972=ORIENTED_EDGE('',*,*,#8114,.T.);
#10973=ORIENTED_EDGE('',*,*,#8021,.F.);
#10974=ORIENTED_EDGE('',*,*,#8114,.F.);
#10975=ORIENTED_EDGE('',*,*,#8115,.F.);
#10976=ORIENTED_EDGE('',*,*,#8116,.F.);
#10977=ORIENTED_EDGE('',*,*,#8022,.F.);
#10978=ORIENTED_EDGE('',*,*,#8116,.T.);
#10979=ORIENTED_EDGE('',*,*,#8117,.F.);
#10980=ORIENTED_EDGE('',*,*,#8118,.F.);
#10981=ORIENTED_EDGE('',*,*,#8023,.F.);
#10982=ORIENTED_EDGE('',*,*,#8118,.T.);
#10983=ORIENTED_EDGE('',*,*,#8119,.F.);
#10984=ORIENTED_EDGE('',*,*,#8120,.F.);
#10985=ORIENTED_EDGE('',*,*,#8024,.F.);
#10986=ORIENTED_EDGE('',*,*,#8120,.T.);
#10987=ORIENTED_EDGE('',*,*,#8121,.F.);
#10988=ORIENTED_EDGE('',*,*,#8122,.T.);
#10989=ORIENTED_EDGE('',*,*,#8025,.F.);
#10990=ORIENTED_EDGE('',*,*,#8122,.F.);
#10991=ORIENTED_EDGE('',*,*,#8123,.F.);
#10992=ORIENTED_EDGE('',*,*,#8124,.F.);
#10993=ORIENTED_EDGE('',*,*,#8026,.F.);
#10994=ORIENTED_EDGE('',*,*,#8124,.T.);
#10995=ORIENTED_EDGE('',*,*,#8125,.F.);
#10996=ORIENTED_EDGE('',*,*,#8126,.F.);
#10997=ORIENTED_EDGE('',*,*,#8027,.F.);
#10998=ORIENTED_EDGE('',*,*,#8126,.T.);
#10999=ORIENTED_EDGE('',*,*,#8127,.F.);
#11000=ORIENTED_EDGE('',*,*,#8128,.F.);
#11001=ORIENTED_EDGE('',*,*,#8028,.F.);
#11002=ORIENTED_EDGE('',*,*,#8128,.T.);
#11003=ORIENTED_EDGE('',*,*,#8129,.F.);
#11004=ORIENTED_EDGE('',*,*,#8130,.T.);
#11005=ORIENTED_EDGE('',*,*,#8029,.F.);
#11006=ORIENTED_EDGE('',*,*,#8130,.F.);
#11007=ORIENTED_EDGE('',*,*,#8131,.F.);
#11008=ORIENTED_EDGE('',*,*,#8132,.F.);
#11009=ORIENTED_EDGE('',*,*,#8030,.F.);
#11010=ORIENTED_EDGE('',*,*,#8132,.T.);
#11011=ORIENTED_EDGE('',*,*,#8133,.F.);
#11012=ORIENTED_EDGE('',*,*,#8134,.F.);
#11013=ORIENTED_EDGE('',*,*,#8031,.F.);
#11014=ORIENTED_EDGE('',*,*,#8134,.T.);
#11015=ORIENTED_EDGE('',*,*,#8135,.F.);
#11016=ORIENTED_EDGE('',*,*,#8136,.F.);
#11017=ORIENTED_EDGE('',*,*,#8032,.F.);
#11018=ORIENTED_EDGE('',*,*,#8136,.T.);
#11019=ORIENTED_EDGE('',*,*,#8137,.F.);
#11020=ORIENTED_EDGE('',*,*,#8138,.T.);
#11021=ORIENTED_EDGE('',*,*,#8033,.F.);
#11022=ORIENTED_EDGE('',*,*,#8138,.F.);
#11023=ORIENTED_EDGE('',*,*,#8139,.F.);
#11024=ORIENTED_EDGE('',*,*,#8140,.F.);
#11025=ORIENTED_EDGE('',*,*,#8034,.F.);
#11026=ORIENTED_EDGE('',*,*,#8140,.T.);
#11027=ORIENTED_EDGE('',*,*,#8141,.F.);
#11028=ORIENTED_EDGE('',*,*,#8142,.F.);
#11029=ORIENTED_EDGE('',*,*,#8035,.F.);
#11030=ORIENTED_EDGE('',*,*,#8142,.T.);
#11031=ORIENTED_EDGE('',*,*,#8143,.F.);
#11032=ORIENTED_EDGE('',*,*,#8144,.F.);
#11033=ORIENTED_EDGE('',*,*,#8036,.F.);
#11034=ORIENTED_EDGE('',*,*,#8144,.T.);
#11035=ORIENTED_EDGE('',*,*,#8145,.F.);
#11036=ORIENTED_EDGE('',*,*,#8146,.T.);
#11037=ORIENTED_EDGE('',*,*,#8037,.F.);
#11038=ORIENTED_EDGE('',*,*,#8146,.F.);
#11039=ORIENTED_EDGE('',*,*,#8147,.F.);
#11040=ORIENTED_EDGE('',*,*,#8148,.F.);
#11041=ORIENTED_EDGE('',*,*,#8038,.F.);
#11042=ORIENTED_EDGE('',*,*,#8148,.T.);
#11043=ORIENTED_EDGE('',*,*,#8149,.F.);
#11044=ORIENTED_EDGE('',*,*,#8150,.F.);
#11045=ORIENTED_EDGE('',*,*,#8039,.F.);
#11046=ORIENTED_EDGE('',*,*,#8150,.T.);
#11047=ORIENTED_EDGE('',*,*,#8151,.F.);
#11048=ORIENTED_EDGE('',*,*,#8152,.F.);
#11049=ORIENTED_EDGE('',*,*,#8040,.F.);
#11050=ORIENTED_EDGE('',*,*,#8152,.T.);
#11051=ORIENTED_EDGE('',*,*,#8153,.F.);
#11052=ORIENTED_EDGE('',*,*,#8154,.T.);
#11053=ORIENTED_EDGE('',*,*,#8041,.F.);
#11054=ORIENTED_EDGE('',*,*,#8154,.F.);
#11055=ORIENTED_EDGE('',*,*,#8155,.F.);
#11056=ORIENTED_EDGE('',*,*,#8156,.F.);
#11057=ORIENTED_EDGE('',*,*,#8042,.F.);
#11058=ORIENTED_EDGE('',*,*,#8156,.T.);
#11059=ORIENTED_EDGE('',*,*,#8157,.F.);
#11060=ORIENTED_EDGE('',*,*,#8158,.F.);
#11061=ORIENTED_EDGE('',*,*,#8043,.F.);
#11062=ORIENTED_EDGE('',*,*,#8158,.T.);
#11063=ORIENTED_EDGE('',*,*,#8159,.F.);
#11064=ORIENTED_EDGE('',*,*,#8160,.F.);
#11065=ORIENTED_EDGE('',*,*,#8044,.F.);
#11066=ORIENTED_EDGE('',*,*,#8160,.T.);
#11067=ORIENTED_EDGE('',*,*,#8161,.F.);
#11068=ORIENTED_EDGE('',*,*,#8162,.T.);
#11069=ORIENTED_EDGE('',*,*,#8045,.F.);
#11070=ORIENTED_EDGE('',*,*,#8162,.F.);
#11071=ORIENTED_EDGE('',*,*,#8163,.F.);
#11072=ORIENTED_EDGE('',*,*,#8164,.F.);
#11073=ORIENTED_EDGE('',*,*,#8046,.F.);
#11074=ORIENTED_EDGE('',*,*,#8164,.T.);
#11075=ORIENTED_EDGE('',*,*,#8165,.F.);
#11076=ORIENTED_EDGE('',*,*,#8166,.F.);
#11077=ORIENTED_EDGE('',*,*,#8047,.F.);
#11078=ORIENTED_EDGE('',*,*,#8166,.T.);
#11079=ORIENTED_EDGE('',*,*,#8167,.F.);
#11080=ORIENTED_EDGE('',*,*,#8168,.F.);
#11081=ORIENTED_EDGE('',*,*,#8048,.F.);
#11082=ORIENTED_EDGE('',*,*,#8168,.T.);
#11083=ORIENTED_EDGE('',*,*,#8169,.F.);
#11084=ORIENTED_EDGE('',*,*,#8170,.T.);
#11085=ORIENTED_EDGE('',*,*,#8049,.F.);
#11086=ORIENTED_EDGE('',*,*,#8170,.F.);
#11087=ORIENTED_EDGE('',*,*,#8171,.F.);
#11088=ORIENTED_EDGE('',*,*,#8172,.F.);
#11089=ORIENTED_EDGE('',*,*,#8050,.F.);
#11090=ORIENTED_EDGE('',*,*,#8172,.T.);
#11091=ORIENTED_EDGE('',*,*,#8173,.F.);
#11092=ORIENTED_EDGE('',*,*,#8174,.F.);
#11093=ORIENTED_EDGE('',*,*,#8051,.F.);
#11094=ORIENTED_EDGE('',*,*,#8174,.T.);
#11095=ORIENTED_EDGE('',*,*,#8175,.F.);
#11096=ORIENTED_EDGE('',*,*,#8176,.F.);
#11097=ORIENTED_EDGE('',*,*,#8052,.F.);
#11098=ORIENTED_EDGE('',*,*,#8176,.T.);
#11099=ORIENTED_EDGE('',*,*,#8177,.F.);
#11100=ORIENTED_EDGE('',*,*,#8178,.T.);
#11101=ORIENTED_EDGE('',*,*,#8053,.F.);
#11102=ORIENTED_EDGE('',*,*,#8178,.F.);
#11103=ORIENTED_EDGE('',*,*,#8179,.F.);
#11104=ORIENTED_EDGE('',*,*,#8180,.F.);
#11105=ORIENTED_EDGE('',*,*,#8054,.F.);
#11106=ORIENTED_EDGE('',*,*,#8180,.T.);
#11107=ORIENTED_EDGE('',*,*,#8181,.F.);
#11108=ORIENTED_EDGE('',*,*,#8182,.F.);
#11109=ORIENTED_EDGE('',*,*,#8055,.F.);
#11110=ORIENTED_EDGE('',*,*,#8182,.T.);
#11111=ORIENTED_EDGE('',*,*,#8183,.F.);
#11112=ORIENTED_EDGE('',*,*,#8184,.F.);
#11113=ORIENTED_EDGE('',*,*,#8056,.F.);
#11114=ORIENTED_EDGE('',*,*,#8184,.T.);
#11115=ORIENTED_EDGE('',*,*,#8185,.F.);
#11116=ORIENTED_EDGE('',*,*,#8186,.T.);
#11117=ORIENTED_EDGE('',*,*,#8057,.F.);
#11118=ORIENTED_EDGE('',*,*,#8186,.F.);
#11119=ORIENTED_EDGE('',*,*,#8187,.F.);
#11120=ORIENTED_EDGE('',*,*,#8188,.F.);
#11121=ORIENTED_EDGE('',*,*,#8058,.F.);
#11122=ORIENTED_EDGE('',*,*,#8188,.T.);
#11123=ORIENTED_EDGE('',*,*,#8189,.F.);
#11124=ORIENTED_EDGE('',*,*,#8190,.F.);
#11125=ORIENTED_EDGE('',*,*,#8059,.F.);
#11126=ORIENTED_EDGE('',*,*,#8190,.T.);
#11127=ORIENTED_EDGE('',*,*,#8191,.F.);
#11128=ORIENTED_EDGE('',*,*,#8192,.F.);
#11129=ORIENTED_EDGE('',*,*,#8060,.F.);
#11130=ORIENTED_EDGE('',*,*,#8192,.T.);
#11131=ORIENTED_EDGE('',*,*,#8193,.F.);
#11132=ORIENTED_EDGE('',*,*,#8194,.T.);
#11133=ORIENTED_EDGE('',*,*,#8061,.F.);
#11134=ORIENTED_EDGE('',*,*,#8194,.F.);
#11135=ORIENTED_EDGE('',*,*,#8195,.F.);
#11136=ORIENTED_EDGE('',*,*,#8196,.F.);
#11137=ORIENTED_EDGE('',*,*,#8062,.F.);
#11138=ORIENTED_EDGE('',*,*,#8196,.T.);
#11139=ORIENTED_EDGE('',*,*,#8197,.F.);
#11140=ORIENTED_EDGE('',*,*,#8198,.F.);
#11141=ORIENTED_EDGE('',*,*,#8063,.F.);
#11142=ORIENTED_EDGE('',*,*,#8198,.T.);
#11143=ORIENTED_EDGE('',*,*,#8199,.F.);
#11144=ORIENTED_EDGE('',*,*,#8200,.F.);
#11145=ORIENTED_EDGE('',*,*,#8064,.F.);
#11146=ORIENTED_EDGE('',*,*,#8200,.T.);
#11147=ORIENTED_EDGE('',*,*,#8201,.F.);
#11148=ORIENTED_EDGE('',*,*,#8202,.T.);
#11149=ORIENTED_EDGE('',*,*,#8065,.F.);
#11150=ORIENTED_EDGE('',*,*,#8202,.F.);
#11151=ORIENTED_EDGE('',*,*,#8203,.F.);
#11152=ORIENTED_EDGE('',*,*,#8204,.F.);
#11153=ORIENTED_EDGE('',*,*,#8066,.F.);
#11154=ORIENTED_EDGE('',*,*,#8204,.T.);
#11155=ORIENTED_EDGE('',*,*,#8205,.F.);
#11156=ORIENTED_EDGE('',*,*,#8206,.F.);
#11157=ORIENTED_EDGE('',*,*,#8067,.F.);
#11158=ORIENTED_EDGE('',*,*,#8206,.T.);
#11159=ORIENTED_EDGE('',*,*,#8207,.F.);
#11160=ORIENTED_EDGE('',*,*,#8208,.F.);
#11161=ORIENTED_EDGE('',*,*,#8068,.F.);
#11162=ORIENTED_EDGE('',*,*,#8208,.T.);
#11163=ORIENTED_EDGE('',*,*,#8209,.F.);
#11164=ORIENTED_EDGE('',*,*,#8210,.T.);
#11165=ORIENTED_EDGE('',*,*,#8069,.F.);
#11166=ORIENTED_EDGE('',*,*,#8210,.F.);
#11167=ORIENTED_EDGE('',*,*,#8211,.F.);
#11168=ORIENTED_EDGE('',*,*,#8212,.F.);
#11169=ORIENTED_EDGE('',*,*,#8070,.F.);
#11170=ORIENTED_EDGE('',*,*,#8212,.T.);
#11171=ORIENTED_EDGE('',*,*,#8213,.F.);
#11172=ORIENTED_EDGE('',*,*,#8214,.F.);
#11173=ORIENTED_EDGE('',*,*,#8071,.F.);
#11174=ORIENTED_EDGE('',*,*,#8214,.T.);
#11175=ORIENTED_EDGE('',*,*,#8215,.F.);
#11176=ORIENTED_EDGE('',*,*,#8216,.F.);
#11177=ORIENTED_EDGE('',*,*,#8072,.F.);
#11178=ORIENTED_EDGE('',*,*,#8216,.T.);
#11179=ORIENTED_EDGE('',*,*,#8217,.F.);
#11180=ORIENTED_EDGE('',*,*,#8218,.T.);
#11181=ORIENTED_EDGE('',*,*,#8073,.F.);
#11182=ORIENTED_EDGE('',*,*,#8218,.F.);
#11183=ORIENTED_EDGE('',*,*,#8219,.F.);
#11184=ORIENTED_EDGE('',*,*,#8220,.F.);
#11185=ORIENTED_EDGE('',*,*,#8074,.F.);
#11186=ORIENTED_EDGE('',*,*,#8220,.T.);
#11187=ORIENTED_EDGE('',*,*,#8221,.F.);
#11188=ORIENTED_EDGE('',*,*,#8222,.F.);
#11189=ORIENTED_EDGE('',*,*,#8075,.F.);
#11190=ORIENTED_EDGE('',*,*,#8222,.T.);
#11191=ORIENTED_EDGE('',*,*,#8223,.F.);
#11192=ORIENTED_EDGE('',*,*,#8224,.F.);
#11193=ORIENTED_EDGE('',*,*,#8076,.F.);
#11194=ORIENTED_EDGE('',*,*,#8224,.T.);
#11195=ORIENTED_EDGE('',*,*,#8225,.F.);
#11196=ORIENTED_EDGE('',*,*,#8226,.T.);
#11197=ORIENTED_EDGE('',*,*,#8077,.F.);
#11198=ORIENTED_EDGE('',*,*,#8226,.F.);
#11199=ORIENTED_EDGE('',*,*,#8227,.F.);
#11200=ORIENTED_EDGE('',*,*,#8228,.F.);
#11201=ORIENTED_EDGE('',*,*,#8078,.F.);
#11202=ORIENTED_EDGE('',*,*,#8228,.T.);
#11203=ORIENTED_EDGE('',*,*,#8229,.F.);
#11204=ORIENTED_EDGE('',*,*,#8230,.F.);
#11205=ORIENTED_EDGE('',*,*,#8079,.F.);
#11206=ORIENTED_EDGE('',*,*,#8230,.T.);
#11207=ORIENTED_EDGE('',*,*,#8231,.F.);
#11208=ORIENTED_EDGE('',*,*,#8232,.F.);
#11209=ORIENTED_EDGE('',*,*,#8080,.F.);
#11210=ORIENTED_EDGE('',*,*,#8232,.T.);
#11211=ORIENTED_EDGE('',*,*,#8233,.F.);
#11212=ORIENTED_EDGE('',*,*,#8234,.T.);
#11213=ORIENTED_EDGE('',*,*,#8081,.F.);
#11214=ORIENTED_EDGE('',*,*,#8234,.F.);
#11215=ORIENTED_EDGE('',*,*,#8235,.F.);
#11216=ORIENTED_EDGE('',*,*,#8236,.F.);
#11217=ORIENTED_EDGE('',*,*,#8082,.F.);
#11218=ORIENTED_EDGE('',*,*,#8236,.T.);
#11219=ORIENTED_EDGE('',*,*,#8237,.F.);
#11220=ORIENTED_EDGE('',*,*,#8238,.F.);
#11221=ORIENTED_EDGE('',*,*,#8083,.F.);
#11222=ORIENTED_EDGE('',*,*,#8238,.T.);
#11223=ORIENTED_EDGE('',*,*,#8239,.F.);
#11224=ORIENTED_EDGE('',*,*,#8240,.F.);
#11225=ORIENTED_EDGE('',*,*,#8084,.F.);
#11226=ORIENTED_EDGE('',*,*,#8240,.T.);
#11227=ORIENTED_EDGE('',*,*,#8241,.F.);
#11228=ORIENTED_EDGE('',*,*,#8242,.T.);
#11229=ORIENTED_EDGE('',*,*,#8085,.F.);
#11230=ORIENTED_EDGE('',*,*,#8242,.F.);
#11231=ORIENTED_EDGE('',*,*,#8243,.F.);
#11232=ORIENTED_EDGE('',*,*,#8244,.F.);
#11233=ORIENTED_EDGE('',*,*,#8086,.F.);
#11234=ORIENTED_EDGE('',*,*,#8244,.T.);
#11235=ORIENTED_EDGE('',*,*,#8245,.F.);
#11236=ORIENTED_EDGE('',*,*,#8246,.F.);
#11237=ORIENTED_EDGE('',*,*,#8087,.F.);
#11238=ORIENTED_EDGE('',*,*,#8246,.T.);
#11239=ORIENTED_EDGE('',*,*,#8247,.F.);
#11240=ORIENTED_EDGE('',*,*,#8248,.F.);
#11241=ORIENTED_EDGE('',*,*,#8088,.F.);
#11242=ORIENTED_EDGE('',*,*,#8248,.T.);
#11243=ORIENTED_EDGE('',*,*,#8249,.F.);
#11244=ORIENTED_EDGE('',*,*,#8250,.T.);
#11245=ORIENTED_EDGE('',*,*,#8089,.F.);
#11246=ORIENTED_EDGE('',*,*,#8250,.F.);
#11247=ORIENTED_EDGE('',*,*,#8251,.F.);
#11248=ORIENTED_EDGE('',*,*,#8252,.F.);
#11249=ORIENTED_EDGE('',*,*,#8090,.F.);
#11250=ORIENTED_EDGE('',*,*,#8252,.T.);
#11251=ORIENTED_EDGE('',*,*,#8253,.F.);
#11252=ORIENTED_EDGE('',*,*,#8254,.F.);
#11253=ORIENTED_EDGE('',*,*,#8091,.F.);
#11254=ORIENTED_EDGE('',*,*,#8254,.T.);
#11255=ORIENTED_EDGE('',*,*,#8255,.F.);
#11256=ORIENTED_EDGE('',*,*,#8256,.F.);
#11257=ORIENTED_EDGE('',*,*,#8092,.F.);
#11258=ORIENTED_EDGE('',*,*,#8256,.T.);
#11259=ORIENTED_EDGE('',*,*,#8257,.F.);
#11260=ORIENTED_EDGE('',*,*,#8258,.T.);
#11261=ORIENTED_EDGE('',*,*,#8093,.F.);
#11262=ORIENTED_EDGE('',*,*,#8258,.F.);
#11263=ORIENTED_EDGE('',*,*,#8259,.F.);
#11264=ORIENTED_EDGE('',*,*,#8260,.F.);
#11265=ORIENTED_EDGE('',*,*,#8094,.F.);
#11266=ORIENTED_EDGE('',*,*,#8260,.T.);
#11267=ORIENTED_EDGE('',*,*,#8261,.F.);
#11268=ORIENTED_EDGE('',*,*,#8262,.F.);
#11269=ORIENTED_EDGE('',*,*,#8095,.F.);
#11270=ORIENTED_EDGE('',*,*,#8262,.T.);
#11271=ORIENTED_EDGE('',*,*,#8263,.F.);
#11272=ORIENTED_EDGE('',*,*,#8264,.F.);
#11273=ORIENTED_EDGE('',*,*,#8096,.F.);
#11274=ORIENTED_EDGE('',*,*,#8265,.T.);
#11275=ORIENTED_EDGE('',*,*,#8263,.T.);
#11276=ORIENTED_EDGE('',*,*,#8261,.T.);
#11277=ORIENTED_EDGE('',*,*,#8259,.T.);
#11278=ORIENTED_EDGE('',*,*,#8257,.T.);
#11279=ORIENTED_EDGE('',*,*,#8255,.T.);
#11280=ORIENTED_EDGE('',*,*,#8253,.T.);
#11281=ORIENTED_EDGE('',*,*,#8251,.T.);
#11282=ORIENTED_EDGE('',*,*,#8249,.T.);
#11283=ORIENTED_EDGE('',*,*,#8247,.T.);
#11284=ORIENTED_EDGE('',*,*,#8245,.T.);
#11285=ORIENTED_EDGE('',*,*,#8243,.T.);
#11286=ORIENTED_EDGE('',*,*,#8241,.T.);
#11287=ORIENTED_EDGE('',*,*,#8239,.T.);
#11288=ORIENTED_EDGE('',*,*,#8237,.T.);
#11289=ORIENTED_EDGE('',*,*,#8235,.T.);
#11290=ORIENTED_EDGE('',*,*,#8233,.T.);
#11291=ORIENTED_EDGE('',*,*,#8231,.T.);
#11292=ORIENTED_EDGE('',*,*,#8229,.T.);
#11293=ORIENTED_EDGE('',*,*,#8227,.T.);
#11294=ORIENTED_EDGE('',*,*,#8225,.T.);
#11295=ORIENTED_EDGE('',*,*,#8223,.T.);
#11296=ORIENTED_EDGE('',*,*,#8221,.T.);
#11297=ORIENTED_EDGE('',*,*,#8219,.T.);
#11298=ORIENTED_EDGE('',*,*,#8217,.T.);
#11299=ORIENTED_EDGE('',*,*,#8215,.T.);
#11300=ORIENTED_EDGE('',*,*,#8213,.T.);
#11301=ORIENTED_EDGE('',*,*,#8211,.T.);
#11302=ORIENTED_EDGE('',*,*,#8209,.T.);
#11303=ORIENTED_EDGE('',*,*,#8207,.T.);
#11304=ORIENTED_EDGE('',*,*,#8205,.T.);
#11305=ORIENTED_EDGE('',*,*,#8203,.T.);
#11306=ORIENTED_EDGE('',*,*,#8201,.T.);
#11307=ORIENTED_EDGE('',*,*,#8199,.T.);
#11308=ORIENTED_EDGE('',*,*,#8197,.T.);
#11309=ORIENTED_EDGE('',*,*,#8195,.T.);
#11310=ORIENTED_EDGE('',*,*,#8193,.T.);
#11311=ORIENTED_EDGE('',*,*,#8191,.T.);
#11312=ORIENTED_EDGE('',*,*,#8189,.T.);
#11313=ORIENTED_EDGE('',*,*,#8187,.T.);
#11314=ORIENTED_EDGE('',*,*,#8185,.T.);
#11315=ORIENTED_EDGE('',*,*,#8183,.T.);
#11316=ORIENTED_EDGE('',*,*,#8181,.T.);
#11317=ORIENTED_EDGE('',*,*,#8179,.T.);
#11318=ORIENTED_EDGE('',*,*,#8177,.T.);
#11319=ORIENTED_EDGE('',*,*,#8175,.T.);
#11320=ORIENTED_EDGE('',*,*,#8173,.T.);
#11321=ORIENTED_EDGE('',*,*,#8171,.T.);
#11322=ORIENTED_EDGE('',*,*,#8169,.T.);
#11323=ORIENTED_EDGE('',*,*,#8167,.T.);
#11324=ORIENTED_EDGE('',*,*,#8165,.T.);
#11325=ORIENTED_EDGE('',*,*,#8163,.T.);
#11326=ORIENTED_EDGE('',*,*,#8161,.T.);
#11327=ORIENTED_EDGE('',*,*,#8159,.T.);
#11328=ORIENTED_EDGE('',*,*,#8157,.T.);
#11329=ORIENTED_EDGE('',*,*,#8155,.T.);
#11330=ORIENTED_EDGE('',*,*,#8153,.T.);
#11331=ORIENTED_EDGE('',*,*,#8151,.T.);
#11332=ORIENTED_EDGE('',*,*,#8149,.T.);
#11333=ORIENTED_EDGE('',*,*,#8147,.T.);
#11334=ORIENTED_EDGE('',*,*,#8145,.T.);
#11335=ORIENTED_EDGE('',*,*,#8143,.T.);
#11336=ORIENTED_EDGE('',*,*,#8141,.T.);
#11337=ORIENTED_EDGE('',*,*,#8139,.T.);
#11338=ORIENTED_EDGE('',*,*,#8137,.T.);
#11339=ORIENTED_EDGE('',*,*,#8135,.T.);
#11340=ORIENTED_EDGE('',*,*,#8133,.T.);
#11341=ORIENTED_EDGE('',*,*,#8131,.T.);
#11342=ORIENTED_EDGE('',*,*,#8129,.T.);
#11343=ORIENTED_EDGE('',*,*,#8127,.T.);
#11344=ORIENTED_EDGE('',*,*,#8125,.T.);
#11345=ORIENTED_EDGE('',*,*,#8123,.T.);
#11346=ORIENTED_EDGE('',*,*,#8121,.T.);
#11347=ORIENTED_EDGE('',*,*,#8119,.T.);
#11348=ORIENTED_EDGE('',*,*,#8117,.T.);
#11349=ORIENTED_EDGE('',*,*,#8115,.T.);
#11350=ORIENTED_EDGE('',*,*,#8113,.T.);
#11351=ORIENTED_EDGE('',*,*,#8111,.T.);
#11352=ORIENTED_EDGE('',*,*,#8109,.T.);
#11353=ORIENTED_EDGE('',*,*,#8107,.T.);
#11354=ORIENTED_EDGE('',*,*,#8105,.T.);
#11355=ORIENTED_EDGE('',*,*,#8106,.T.);
#11356=ORIENTED_EDGE('',*,*,#8097,.F.);
#11357=ORIENTED_EDGE('',*,*,#8264,.T.);
#11358=ORIENTED_EDGE('',*,*,#8265,.F.);
#12731=CYLINDRICAL_SURFACE('',#15154,0.6);
#12732=CYLINDRICAL_SURFACE('',#15156,1.4);
#12733=CYLINDRICAL_SURFACE('',#15161,1.75);
#12734=CYLINDRICAL_SURFACE('',#15164,1.75);
#12735=CYLINDRICAL_SURFACE('',#15167,1.75);
#12736=CYLINDRICAL_SURFACE('',#15170,1.75);
#12737=CYLINDRICAL_SURFACE('',#15173,1.75);
#12738=CYLINDRICAL_SURFACE('',#15176,1.75);
#12739=CYLINDRICAL_SURFACE('',#15179,1.75);
#12740=CYLINDRICAL_SURFACE('',#15182,1.75);
#12741=CYLINDRICAL_SURFACE('',#15185,1.75);
#12742=CYLINDRICAL_SURFACE('',#15188,1.75);
#12743=CYLINDRICAL_SURFACE('',#15191,1.75);
#12744=CYLINDRICAL_SURFACE('',#15194,1.75);
#12745=CYLINDRICAL_SURFACE('',#15197,1.75);
#12746=CYLINDRICAL_SURFACE('',#15200,1.75);
#12747=CYLINDRICAL_SURFACE('',#15203,1.75);
#12748=CYLINDRICAL_SURFACE('',#15206,1.75);
#12749=CYLINDRICAL_SURFACE('',#15209,1.75);
#12750=CYLINDRICAL_SURFACE('',#15212,1.75);
#12751=CYLINDRICAL_SURFACE('',#15215,1.75);
#12752=CYLINDRICAL_SURFACE('',#15220,1.75);
#13256=ADVANCED_FACE('',(#2139),#1578,.F.);
#13257=ADVANCED_FACE('',(#2140),#1579,.F.);
#13258=ADVANCED_FACE('',(#2141),#1580,.F.);
#13259=ADVANCED_FACE('',(#2142,#1308),#1581,.F.);
#13260=ADVANCED_FACE('',(#2143),#12731,.F.);
#13261=ADVANCED_FACE('',(#2144),#12732,.T.);
#13262=ADVANCED_FACE('',(#2145,#1309),#1582,.T.);
#13263=ADVANCED_FACE('',(#2146),#11,.T.);
#13264=ADVANCED_FACE('',(#2147),#1583,.T.);
#13265=ADVANCED_FACE('',(#2148),#12,.T.);
#13266=ADVANCED_FACE('',(#2149),#12733,.T.);
#13267=ADVANCED_FACE('',(#2150),#13,.T.);
#13268=ADVANCED_FACE('',(#2151),#1584,.T.);
#13269=ADVANCED_FACE('',(#2152),#14,.T.);
#13270=ADVANCED_FACE('',(#2153),#12734,.T.);
#13271=ADVANCED_FACE('',(#2154),#15,.T.);
#13272=ADVANCED_FACE('',(#2155),#1585,.T.);
#13273=ADVANCED_FACE('',(#2156),#16,.T.);
#13274=ADVANCED_FACE('',(#2157),#12735,.T.);
#13275=ADVANCED_FACE('',(#2158),#17,.T.);
#13276=ADVANCED_FACE('',(#2159),#1586,.T.);
#13277=ADVANCED_FACE('',(#2160),#18,.T.);
#13278=ADVANCED_FACE('',(#2161),#12736,.T.);
#13279=ADVANCED_FACE('',(#2162),#19,.T.);
#13280=ADVANCED_FACE('',(#2163),#1587,.T.);
#13281=ADVANCED_FACE('',(#2164),#20,.T.);
#13282=ADVANCED_FACE('',(#2165),#12737,.T.);
#13283=ADVANCED_FACE('',(#2166),#21,.T.);
#13284=ADVANCED_FACE('',(#2167),#1588,.T.);
#13285=ADVANCED_FACE('',(#2168),#22,.T.);
#13286=ADVANCED_FACE('',(#2169),#12738,.T.);
#13287=ADVANCED_FACE('',(#2170),#23,.T.);
#13288=ADVANCED_FACE('',(#2171),#1589,.T.);
#13289=ADVANCED_FACE('',(#2172),#24,.T.);
#13290=ADVANCED_FACE('',(#2173),#12739,.T.);
#13291=ADVANCED_FACE('',(#2174),#25,.T.);
#13292=ADVANCED_FACE('',(#2175),#1590,.T.);
#13293=ADVANCED_FACE('',(#2176),#26,.T.);
#13294=ADVANCED_FACE('',(#2177),#12740,.T.);
#13295=ADVANCED_FACE('',(#2178),#27,.T.);
#13296=ADVANCED_FACE('',(#2179),#1591,.T.);
#13297=ADVANCED_FACE('',(#2180),#28,.T.);
#13298=ADVANCED_FACE('',(#2181),#12741,.T.);
#13299=ADVANCED_FACE('',(#2182),#29,.T.);
#13300=ADVANCED_FACE('',(#2183),#1592,.T.);
#13301=ADVANCED_FACE('',(#2184),#30,.T.);
#13302=ADVANCED_FACE('',(#2185),#12742,.T.);
#13303=ADVANCED_FACE('',(#2186),#31,.T.);
#13304=ADVANCED_FACE('',(#2187),#1593,.T.);
#13305=ADVANCED_FACE('',(#2188),#32,.T.);
#13306=ADVANCED_FACE('',(#2189),#12743,.T.);
#13307=ADVANCED_FACE('',(#2190),#33,.T.);
#13308=ADVANCED_FACE('',(#2191),#1594,.T.);
#13309=ADVANCED_FACE('',(#2192),#34,.T.);
#13310=ADVANCED_FACE('',(#2193),#12744,.T.);
#13311=ADVANCED_FACE('',(#2194),#35,.T.);
#13312=ADVANCED_FACE('',(#2195),#1595,.T.);
#13313=ADVANCED_FACE('',(#2196),#36,.T.);
#13314=ADVANCED_FACE('',(#2197),#12745,.T.);
#13315=ADVANCED_FACE('',(#2198),#37,.T.);
#13316=ADVANCED_FACE('',(#2199),#1596,.T.);
#13317=ADVANCED_FACE('',(#2200),#38,.T.);
#13318=ADVANCED_FACE('',(#2201),#12746,.T.);
#13319=ADVANCED_FACE('',(#2202),#39,.T.);
#13320=ADVANCED_FACE('',(#2203),#1597,.T.);
#13321=ADVANCED_FACE('',(#2204),#40,.T.);
#13322=ADVANCED_FACE('',(#2205),#12747,.T.);
#13323=ADVANCED_FACE('',(#2206),#41,.T.);
#13324=ADVANCED_FACE('',(#2207),#1598,.T.);
#13325=ADVANCED_FACE('',(#2208),#42,.T.);
#13326=ADVANCED_FACE('',(#2209),#12748,.T.);
#13327=ADVANCED_FACE('',(#2210),#43,.T.);
#13328=ADVANCED_FACE('',(#2211),#1599,.T.);
#13329=ADVANCED_FACE('',(#2212),#44,.T.);
#13330=ADVANCED_FACE('',(#2213),#12749,.T.);
#13331=ADVANCED_FACE('',(#2214),#45,.T.);
#13332=ADVANCED_FACE('',(#2215),#1600,.T.);
#13333=ADVANCED_FACE('',(#2216),#46,.T.);
#13334=ADVANCED_FACE('',(#2217),#12750,.T.);
#13335=ADVANCED_FACE('',(#2218),#47,.T.);
#13336=ADVANCED_FACE('',(#2219),#1601,.T.);
#13337=ADVANCED_FACE('',(#2220),#48,.T.);
#13338=ADVANCED_FACE('',(#2221),#12751,.T.);
#13339=ADVANCED_FACE('',(#2222),#49,.T.);
#13340=ADVANCED_FACE('',(#2223),#1602,.T.);
#13341=ADVANCED_FACE('',(#2224),#50,.T.);
#13342=ADVANCED_FACE('',(#2225,#1310),#1603,.T.);
#13343=ADVANCED_FACE('',(#2226),#12752,.T.);
#13633=CLOSED_SHELL('',(#13256,#13257,#13258,#13259,#13260,#13261,#13262,
#13263,#13264,#13265,#13266,#13267,#13268,#13269,#13270,#13271,#13272,#13273,
#13274,#13275,#13276,#13277,#13278,#13279,#13280,#13281,#13282,#13283,#13284,
#13285,#13286,#13287,#13288,#13289,#13290,#13291,#13292,#13293,#13294,#13295,
#13296,#13297,#13298,#13299,#13300,#13301,#13302,#13303,#13304,#13305,#13306,
#13307,#13308,#13309,#13310,#13311,#13312,#13313,#13314,#13315,#13316,#13317,
#13318,#13319,#13320,#13321,#13322,#13323,#13324,#13325,#13326,#13327,#13328,
#13329,#13330,#13331,#13332,#13333,#13334,#13335,#13336,#13337,#13338,#13339,
#13340,#13341,#13342,#13343));
#15128=AXIS2_PLACEMENT_3D('',#22223,#17953,#17954);
#15129=AXIS2_PLACEMENT_3D('',#22224,#17955,#17956);
#15130=AXIS2_PLACEMENT_3D('',#22233,#17961,#17962);
#15131=AXIS2_PLACEMENT_3D('',#22239,#17966,#17967);
#15132=AXIS2_PLACEMENT_3D('',#22245,#17971,#17972);
#15133=AXIS2_PLACEMENT_3D('',#22248,#17973,#17974);
#15134=AXIS2_PLACEMENT_3D('',#22394,#17976,#17977);
#15135=AXIS2_PLACEMENT_3D('',#22540,#17979,#17980);
#15136=AXIS2_PLACEMENT_3D('',#22686,#17982,#17983);
#15137=AXIS2_PLACEMENT_3D('',#22832,#17985,#17986);
#15138=AXIS2_PLACEMENT_3D('',#22978,#17988,#17989);
#15139=AXIS2_PLACEMENT_3D('',#23124,#17991,#17992);
#15140=AXIS2_PLACEMENT_3D('',#23270,#17994,#17995);
#15141=AXIS2_PLACEMENT_3D('',#23416,#17997,#17998);
#15142=AXIS2_PLACEMENT_3D('',#23562,#18000,#18001);
#15143=AXIS2_PLACEMENT_3D('',#23708,#18003,#18004);
#15144=AXIS2_PLACEMENT_3D('',#23854,#18006,#18007);
#15145=AXIS2_PLACEMENT_3D('',#24000,#18009,#18010);
#15146=AXIS2_PLACEMENT_3D('',#24146,#18012,#18013);
#15147=AXIS2_PLACEMENT_3D('',#24292,#18015,#18016);
#15148=AXIS2_PLACEMENT_3D('',#24438,#18018,#18019);
#15149=AXIS2_PLACEMENT_3D('',#24584,#18021,#18022);
#15150=AXIS2_PLACEMENT_3D('',#24730,#18024,#18025);
#15151=AXIS2_PLACEMENT_3D('',#24876,#18027,#18028);
#15152=AXIS2_PLACEMENT_3D('',#25022,#18030,#18031);
#15153=AXIS2_PLACEMENT_3D('',#25166,#18033,#18034);
#15154=AXIS2_PLACEMENT_3D('',#25167,#18035,#18036);
#15155=AXIS2_PLACEMENT_3D('',#25168,#18037,#18038);
#15156=AXIS2_PLACEMENT_3D('',#25169,#18039,#18040);
#15157=AXIS2_PLACEMENT_3D('',#25171,#18041,#18042);
#15158=AXIS2_PLACEMENT_3D('',#25174,#18044,#18045);
#15159=AXIS2_PLACEMENT_3D('',#25175,#18046,#18047);
#15160=AXIS2_PLACEMENT_3D('',#25390,#18050,#18051);
#15161=AXIS2_PLACEMENT_3D('',#25606,#18055,#18056);
#15162=AXIS2_PLACEMENT_3D('',#25608,#18057,#18058);
#15163=AXIS2_PLACEMENT_3D('',#25822,#18061,#18062);
#15164=AXIS2_PLACEMENT_3D('',#26038,#18066,#18067);
#15165=AXIS2_PLACEMENT_3D('',#26040,#18068,#18069);
#15166=AXIS2_PLACEMENT_3D('',#26254,#18072,#18073);
#15167=AXIS2_PLACEMENT_3D('',#26470,#18077,#18078);
#15168=AXIS2_PLACEMENT_3D('',#26472,#18079,#18080);
#15169=AXIS2_PLACEMENT_3D('',#26686,#18083,#18084);
#15170=AXIS2_PLACEMENT_3D('',#26902,#18088,#18089);
#15171=AXIS2_PLACEMENT_3D('',#26904,#18090,#18091);
#15172=AXIS2_PLACEMENT_3D('',#27118,#18094,#18095);
#15173=AXIS2_PLACEMENT_3D('',#27334,#18099,#18100);
#15174=AXIS2_PLACEMENT_3D('',#27336,#18101,#18102);
#15175=AXIS2_PLACEMENT_3D('',#27550,#18105,#18106);
#15176=AXIS2_PLACEMENT_3D('',#27766,#18110,#18111);
#15177=AXIS2_PLACEMENT_3D('',#27768,#18112,#18113);
#15178=AXIS2_PLACEMENT_3D('',#27982,#18116,#18117);
#15179=AXIS2_PLACEMENT_3D('',#28198,#18121,#18122);
#15180=AXIS2_PLACEMENT_3D('',#28200,#18123,#18124);
#15181=AXIS2_PLACEMENT_3D('',#28414,#18127,#18128);
#15182=AXIS2_PLACEMENT_3D('',#28630,#18132,#18133);
#15183=AXIS2_PLACEMENT_3D('',#28632,#18134,#18135);
#15184=AXIS2_PLACEMENT_3D('',#28846,#18138,#18139);
#15185=AXIS2_PLACEMENT_3D('',#29062,#18143,#18144);
#15186=AXIS2_PLACEMENT_3D('',#29064,#18145,#18146);
#15187=AXIS2_PLACEMENT_3D('',#29278,#18149,#18150);
#15188=AXIS2_PLACEMENT_3D('',#29494,#18154,#18155);
#15189=AXIS2_PLACEMENT_3D('',#29496,#18156,#18157);
#15190=AXIS2_PLACEMENT_3D('',#29710,#18160,#18161);
#15191=AXIS2_PLACEMENT_3D('',#29926,#18165,#18166);
#15192=AXIS2_PLACEMENT_3D('',#29928,#18167,#18168);
#15193=AXIS2_PLACEMENT_3D('',#30142,#18171,#18172);
#15194=AXIS2_PLACEMENT_3D('',#30358,#18176,#18177);
#15195=AXIS2_PLACEMENT_3D('',#30360,#18178,#18179);
#15196=AXIS2_PLACEMENT_3D('',#30574,#18182,#18183);
#15197=AXIS2_PLACEMENT_3D('',#30790,#18187,#18188);
#15198=AXIS2_PLACEMENT_3D('',#30792,#18189,#18190);
#15199=AXIS2_PLACEMENT_3D('',#31006,#18193,#18194);
#15200=AXIS2_PLACEMENT_3D('',#31222,#18198,#18199);
#15201=AXIS2_PLACEMENT_3D('',#31224,#18200,#18201);
#15202=AXIS2_PLACEMENT_3D('',#31438,#18204,#18205);
#15203=AXIS2_PLACEMENT_3D('',#31654,#18209,#18210);
#15204=AXIS2_PLACEMENT_3D('',#31656,#18211,#18212);
#15205=AXIS2_PLACEMENT_3D('',#31870,#18215,#18216);
#15206=AXIS2_PLACEMENT_3D('',#32086,#18220,#18221);
#15207=AXIS2_PLACEMENT_3D('',#32088,#18222,#18223);
#15208=AXIS2_PLACEMENT_3D('',#32302,#18226,#18227);
#15209=AXIS2_PLACEMENT_3D('',#32518,#18231,#18232);
#15210=AXIS2_PLACEMENT_3D('',#32520,#18233,#18234);
#15211=AXIS2_PLACEMENT_3D('',#32734,#18237,#18238);
#15212=AXIS2_PLACEMENT_3D('',#32950,#18242,#18243);
#15213=AXIS2_PLACEMENT_3D('',#32952,#18244,#18245);
#15214=AXIS2_PLACEMENT_3D('',#33166,#18248,#18249);
#15215=AXIS2_PLACEMENT_3D('',#33382,#18253,#18254);
#15216=AXIS2_PLACEMENT_3D('',#33384,#18255,#18256);
#15217=AXIS2_PLACEMENT_3D('',#33598,#18259,#18260);
#15218=AXIS2_PLACEMENT_3D('',#33814,#18264,#18265);
#15219=AXIS2_PLACEMENT_3D('',#33815,#18266,#18267);
#15220=AXIS2_PLACEMENT_3D('',#33816,#18268,#18269);
#17953=DIRECTION('axis',(0.,0.,1.));
#17954=DIRECTION('refdir',(1.,0.,0.));
#17955=DIRECTION('center_axis',(1.,0.,0.));
#17956=DIRECTION('ref_axis',(0.,0.,-1.));
#17957=DIRECTION('',(0.,0.,1.));
#17958=DIRECTION('',(0.,1.,0.));
#17959=DIRECTION('',(0.,0.,-1.));
#17960=DIRECTION('',(0.,-1.,0.));
#17961=DIRECTION('center_axis',(0.,0.,-1.));
#17962=DIRECTION('ref_axis',(-1.,0.,0.));
#17963=DIRECTION('',(1.,0.,0.));
#17964=DIRECTION('',(0.,-1.,0.));
#17965=DIRECTION('',(-1.,0.,0.));
#17966=DIRECTION('center_axis',(-1.,0.,0.));
#17967=DIRECTION('ref_axis',(0.,0.,1.));
#17968=DIRECTION('',(0.,0.,-1.));
#17969=DIRECTION('',(0.,1.,0.));
#17970=DIRECTION('',(0.,0.,1.));
#17971=DIRECTION('center_axis',(0.,1.,0.));
#17972=DIRECTION('ref_axis',(1.,0.,0.));
#17973=DIRECTION('center_axis',(0.,-1.,0.));
#17974=DIRECTION('ref_axis',(1.,0.,0.));
#17975=DIRECTION('',(-0.587785252292473,0.,0.809016994374947));
#17976=DIRECTION('center_axis',(0.,-1.,0.));
#17977=DIRECTION('ref_axis',(1.,0.,0.));
#17978=DIRECTION('',(-0.809016994374948,0.,0.587785252292473));
#17979=DIRECTION('center_axis',(0.,-1.,0.));
#17980=DIRECTION('ref_axis',(1.,0.,0.));
#17981=DIRECTION('',(-0.951056516295154,0.,0.309016994374947));
#17982=DIRECTION('center_axis',(0.,-1.,0.));
#17983=DIRECTION('ref_axis',(1.,0.,0.));
#17984=DIRECTION('',(-1.,0.,-1.83697019872103E-16));
#17985=DIRECTION('center_axis',(0.,-1.,0.));
#17986=DIRECTION('ref_axis',(1.,0.,0.));
#17987=DIRECTION('',(-0.951056516295154,0.,-0.309016994374948));
#17988=DIRECTION('center_axis',(0.,-1.,0.));
#17989=DIRECTION('ref_axis',(1.,0.,0.));
#17990=DIRECTION('',(-0.809016994374947,0.,-0.587785252292473));
#17991=DIRECTION('center_axis',(0.,-1.,0.));
#17992=DIRECTION('ref_axis',(1.,0.,0.));
#17993=DIRECTION('',(-0.587785252292473,0.,-0.809016994374948));
#17994=DIRECTION('center_axis',(0.,-1.,0.));
#17995=DIRECTION('ref_axis',(1.,0.,0.));
#17996=DIRECTION('',(-0.309016994374947,0.,-0.951056516295154));
#17997=DIRECTION('center_axis',(0.,-1.,0.));
#17998=DIRECTION('ref_axis',(1.,0.,0.));
#17999=DIRECTION('',(1.22464679914735E-16,0.,-1.));
#18000=DIRECTION('center_axis',(0.,-1.,0.));
#18001=DIRECTION('ref_axis',(1.,0.,0.));
#18002=DIRECTION('',(0.309016994374948,0.,-0.951056516295154));
#18003=DIRECTION('center_axis',(0.,-1.,0.));
#18004=DIRECTION('ref_axis',(1.,0.,0.));
#18005=DIRECTION('',(0.587785252292473,0.,-0.809016994374947));
#18006=DIRECTION('center_axis',(0.,-1.,0.));
#18007=DIRECTION('ref_axis',(1.,0.,0.));
#18008=DIRECTION('',(0.809016994374948,0.,-0.587785252292473));
#18009=DIRECTION('center_axis',(0.,-1.,0.));
#18010=DIRECTION('ref_axis',(1.,0.,0.));
#18011=DIRECTION('',(0.951056516295154,0.,-0.309016994374947));
#18012=DIRECTION('center_axis',(0.,-1.,0.));
#18013=DIRECTION('ref_axis',(1.,0.,0.));
#18014=DIRECTION('',(1.,0.,6.12323399573677E-17));
#18015=DIRECTION('center_axis',(0.,-1.,0.));
#18016=DIRECTION('ref_axis',(1.,0.,0.));
#18017=DIRECTION('',(0.951056516295154,0.,0.309016994374948));
#18018=DIRECTION('center_axis',(0.,-1.,0.));
#18019=DIRECTION('ref_axis',(1.,0.,0.));
#18020=DIRECTION('',(0.809016994374947,0.,0.587785252292473));
#18021=DIRECTION('center_axis',(0.,-1.,0.));
#18022=DIRECTION('ref_axis',(1.,0.,0.));
#18023=DIRECTION('',(0.587785252292473,0.,0.809016994374947));
#18024=DIRECTION('center_axis',(0.,-1.,0.));
#18025=DIRECTION('ref_axis',(1.,0.,0.));
#18026=DIRECTION('',(0.309016994374947,0.,0.951056516295154));
#18027=DIRECTION('center_axis',(0.,-1.,0.));
#18028=DIRECTION('ref_axis',(1.,0.,0.));
#18029=DIRECTION('',(0.,0.,1.));
#18030=DIRECTION('center_axis',(0.,-1.,0.));
#18031=DIRECTION('ref_axis',(1.,0.,0.));
#18032=DIRECTION('',(-0.309016994374948,0.,0.951056516295154));
#18033=DIRECTION('center_axis',(0.,1.,0.));
#18034=DIRECTION('ref_axis',(1.,0.,0.));
#18035=DIRECTION('center_axis',(0.,1.,0.));
#18036=DIRECTION('ref_axis',(6.12323399573677E-17,0.,1.));
#18037=DIRECTION('center_axis',(0.,-1.,0.));
#18038=DIRECTION('ref_axis',(1.,0.,0.));
#18039=DIRECTION('center_axis',(0.,1.,0.));
#18040=DIRECTION('ref_axis',(1.,0.,0.));
#18041=DIRECTION('center_axis',(0.,1.,0.));
#18042=DIRECTION('ref_axis',(1.,0.,0.));
#18043=DIRECTION('',(0.,-1.,0.));
#18044=DIRECTION('center_axis',(0.,-1.,0.));
#18045=DIRECTION('ref_axis',(1.,0.,0.));
#18046=DIRECTION('center_axis',(0.,1.,0.));
#18047=DIRECTION('ref_axis',(1.,0.,0.));
#18048=DIRECTION('',(0.,-1.,0.));
#18049=DIRECTION('',(0.,1.,0.));
#18050=DIRECTION('center_axis',(0.951056516295154,0.,0.309016994374948));
#18051=DIRECTION('ref_axis',(0.309016994374948,0.,-0.951056516295154));
#18052=DIRECTION('',(0.309016994374948,0.,-0.951056516295154));
#18053=DIRECTION('',(0.,1.,0.));
#18054=DIRECTION('',(0.,1.,0.));
#18055=DIRECTION('center_axis',(0.,1.,0.));
#18056=DIRECTION('ref_axis',(1.,0.,0.));
#18057=DIRECTION('center_axis',(0.,1.,0.));
#18058=DIRECTION('ref_axis',(1.,0.,0.));
#18059=DIRECTION('',(0.,-1.,0.));
#18060=DIRECTION('',(0.,1.,0.));
#18061=DIRECTION('center_axis',(0.809016994374947,0.,0.587785252292473));
#18062=DIRECTION('ref_axis',(0.587785252292473,0.,-0.809016994374947));
#18063=DIRECTION('',(0.587785252292473,0.,-0.809016994374947));
#18064=DIRECTION('',(0.,1.,0.));
#18065=DIRECTION('',(0.,1.,0.));
#18066=DIRECTION('center_axis',(0.,1.,0.));
#18067=DIRECTION('ref_axis',(1.,0.,0.));
#18068=DIRECTION('center_axis',(0.,1.,0.));
#18069=DIRECTION('ref_axis',(1.,0.,0.));
#18070=DIRECTION('',(0.,-1.,0.));
#18071=DIRECTION('',(0.,1.,0.));
#18072=DIRECTION('center_axis',(0.587785252292473,0.,0.809016994374948));
#18073=DIRECTION('ref_axis',(0.809016994374948,0.,-0.587785252292473));
#18074=DIRECTION('',(0.809016994374948,0.,-0.587785252292473));
#18075=DIRECTION('',(0.,1.,0.));
#18076=DIRECTION('',(0.,1.,0.));
#18077=DIRECTION('center_axis',(0.,1.,0.));
#18078=DIRECTION('ref_axis',(1.,0.,0.));
#18079=DIRECTION('center_axis',(0.,1.,0.));
#18080=DIRECTION('ref_axis',(1.,0.,0.));
#18081=DIRECTION('',(0.,-1.,0.));
#18082=DIRECTION('',(0.,1.,0.));
#18083=DIRECTION('center_axis',(0.309016994374947,0.,0.951056516295154));
#18084=DIRECTION('ref_axis',(0.951056516295154,0.,-0.309016994374947));
#18085=DIRECTION('',(0.951056516295154,0.,-0.309016994374947));
#18086=DIRECTION('',(0.,1.,0.));
#18087=DIRECTION('',(0.,1.,0.));
#18088=DIRECTION('center_axis',(0.,1.,0.));
#18089=DIRECTION('ref_axis',(1.,0.,0.));
#18090=DIRECTION('center_axis',(0.,1.,0.));
#18091=DIRECTION('ref_axis',(1.,0.,0.));
#18092=DIRECTION('',(0.,-1.,0.));
#18093=DIRECTION('',(0.,1.,0.));
#18094=DIRECTION('center_axis',(-1.83697019872103E-16,0.,1.));
#18095=DIRECTION('ref_axis',(1.,0.,1.83697019872103E-16));
#18096=DIRECTION('',(1.,0.,1.83697019872103E-16));
#18097=DIRECTION('',(0.,1.,0.));
#18098=DIRECTION('',(0.,1.,0.));
#18099=DIRECTION('center_axis',(0.,1.,0.));
#18100=DIRECTION('ref_axis',(1.,0.,0.));
#18101=DIRECTION('center_axis',(0.,1.,0.));
#18102=DIRECTION('ref_axis',(1.,0.,0.));
#18103=DIRECTION('',(0.,-1.,0.));
#18104=DIRECTION('',(0.,1.,0.));
#18105=DIRECTION('center_axis',(-0.309016994374948,0.,0.951056516295154));
#18106=DIRECTION('ref_axis',(0.951056516295154,0.,0.309016994374948));
#18107=DIRECTION('',(0.951056516295154,0.,0.309016994374948));
#18108=DIRECTION('',(0.,1.,0.));
#18109=DIRECTION('',(0.,1.,0.));
#18110=DIRECTION('center_axis',(0.,1.,0.));
#18111=DIRECTION('ref_axis',(1.,0.,0.));
#18112=DIRECTION('center_axis',(0.,1.,0.));
#18113=DIRECTION('ref_axis',(1.,0.,0.));
#18114=DIRECTION('',(0.,-1.,0.));
#18115=DIRECTION('',(0.,1.,0.));
#18116=DIRECTION('center_axis',(-0.587785252292473,0.,0.809016994374947));
#18117=DIRECTION('ref_axis',(0.809016994374947,0.,0.587785252292473));
#18118=DIRECTION('',(0.809016994374947,0.,0.587785252292473));
#18119=DIRECTION('',(0.,1.,0.));
#18120=DIRECTION('',(0.,1.,0.));
#18121=DIRECTION('center_axis',(0.,1.,0.));
#18122=DIRECTION('ref_axis',(1.,0.,0.));
#18123=DIRECTION('center_axis',(0.,1.,0.));
#18124=DIRECTION('ref_axis',(1.,0.,0.));
#18125=DIRECTION('',(0.,-1.,0.));
#18126=DIRECTION('',(0.,1.,0.));
#18127=DIRECTION('center_axis',(-0.809016994374948,0.,0.587785252292473));
#18128=DIRECTION('ref_axis',(0.587785252292473,0.,0.809016994374948));
#18129=DIRECTION('',(0.587785252292473,0.,0.809016994374948));
#18130=DIRECTION('',(0.,1.,0.));
#18131=DIRECTION('',(0.,1.,0.));
#18132=DIRECTION('center_axis',(0.,1.,0.));
#18133=DIRECTION('ref_axis',(1.,0.,0.));
#18134=DIRECTION('center_axis',(0.,1.,0.));
#18135=DIRECTION('ref_axis',(1.,0.,0.));
#18136=DIRECTION('',(0.,-1.,0.));
#18137=DIRECTION('',(0.,1.,0.));
#18138=DIRECTION('center_axis',(-0.951056516295154,0.,0.309016994374947));
#18139=DIRECTION('ref_axis',(0.309016994374947,0.,0.951056516295154));
#18140=DIRECTION('',(0.309016994374947,0.,0.951056516295154));
#18141=DIRECTION('',(0.,1.,0.));
#18142=DIRECTION('',(0.,1.,0.));
#18143=DIRECTION('center_axis',(0.,1.,0.));
#18144=DIRECTION('ref_axis',(1.,0.,0.));
#18145=DIRECTION('center_axis',(0.,1.,0.));
#18146=DIRECTION('ref_axis',(1.,0.,0.));
#18147=DIRECTION('',(0.,-1.,0.));
#18148=DIRECTION('',(0.,1.,0.));
#18149=DIRECTION('center_axis',(-1.,0.,-1.22464679914735E-16));
#18150=DIRECTION('ref_axis',(-1.22464679914735E-16,0.,1.));
#18151=DIRECTION('',(-1.22464679914735E-16,0.,1.));
#18152=DIRECTION('',(0.,1.,0.));
#18153=DIRECTION('',(0.,1.,0.));
#18154=DIRECTION('center_axis',(0.,1.,0.));
#18155=DIRECTION('ref_axis',(1.,0.,0.));
#18156=DIRECTION('center_axis',(0.,1.,0.));
#18157=DIRECTION('ref_axis',(1.,0.,0.));
#18158=DIRECTION('',(0.,-1.,0.));
#18159=DIRECTION('',(0.,1.,0.));
#18160=DIRECTION('center_axis',(-0.951056516295154,0.,-0.309016994374948));
#18161=DIRECTION('ref_axis',(-0.309016994374948,0.,0.951056516295154));
#18162=DIRECTION('',(-0.309016994374948,0.,0.951056516295154));
#18163=DIRECTION('',(0.,1.,0.));
#18164=DIRECTION('',(0.,1.,0.));
#18165=DIRECTION('center_axis',(0.,1.,0.));
#18166=DIRECTION('ref_axis',(1.,0.,0.));
#18167=DIRECTION('center_axis',(0.,1.,0.));
#18168=DIRECTION('ref_axis',(1.,0.,0.));
#18169=DIRECTION('',(0.,-1.,0.));
#18170=DIRECTION('',(0.,1.,0.));
#18171=DIRECTION('center_axis',(-0.809016994374947,0.,-0.587785252292473));
#18172=DIRECTION('ref_axis',(-0.587785252292473,0.,0.809016994374947));
#18173=DIRECTION('',(-0.587785252292473,0.,0.809016994374947));
#18174=DIRECTION('',(0.,1.,0.));
#18175=DIRECTION('',(0.,1.,0.));
#18176=DIRECTION('center_axis',(0.,1.,0.));
#18177=DIRECTION('ref_axis',(1.,0.,0.));
#18178=DIRECTION('center_axis',(0.,1.,0.));
#18179=DIRECTION('ref_axis',(1.,0.,0.));
#18180=DIRECTION('',(0.,-1.,0.));
#18181=DIRECTION('',(0.,1.,0.));
#18182=DIRECTION('center_axis',(-0.587785252292473,0.,-0.809016994374948));
#18183=DIRECTION('ref_axis',(-0.809016994374948,0.,0.587785252292473));
#18184=DIRECTION('',(-0.809016994374948,0.,0.587785252292473));
#18185=DIRECTION('',(0.,1.,0.));
#18186=DIRECTION('',(0.,1.,0.));
#18187=DIRECTION('center_axis',(0.,1.,0.));
#18188=DIRECTION('ref_axis',(1.,0.,0.));
#18189=DIRECTION('center_axis',(0.,1.,0.));
#18190=DIRECTION('ref_axis',(1.,0.,0.));
#18191=DIRECTION('',(0.,-1.,0.));
#18192=DIRECTION('',(0.,1.,0.));
#18193=DIRECTION('center_axis',(-0.309016994374947,0.,-0.951056516295154));
#18194=DIRECTION('ref_axis',(-0.951056516295154,0.,0.309016994374947));
#18195=DIRECTION('',(-0.951056516295154,0.,0.309016994374947));
#18196=DIRECTION('',(0.,1.,0.));
#18197=DIRECTION('',(0.,1.,0.));
#18198=DIRECTION('center_axis',(0.,1.,0.));
#18199=DIRECTION('ref_axis',(1.,0.,0.));
#18200=DIRECTION('center_axis',(0.,1.,0.));
#18201=DIRECTION('ref_axis',(1.,0.,0.));
#18202=DIRECTION('',(0.,-1.,0.));
#18203=DIRECTION('',(0.,1.,0.));
#18204=DIRECTION('center_axis',(6.12323399573677E-17,0.,-1.));
#18205=DIRECTION('ref_axis',(-1.,0.,-6.12323399573677E-17));
#18206=DIRECTION('',(-1.,0.,-6.12323399573677E-17));
#18207=DIRECTION('',(0.,1.,0.));
#18208=DIRECTION('',(0.,1.,0.));
#18209=DIRECTION('center_axis',(0.,1.,0.));
#18210=DIRECTION('ref_axis',(1.,0.,0.));
#18211=DIRECTION('center_axis',(0.,1.,0.));
#18212=DIRECTION('ref_axis',(1.,0.,0.));
#18213=DIRECTION('',(0.,-1.,0.));
#18214=DIRECTION('',(0.,1.,0.));
#18215=DIRECTION('center_axis',(0.309016994374948,0.,-0.951056516295154));
#18216=DIRECTION('ref_axis',(-0.951056516295154,0.,-0.309016994374948));
#18217=DIRECTION('',(-0.951056516295154,0.,-0.309016994374948));
#18218=DIRECTION('',(0.,1.,0.));
#18219=DIRECTION('',(0.,1.,0.));
#18220=DIRECTION('center_axis',(0.,1.,0.));
#18221=DIRECTION('ref_axis',(1.,0.,0.));
#18222=DIRECTION('center_axis',(0.,1.,0.));
#18223=DIRECTION('ref_axis',(1.,0.,0.));
#18224=DIRECTION('',(0.,-1.,0.));
#18225=DIRECTION('',(0.,1.,0.));
#18226=DIRECTION('center_axis',(0.587785252292473,0.,-0.809016994374947));
#18227=DIRECTION('ref_axis',(-0.809016994374947,0.,-0.587785252292473));
#18228=DIRECTION('',(-0.809016994374947,0.,-0.587785252292473));
#18229=DIRECTION('',(0.,1.,0.));
#18230=DIRECTION('',(0.,1.,0.));
#18231=DIRECTION('center_axis',(0.,1.,0.));
#18232=DIRECTION('ref_axis',(1.,0.,0.));
#18233=DIRECTION('center_axis',(0.,1.,0.));
#18234=DIRECTION('ref_axis',(1.,0.,0.));
#18235=DIRECTION('',(0.,-1.,0.));
#18236=DIRECTION('',(0.,1.,0.));
#18237=DIRECTION('center_axis',(0.809016994374947,0.,-0.587785252292473));
#18238=DIRECTION('ref_axis',(-0.587785252292473,0.,-0.809016994374947));
#18239=DIRECTION('',(-0.587785252292473,0.,-0.809016994374947));
#18240=DIRECTION('',(0.,1.,0.));
#18241=DIRECTION('',(0.,1.,0.));
#18242=DIRECTION('center_axis',(0.,1.,0.));
#18243=DIRECTION('ref_axis',(1.,0.,0.));
#18244=DIRECTION('center_axis',(0.,1.,0.));
#18245=DIRECTION('ref_axis',(1.,0.,0.));
#18246=DIRECTION('',(0.,-1.,0.));
#18247=DIRECTION('',(0.,1.,0.));
#18248=DIRECTION('center_axis',(0.951056516295154,0.,-0.309016994374947));
#18249=DIRECTION('ref_axis',(-0.309016994374947,0.,-0.951056516295154));
#18250=DIRECTION('',(-0.309016994374947,0.,-0.951056516295154));
#18251=DIRECTION('',(0.,1.,0.));
#18252=DIRECTION('',(0.,1.,0.));
#18253=DIRECTION('center_axis',(0.,1.,0.));
#18254=DIRECTION('ref_axis',(1.,0.,0.));
#18255=DIRECTION('center_axis',(0.,1.,0.));
#18256=DIRECTION('ref_axis',(1.,0.,0.));
#18257=DIRECTION('',(0.,-1.,0.));
#18258=DIRECTION('',(0.,1.,0.));
#18259=DIRECTION('center_axis',(1.,0.,0.));
#18260=DIRECTION('ref_axis',(0.,0.,-1.));
#18261=DIRECTION('',(0.,0.,-1.));
#18262=DIRECTION('',(0.,1.,0.));
#18263=DIRECTION('',(0.,1.,0.));
#18264=DIRECTION('center_axis',(0.,1.,0.));
#18265=DIRECTION('ref_axis',(1.,0.,0.));
#18266=DIRECTION('center_axis',(0.,1.,0.));
#18267=DIRECTION('ref_axis',(1.,0.,0.));
#18268=DIRECTION('center_axis',(0.,1.,0.));
#18269=DIRECTION('ref_axis',(1.,0.,0.));
#22223=CARTESIAN_POINT('',(0.,0.,0.));
#22224=CARTESIAN_POINT('Origin',(0.2,0.,0.));
#22225=CARTESIAN_POINT('',(0.2,2.2,-0.78));
#22226=CARTESIAN_POINT('',(0.2,2.2,-0.565685424949238));
#22227=CARTESIAN_POINT('',(0.2,2.2,0.));
#22228=CARTESIAN_POINT('',(0.2,-1.,-0.78));
#22229=CARTESIAN_POINT('',(0.2,0.,-0.78));
#22230=CARTESIAN_POINT('',(0.2,-1.,-0.565685424949238));
#22231=CARTESIAN_POINT('',(0.2,-1.,0.));
#22232=CARTESIAN_POINT('',(0.2,0.,-0.565685424949238));
#22233=CARTESIAN_POINT('Origin',(0.2,0.,-0.78));
#22234=CARTESIAN_POINT('',(-0.2,2.2,-0.78));
#22235=CARTESIAN_POINT('',(0.1,2.2,-0.78));
#22236=CARTESIAN_POINT('',(-0.2,-1.,-0.78));
#22237=CARTESIAN_POINT('',(-0.2,0.,-0.78));
#22238=CARTESIAN_POINT('',(0.1,-1.,-0.78));
#22239=CARTESIAN_POINT('Origin',(-0.2,0.,-0.78));
#22240=CARTESIAN_POINT('',(-0.2,2.2,-0.565685424949238));
#22241=CARTESIAN_POINT('',(-0.2,2.2,-0.39));
#22242=CARTESIAN_POINT('',(-0.2,-1.,-0.565685424949238));
#22243=CARTESIAN_POINT('',(-0.2,0.,-0.565685424949238));
#22244=CARTESIAN_POINT('',(-0.2,-1.,-0.39));
#22245=CARTESIAN_POINT('Origin',(0.,-1.,0.));
#22246=CARTESIAN_POINT('',(1.60662857109684,-1.,0.693717979106306));
#22247=CARTESIAN_POINT('',(1.5055822144029,-1.,0.892032620296856));
#22248=CARTESIAN_POINT('Origin',(0.,-1.,0.));
#22249=CARTESIAN_POINT('',(1.81978687191668,-1.,1.23627494547115));
#22250=CARTESIAN_POINT('Ctrl Pts',(1.5055822144029,-1.,0.892032620296856));
#22251=CARTESIAN_POINT('Ctrl Pts',(1.50980486806688,-1.,0.894452006964544));
#22252=CARTESIAN_POINT('Ctrl Pts',(1.51805569590094,-1.,0.899185047483511));
#22253=CARTESIAN_POINT('Ctrl Pts',(1.52984849887993,-1.,0.905967409625651));
#22254=CARTESIAN_POINT('Ctrl Pts',(1.54440491149498,-1.,0.914375919026456));
#22255=CARTESIAN_POINT('Ctrl Pts',(1.56065988578893,-1.,0.923832188944341));
#22256=CARTESIAN_POINT('Ctrl Pts',(1.57499388382243,-1.,0.932246680108685));
#22257=CARTESIAN_POINT('Ctrl Pts',(1.58744937487176,-1.,0.939646377893399));
#22258=CARTESIAN_POINT('Ctrl Pts',(1.59810042043673,-1.,0.946078063315257));
#22259=CARTESIAN_POINT('Ctrl Pts',(1.60706069896936,-1.,0.951613284356035));
#22260=CARTESIAN_POINT('Ctrl Pts',(1.61449324337085,-1.,0.956354422920671));
#22261=CARTESIAN_POINT('Ctrl Pts',(1.62061638140221,-1.,0.960438326101729));
#22262=CARTESIAN_POINT('Ctrl Pts',(1.62571930670187,-1.,0.964046107040536));
#22263=CARTESIAN_POINT('Ctrl Pts',(1.63013849959461,-1.,0.967387853230345));
#22264=CARTESIAN_POINT('Ctrl Pts',(1.63420665729798,-1.,0.970669715997509));
#22265=CARTESIAN_POINT('Ctrl Pts',(1.63820952658144,-1.,0.974066058287419));
#22266=CARTESIAN_POINT('Ctrl Pts',(1.64233990826687,-1.,0.977689794119417));
#22267=CARTESIAN_POINT('Ctrl Pts',(1.64665139190656,-1.,0.981562530939489));
#22268=CARTESIAN_POINT('Ctrl Pts',(1.65110016612638,-1.,0.985642622920821));
#22269=CARTESIAN_POINT('Ctrl Pts',(1.65559044289699,-1.,0.989855627854165));
#22270=CARTESIAN_POINT('Ctrl Pts',(1.66001553809947,-1.,0.994121836661306));
#22271=CARTESIAN_POINT('Ctrl Pts',(1.66430758030376,-1.,0.998389654952758));
#22272=CARTESIAN_POINT('Ctrl Pts',(1.66846059277303,-1.,1.00265091003727));
#22273=CARTESIAN_POINT('Ctrl Pts',(1.67250335383293,-1.,1.00692206696414));
#22274=CARTESIAN_POINT('Ctrl Pts',(1.67648246776464,-1.,1.01123236493511));
#22275=CARTESIAN_POINT('Ctrl Pts',(1.68044289894798,-1.,1.01561026162773));
#22276=CARTESIAN_POINT('Ctrl Pts',(1.68440578021706,-1.,1.02006795074201));
#22277=CARTESIAN_POINT('Ctrl Pts',(1.68836910178447,-1.,1.02460180535255));
#22278=CARTESIAN_POINT('Ctrl Pts',(1.69231840863458,-1.,1.02919977579147));
#22279=CARTESIAN_POINT('Ctrl Pts',(1.69623414782771,-1.,1.03384646003588));
#22280=CARTESIAN_POINT('Ctrl Pts',(1.70010052930962,-1.,1.03852922490789));
#22281=CARTESIAN_POINT('Ctrl Pts',(1.70391338707982,-1.,1.04324363334554));
#22282=CARTESIAN_POINT('Ctrl Pts',(1.70767646263649,-1.,1.04799085404995));
#22283=CARTESIAN_POINT('Ctrl Pts',(1.71139783543989,-1.,1.05277517202855));
#22284=CARTESIAN_POINT('Ctrl Pts',(1.7150865442702,-1.,1.05760163192479));
#22285=CARTESIAN_POINT('Ctrl Pts',(1.71874858456904,-1.,1.06247324680647));
#22286=CARTESIAN_POINT('Ctrl Pts',(1.72238500928453,-1.,1.06738966975462));
#22287=CARTESIAN_POINT('Ctrl Pts',(1.72599406198488,-1.,1.07234866990252));
#22288=CARTESIAN_POINT('Ctrl Pts',(1.72957248977424,-1.,1.0773470373727));
#22289=CARTESIAN_POINT('Ctrl Pts',(1.73311705663407,-1.,1.08238162784749));
#22290=CARTESIAN_POINT('Ctrl Pts',(1.73662628326091,-1.,1.08745056285427));
#22291=CARTESIAN_POINT('Ctrl Pts',(1.74010053962247,-1.,1.09255329056493));
#22292=CARTESIAN_POINT('Ctrl Pts',(1.74354119236208,-1.,1.09768999241226));
#22293=CARTESIAN_POINT('Ctrl Pts',(1.74695004214923,-1.,1.10286118991143));
#22294=CARTESIAN_POINT('Ctrl Pts',(1.7503286607592,-1.,1.10806728183007));
#22295=CARTESIAN_POINT('Ctrl Pts',(1.7536777209463,-1.,1.11330807582551));
#22296=CARTESIAN_POINT('Ctrl Pts',(1.75699720772105,-1.,1.11858293216763));
#22297=CARTESIAN_POINT('Ctrl Pts',(1.76028671825096,-1.,1.12389096855086));
#22298=CARTESIAN_POINT('Ctrl Pts',(1.7635457196617,-1.,1.12923123555075));
#22299=CARTESIAN_POINT('Ctrl Pts',(1.76677384551862,-1.,1.1346029180462));
#22300=CARTESIAN_POINT('Ctrl Pts',(1.76997111386769,-1.,1.14000548336975));
#22301=CARTESIAN_POINT('Ctrl Pts',(1.77313777896194,-1.,1.1454385822692));
#22302=CARTESIAN_POINT('Ctrl Pts',(1.7762742255701,-1.,1.15090197841515));
#22303=CARTESIAN_POINT('Ctrl Pts',(1.77938085564275,-1.,1.15639547194698));
#22304=CARTESIAN_POINT('Ctrl Pts',(1.78245795881009,-1.,1.16191881298499));
#22305=CARTESIAN_POINT('Ctrl Pts',(1.78550566040443,-1.,1.16747166312303));
#22306=CARTESIAN_POINT('Ctrl Pts',(1.78852398877616,-1.,1.17305363177328));
#22307=CARTESIAN_POINT('Ctrl Pts',(1.79151291552689,-1.,1.17866429440809));
#22308=CARTESIAN_POINT('Ctrl Pts',(1.79447240321515,-1.,1.18430321697432));
#22309=CARTESIAN_POINT('Ctrl Pts',(1.79740245923478,-1.,1.18996997934445));
#22310=CARTESIAN_POINT('Ctrl Pts',(1.80030314369879,-1.,1.19566418930242));
#22311=CARTESIAN_POINT('Ctrl Pts',(1.80317454838603,-1.,1.20138548938974));
#22312=CARTESIAN_POINT('Ctrl Pts',(1.80601678480707,-1.,1.20713356605475));
#22313=CARTESIAN_POINT('Ctrl Pts',(1.80882996917129,-1.,1.21290815708314));
#22314=CARTESIAN_POINT('Ctrl Pts',(1.81161420806656,-1.,1.21870906103557));
#22315=CARTESIAN_POINT('Ctrl Pts',(1.81436959210434,-1.,1.2245361330495));
#22316=CARTESIAN_POINT('Ctrl Pts',(1.8165508718364,-1.,1.2292186489137));
#22317=CARTESIAN_POINT('Ctrl Pts',(1.81817389921279,-1.,1.2327422452705));
#22318=CARTESIAN_POINT('Ctrl Pts',(1.81925017193666,-1.,1.23509651170476));
#22319=CARTESIAN_POINT('Ctrl Pts',(1.81978687191668,-1.,1.23627494547115));
#22320=CARTESIAN_POINT('',(1.73811241238545,-1.,1.34869019493419));
#22321=CARTESIAN_POINT('',(1.81978687191668,-1.,1.23627494547115));
#22322=CARTESIAN_POINT('',(1.31362392696032,-1.,1.15624053661742));
#22323=CARTESIAN_POINT('Ctrl Pts',(1.73811241238545,-1.,1.34869019493419));
#22324=CARTESIAN_POINT('Ctrl Pts',(1.73682580585691,-1.,1.34854391898045));
#22325=CARTESIAN_POINT('Ctrl Pts',(1.73425417885907,-1.,1.34824783112887));
#22326=CARTESIAN_POINT('Ctrl Pts',(1.7304014965394,-1.,1.34779309152035));
#22327=CARTESIAN_POINT('Ctrl Pts',(1.72527410680674,-1.,1.34716554819527));
#22328=CARTESIAN_POINT('Ctrl Pts',(1.7188807715049,-1.,1.34634568653227));
#22329=CARTESIAN_POINT('Ctrl Pts',(1.71250340686822,-1.,1.34549029589416));
#22330=CARTESIAN_POINT('Ctrl Pts',(1.70614212266738,-1.,1.34459924533831));
#22331=CARTESIAN_POINT('Ctrl Pts',(1.69979707754427,-1.,1.34367237124483));
#22332=CARTESIAN_POINT('Ctrl Pts',(1.6934684849687,-1.,1.34270948206319));
#22333=CARTESIAN_POINT('Ctrl Pts',(1.68715660868764,-1.,1.341710374848));
#22334=CARTESIAN_POINT('Ctrl Pts',(1.68086176030362,-1.,1.34067485185203));
#22335=CARTESIAN_POINT('Ctrl Pts',(1.67458429426086,-1.,1.3396027347034));
#22336=CARTESIAN_POINT('Ctrl Pts',(1.66832460783989,-1.,1.33849388654388));
#22337=CARTESIAN_POINT('Ctrl Pts',(1.66208312541983,-1.,1.33734820885262));
#22338=CARTESIAN_POINT('Ctrl Pts',(1.65586025952593,-1.,1.33616559745172));
#22339=CARTESIAN_POINT('Ctrl Pts',(1.6496563728683,-1.,1.33494590467993));
#22340=CARTESIAN_POINT('Ctrl Pts',(1.6434717485603,-1.,1.33368890676572));
#22341=CARTESIAN_POINT('Ctrl Pts',(1.63730653475089,-1.,1.33239425103724));
#22342=CARTESIAN_POINT('Ctrl Pts',(1.63116079730923,-1.,1.33106149345645));
#22343=CARTESIAN_POINT('Ctrl Pts',(1.62503464209797,-1.,1.3296901950568));
#22344=CARTESIAN_POINT('Ctrl Pts',(1.61892832270724,-1.,1.32828000610449));
#22345=CARTESIAN_POINT('Ctrl Pts',(1.6128423401575,-1.,1.32683074483356));
#22346=CARTESIAN_POINT('Ctrl Pts',(1.60677758290954,-1.,1.32534250785782));
#22347=CARTESIAN_POINT('Ctrl Pts',(1.60073511858687,-1.,1.32381550858256));
#22348=CARTESIAN_POINT('Ctrl Pts',(1.59471591079403,-1.,1.32224985747682));
#22349=CARTESIAN_POINT('Ctrl Pts',(1.58872057258245,-1.,1.32064537110892));
#22350=CARTESIAN_POINT('Ctrl Pts',(1.58274907898834,-1.,1.31900135021432));
#22351=CARTESIAN_POINT('Ctrl Pts',(1.5768005650559,-1.,1.31731642317187));
#22352=CARTESIAN_POINT('Ctrl Pts',(1.57087397835723,-1.,1.31558903860016));
#22353=CARTESIAN_POINT('Ctrl Pts',(1.56496872402353,-1.,1.31381795281002));
#22354=CARTESIAN_POINT('Ctrl Pts',(1.55908521254821,-1.,1.31200264341696));
#22355=CARTESIAN_POINT('Ctrl Pts',(1.55322568759481,-1.,1.31014393684222));
#22356=CARTESIAN_POINT('Ctrl Pts',(1.54739413957185,-1.,1.30824393907473));
#22357=CARTESIAN_POINT('Ctrl Pts',(1.54159462645432,-1.,1.30630475189556));
#22358=CARTESIAN_POINT('Ctrl Pts',(1.53582981268977,-1.,1.30432735639489));
#22359=CARTESIAN_POINT('Ctrl Pts',(1.53009970283891,-1.,1.30231064395568));
#22360=CARTESIAN_POINT('Ctrl Pts',(1.52439957861062,-1.,1.30024984366328));
#22361=CARTESIAN_POINT('Ctrl Pts',(1.51872184912724,-1.,1.29813791800747));
#22362=CARTESIAN_POINT('Ctrl Pts',(1.51305994241402,-1.,1.29596850710509));
#22363=CARTESIAN_POINT('Ctrl Pts',(1.50741159078365,-1.,1.29373841372842));
#22364=CARTESIAN_POINT('Ctrl Pts',(1.50178230149776,-1.,1.29145022885181));
#22365=CARTESIAN_POINT('Ctrl Pts',(1.49618896881754,-1.,1.28911506584254));
#22366=CARTESIAN_POINT('Ctrl Pts',(1.4906522831278,-1.,1.2867467611644));
#22367=CARTESIAN_POINT('Ctrl Pts',(1.4851881711891,-1.,1.28435533880201));
#22368=CARTESIAN_POINT('Ctrl Pts',(1.47980070347095,-1.,1.28194158939517));
#22369=CARTESIAN_POINT('Ctrl Pts',(1.4744717526707,-1.,1.2794891824849));
#22370=CARTESIAN_POINT('Ctrl Pts',(1.46916035917133,-1.,1.2769641483109));
#22371=CARTESIAN_POINT('Ctrl Pts',(1.46382431332476,-1.,1.27433119897822));
#22372=CARTESIAN_POINT('Ctrl Pts',(1.45843906294697,-1.,1.27156805265289));
#22373=CARTESIAN_POINT('Ctrl Pts',(1.45301422764247,-1.,1.2686778680489));
#22374=CARTESIAN_POINT('Ctrl Pts',(1.44761985001662,-1.,1.26570925118868));
#22375=CARTESIAN_POINT('Ctrl Pts',(1.44236470511303,-1.,1.26273903323859));
#22376=CARTESIAN_POINT('Ctrl Pts',(1.43734919180847,-1.,1.25983531012005));
#22377=CARTESIAN_POINT('Ctrl Pts',(1.43262645609691,-1.,1.25702687965755));
#22378=CARTESIAN_POINT('Ctrl Pts',(1.42815938799387,-1.,1.25426945222639));
#22379=CARTESIAN_POINT('Ctrl Pts',(1.42378102115575,-1.,1.2514145557001));
#22380=CARTESIAN_POINT('Ctrl Pts',(1.41923722596025,-1.,1.24824430986571));
#22381=CARTESIAN_POINT('Ctrl Pts',(1.41422913175179,-1.,1.24450600513056));
#22382=CARTESIAN_POINT('Ctrl Pts',(1.40845295531283,-1.,1.23994455029534));
#22383=CARTESIAN_POINT('Ctrl Pts',(1.40164708206106,-1.,1.23434087290423));
#22384=CARTESIAN_POINT('Ctrl Pts',(1.39361389568796,-1.,1.22752961899387));
#22385=CARTESIAN_POINT('Ctrl Pts',(1.38420564527715,-1.,1.21938737280852));
#22386=CARTESIAN_POINT('Ctrl Pts',(1.37331915607905,-1.,1.20982812925645));
#22387=CARTESIAN_POINT('Ctrl Pts',(1.36088705043885,-1.,1.1987959077932));
#22388=CARTESIAN_POINT('Ctrl Pts',(1.34687054001093,-1.,1.18625865667441));
#22389=CARTESIAN_POINT('Ctrl Pts',(1.33437539347008,-1.,1.17501305789857));
#22390=CARTESIAN_POINT('Ctrl Pts',(1.32428080721772,-1.,1.16589330093588));
#22391=CARTESIAN_POINT('Ctrl Pts',(1.31722977216397,-1.,1.15950888730809));
#22392=CARTESIAN_POINT('Ctrl Pts',(1.31362392696032,-1.,1.15624053661742));
#22393=CARTESIAN_POINT('',(1.15624053661742,-1.,1.31362392696033));
#22394=CARTESIAN_POINT('Origin',(0.,-1.,0.));
#22395=CARTESIAN_POINT('',(1.34869019493419,-1.,1.73811241238545));
#22396=CARTESIAN_POINT('Ctrl Pts',(1.15624053661742,-1.,1.31362392696033));
#22397=CARTESIAN_POINT('Ctrl Pts',(1.15950888730433,-1.,1.3172297721596));
#22398=CARTESIAN_POINT('Ctrl Pts',(1.16589330092532,-1.,1.32428080720544));
#22399=CARTESIAN_POINT('Ctrl Pts',(1.17501305787994,-1.,1.33437539344842));
#22400=CARTESIAN_POINT('Ctrl Pts',(1.18625865664915,-1.,1.34687053998157));
#22401=CARTESIAN_POINT('Ctrl Pts',(1.1987959077656,-1.,1.36088705040677));
#22402=CARTESIAN_POINT('Ctrl Pts',(1.20982812923113,-1.,1.37331915604962));
#22403=CARTESIAN_POINT('Ctrl Pts',(1.21938737278853,-1.,1.38420564525391));
#22404=CARTESIAN_POINT('Ctrl Pts',(1.22752961898063,-1.,1.39361389567257));
#22405=CARTESIAN_POINT('Ctrl Pts',(1.23434087289768,-1.,1.40164708205345));
#22406=CARTESIAN_POINT('Ctrl Pts',(1.23994455029421,-1.,1.40845295531151));
#22407=CARTESIAN_POINT('Ctrl Pts',(1.24450600513278,-1.,1.41422913175437));
#22408=CARTESIAN_POINT('Ctrl Pts',(1.24824430986911,-1.,1.41923722596421));
#22409=CARTESIAN_POINT('Ctrl Pts',(1.25141455570299,-1.,1.42378102115911));
#22410=CARTESIAN_POINT('Ctrl Pts',(1.25426945222783,-1.,1.42815938799555));
#22411=CARTESIAN_POINT('Ctrl Pts',(1.25702687965744,-1.,1.43262645609679));
#22412=CARTESIAN_POINT('Ctrl Pts',(1.25983531011894,-1.,1.43734919180719));
#22413=CARTESIAN_POINT('Ctrl Pts',(1.26273903323723,-1.,1.44236470511145));
#22414=CARTESIAN_POINT('Ctrl Pts',(1.26570925118767,-1.,1.44761985001544));
#22415=CARTESIAN_POINT('Ctrl Pts',(1.26867786804854,-1.,1.45301422764205));
#22416=CARTESIAN_POINT('Ctrl Pts',(1.27156805265312,-1.,1.45843906294725));
#22417=CARTESIAN_POINT('Ctrl Pts',(1.27433119897877,-1.,1.4638243133254));
#22418=CARTESIAN_POINT('Ctrl Pts',(1.27696414831144,-1.,1.46916035917197));
#22419=CARTESIAN_POINT('Ctrl Pts',(1.27948918248524,-1.,1.4744717526711));
#22420=CARTESIAN_POINT('Ctrl Pts',(1.28194158939522,-1.,1.47980070347102));
#22421=CARTESIAN_POINT('Ctrl Pts',(1.28435533880184,-1.,1.48518817118891));
#22422=CARTESIAN_POINT('Ctrl Pts',(1.28674676116415,-1.,1.4906522831275));
#22423=CARTESIAN_POINT('Ctrl Pts',(1.28911506584232,-1.,1.49618896881729));
#22424=CARTESIAN_POINT('Ctrl Pts',(1.29145022885171,-1.,1.50178230149764));
#22425=CARTESIAN_POINT('Ctrl Pts',(1.29373841372843,-1.,1.50741159078367));
#22426=CARTESIAN_POINT('Ctrl Pts',(1.29596850710518,-1.,1.51305994241412));
#22427=CARTESIAN_POINT('Ctrl Pts',(1.29813791800757,-1.,1.51872184912735));
#22428=CARTESIAN_POINT('Ctrl Pts',(1.30024984366334,-1.,1.5243995786107));
#22429=CARTESIAN_POINT('Ctrl Pts',(1.3023106439557,-1.,1.53009970283893));
#22430=CARTESIAN_POINT('Ctrl Pts',(1.30432735639487,-1.,1.53582981268976));
#22431=CARTESIAN_POINT('Ctrl Pts',(1.30630475189553,-1.,1.54159462645428));
#22432=CARTESIAN_POINT('Ctrl Pts',(1.30824393907471,-1.,1.54739413957183));
#22433=CARTESIAN_POINT('Ctrl Pts',(1.31014393684221,-1.,1.55322568759481));
#22434=CARTESIAN_POINT('Ctrl Pts',(1.31200264341696,-1.,1.55908521254822));
#22435=CARTESIAN_POINT('Ctrl Pts',(1.31381795281002,-1.,1.56496872402352));
#22436=CARTESIAN_POINT('Ctrl Pts',(1.31558903860015,-1.,1.57087397835721));
#22437=CARTESIAN_POINT('Ctrl Pts',(1.31731642317183,-1.,1.57680056505585));
#22438=CARTESIAN_POINT('Ctrl Pts',(1.31900135021428,-1.,1.58274907898829));
#22439=CARTESIAN_POINT('Ctrl Pts',(1.32064537110891,-1.,1.58872057258244));
#22440=CARTESIAN_POINT('Ctrl Pts',(1.32224985747686,-1.,1.59471591079408));
#22441=CARTESIAN_POINT('Ctrl Pts',(1.32381550858266,-1.,1.600735118587));
#22442=CARTESIAN_POINT('Ctrl Pts',(1.32534250785794,-1.,1.6067775829097));
#22443=CARTESIAN_POINT('Ctrl Pts',(1.32683074483365,-1.,1.61284234015762));
#22444=CARTESIAN_POINT('Ctrl Pts',(1.32828000610448,-1.,1.61892832270723));
#22445=CARTESIAN_POINT('Ctrl Pts',(1.32969019505665,-1.,1.62503464209777));
#22446=CARTESIAN_POINT('Ctrl Pts',(1.33106149345618,-1.,1.63116079730887));
#22447=CARTESIAN_POINT('Ctrl Pts',(1.33239425103694,-1.,1.6373065347505));
#22448=CARTESIAN_POINT('Ctrl Pts',(1.33368890676554,-1.,1.64347174856007));
#22449=CARTESIAN_POINT('Ctrl Pts',(1.33494590468003,-1.,1.64965637286843));
#22450=CARTESIAN_POINT('Ctrl Pts',(1.33616559745217,-1.,1.65586025952651));
#22451=CARTESIAN_POINT('Ctrl Pts',(1.33734820885331,-1.,1.66208312542073));
#22452=CARTESIAN_POINT('Ctrl Pts',(1.33849388654458,-1.,1.66832460784078));
#22453=CARTESIAN_POINT('Ctrl Pts',(1.33960273470372,-1.,1.67458429426126));
#22454=CARTESIAN_POINT('Ctrl Pts',(1.3406748518516,-1.,1.68086176030308));
#22455=CARTESIAN_POINT('Ctrl Pts',(1.34171037484673,-1.,1.68715660868602));
#22456=CARTESIAN_POINT('Ctrl Pts',(1.34270948206139,-1.,1.6934684849664));
#22457=CARTESIAN_POINT('Ctrl Pts',(1.34367237124322,-1.,1.69979707754221));
#22458=CARTESIAN_POINT('Ctrl Pts',(1.34459924533783,-1.,1.70614212266676));
#22459=CARTESIAN_POINT('Ctrl Pts',(1.34549029589563,-1.,1.71250340687011));
#22460=CARTESIAN_POINT('Ctrl Pts',(1.34634568653586,-1.,1.7188807715095));
#22461=CARTESIAN_POINT('Ctrl Pts',(1.34716554820013,-1.,1.72527410681298));
#22462=CARTESIAN_POINT('Ctrl Pts',(1.3477930915247,-1.,1.73040149654497));
#22463=CARTESIAN_POINT('Ctrl Pts',(1.34824783113158,-1.,1.73425417886255));
#22464=CARTESIAN_POINT('Ctrl Pts',(1.34854391898145,-1.,1.73682580585819));
#22465=CARTESIAN_POINT('Ctrl Pts',(1.34869019493419,-1.,1.73811241238545));
#22466=CARTESIAN_POINT('',(1.23627494547115,-1.,1.81978687191668));
#22467=CARTESIAN_POINT('',(1.34869019493419,-1.,1.73811241238545));
#22468=CARTESIAN_POINT('',(0.892032620296855,-1.,1.5055822144029));
#22469=CARTESIAN_POINT('Ctrl Pts',(1.23627494547115,-1.,1.81978687191668));
#22470=CARTESIAN_POINT('Ctrl Pts',(1.23509651170384,-1.,1.81925017193531));
#22471=CARTESIAN_POINT('Ctrl Pts',(1.23274224526804,-1.,1.81817389920914));
#22472=CARTESIAN_POINT('Ctrl Pts',(1.22921864890975,-1.,1.81655087183054));
#22473=CARTESIAN_POINT('Ctrl Pts',(1.22453613304507,-1.,1.81436959209778));
#22474=CARTESIAN_POINT('Ctrl Pts',(1.2187090610323,-1.,1.81161420806172));
#22475=CARTESIAN_POINT('Ctrl Pts',(1.2129081570818,-1.,1.80882996916931));
#22476=CARTESIAN_POINT('Ctrl Pts',(1.20713356605519,-1.,1.80601678480772));
#22477=CARTESIAN_POINT('Ctrl Pts',(1.2013854893912,-1.,1.8031745483882));
#22478=CARTESIAN_POINT('Ctrl Pts',(1.19566418930405,-1.,1.80030314370121));
#22479=CARTESIAN_POINT('Ctrl Pts',(1.1899699793456,-1.,1.79740245923649));
#22480=CARTESIAN_POINT('Ctrl Pts',(1.18430321697471,-1.,1.79447240321572));
#22481=CARTESIAN_POINT('Ctrl Pts',(1.17866429440781,-1.,1.79151291552646));
#22482=CARTESIAN_POINT('Ctrl Pts',(1.17305363177265,-1.,1.78852398877523));
#22483=CARTESIAN_POINT('Ctrl Pts',(1.16747166312239,-1.,1.78550566040349));
#22484=CARTESIAN_POINT('Ctrl Pts',(1.16191881298458,-1.,1.78245795880949));
#22485=CARTESIAN_POINT('Ctrl Pts',(1.15639547194689,-1.,1.77938085564261));
#22486=CARTESIAN_POINT('Ctrl Pts',(1.15090197841531,-1.,1.77627422557034));
#22487=CARTESIAN_POINT('Ctrl Pts',(1.14543858226948,-1.,1.77313777896234));
#22488=CARTESIAN_POINT('Ctrl Pts',(1.14000548337,-1.,1.76997111386806));
#22489=CARTESIAN_POINT('Ctrl Pts',(1.13460291804634,-1.,1.76677384551883));
#22490=CARTESIAN_POINT('Ctrl Pts',(1.12923123555076,-1.,1.76354571966171));
#22491=CARTESIAN_POINT('Ctrl Pts',(1.12389096855078,-1.,1.76028671825084));
#22492=CARTESIAN_POINT('Ctrl Pts',(1.11858293216752,-1.,1.75699720772089));
#22493=CARTESIAN_POINT('Ctrl Pts',(1.11330807582542,-1.,1.75367772094617));
#22494=CARTESIAN_POINT('Ctrl Pts',(1.10806728183003,-1.,1.75032866075914));
#22495=CARTESIAN_POINT('Ctrl Pts',(1.10286118991144,-1.,1.74695004214924));
#22496=CARTESIAN_POINT('Ctrl Pts',(1.09768999241229,-1.,1.74354119236212));
#22497=CARTESIAN_POINT('Ctrl Pts',(1.09255329056496,-1.,1.74010053962252));
#22498=CARTESIAN_POINT('Ctrl Pts',(1.08745056285429,-1.,1.73662628326093));
#22499=CARTESIAN_POINT('Ctrl Pts',(1.08238162784749,-1.,1.73311705663407));
#22500=CARTESIAN_POINT('Ctrl Pts',(1.0773470373727,-1.,1.72957248977424));
#22501=CARTESIAN_POINT('Ctrl Pts',(1.07234866990252,-1.,1.72599406198489));
#22502=CARTESIAN_POINT('Ctrl Pts',(1.06738966975463,-1.,1.72238500928456));
#22503=CARTESIAN_POINT('Ctrl Pts',(1.06247324680649,-1.,1.71874858456908));
#22504=CARTESIAN_POINT('Ctrl Pts',(1.05760163192481,-1.,1.71508654427022));
#22505=CARTESIAN_POINT('Ctrl Pts',(1.05277517202853,-1.,1.71139783543986));
#22506=CARTESIAN_POINT('Ctrl Pts',(1.0479908540499,-1.,1.70767646263641));
#22507=CARTESIAN_POINT('Ctrl Pts',(1.04324363334546,-1.,1.70391338707969));
#22508=CARTESIAN_POINT('Ctrl Pts',(1.03852922490782,-1.,1.70010052930951));
#22509=CARTESIAN_POINT('Ctrl Pts',(1.03384646003587,-1.,1.69623414782769));
#22510=CARTESIAN_POINT('Ctrl Pts',(1.02919977579155,-1.,1.69231840863471));
#22511=CARTESIAN_POINT('Ctrl Pts',(1.02460180535272,-1.,1.68836910178475));
#22512=CARTESIAN_POINT('Ctrl Pts',(1.02006795074222,-1.,1.68440578021739));
#22513=CARTESIAN_POINT('Ctrl Pts',(1.01561026162786,-1.,1.6804428989482));
#22514=CARTESIAN_POINT('Ctrl Pts',(1.01123236493507,-1.,1.67648246776457));
#22515=CARTESIAN_POINT('Ctrl Pts',(1.00692206696387,-1.,1.67250335383248));
#22516=CARTESIAN_POINT('Ctrl Pts',(1.00265091003682,-1.,1.66846059277231));
#22517=CARTESIAN_POINT('Ctrl Pts',(0.998389654952317,-1.,1.66430758030304));
#22518=CARTESIAN_POINT('Ctrl Pts',(0.994121836661115,-1.,1.66001553809916));
#22519=CARTESIAN_POINT('Ctrl Pts',(0.98985562785445,-1.,1.65559044289746));
#22520=CARTESIAN_POINT('Ctrl Pts',(0.985642622921626,-1.,1.6511001661277));
#22521=CARTESIAN_POINT('Ctrl Pts',(0.981562530940574,-1.,1.64665139190834));
#22522=CARTESIAN_POINT('Ctrl Pts',(0.977689794120296,-1.,1.64233990826831));
#22523=CARTESIAN_POINT('Ctrl Pts',(0.974066058287501,-1.,1.63820952658157));
#22524=CARTESIAN_POINT('Ctrl Pts',(0.970669715996356,-1.,1.63420665729609));
#22525=CARTESIAN_POINT('Ctrl Pts',(0.967387853228041,-1.,1.63013849959083));
#22526=CARTESIAN_POINT('Ctrl Pts',(0.964046107037821,-1.,1.6257193066974));
#22527=CARTESIAN_POINT('Ctrl Pts',(0.960438326099958,-1.,1.62061638139929));
#22528=CARTESIAN_POINT('Ctrl Pts',(0.956354422921572,-1.,1.61449324337233));
#22529=CARTESIAN_POINT('Ctrl Pts',(0.951613284361247,-1.,1.60706069897794));
#22530=CARTESIAN_POINT('Ctrl Pts',(0.946078063325795,-1.,1.59810042045408));
#22531=CARTESIAN_POINT('Ctrl Pts',(0.939646377909319,-1.,1.58744937489796));
#22532=CARTESIAN_POINT('Ctrl Pts',(0.932246680128848,-1.,1.57499388385561));
#22533=CARTESIAN_POINT('Ctrl Pts',(0.923832188966322,-1.,1.56065988582509));
#22534=CARTESIAN_POINT('Ctrl Pts',(0.914375919046579,-1.,1.54440491152808));
#22535=CARTESIAN_POINT('Ctrl Pts',(0.905967409640498,-1.,1.52984849890434));
#22536=CARTESIAN_POINT('Ctrl Pts',(0.89918504749193,-1.,1.51805569591479));
#22537=CARTESIAN_POINT('Ctrl Pts',(0.894452006967538,-1.,1.50980486807181));
#22538=CARTESIAN_POINT('Ctrl Pts',(0.892032620296855,-1.,1.5055822144029));
#22539=CARTESIAN_POINT('',(0.693717979106305,-1.,1.60662857109684));
#22540=CARTESIAN_POINT('Origin',(0.,-1.,0.));
#22541=CARTESIAN_POINT('',(0.7455743247944,-1.,2.0698113262342));
#22542=CARTESIAN_POINT('Ctrl Pts',(0.693717979106305,-1.,1.60662857109684));
#22543=CARTESIAN_POINT('Ctrl Pts',(0.69571209787897,-1.,1.61106790957619));
#22544=CARTESIAN_POINT('Ctrl Pts',(0.699605146398836,-1.,1.61974673471117));
#22545=CARTESIAN_POINT('Ctrl Pts',(0.705159151977294,-1.,1.6321654166204));
#22546=CARTESIAN_POINT('Ctrl Pts',(0.711993139340447,-1.,1.64752408828442));
#22547=CARTESIAN_POINT('Ctrl Pts',(0.719585433787949,-1.,1.66472880551777));
#22548=CARTESIAN_POINT('Ctrl Pts',(0.726235967982445,-1.,1.67996158451922));
#22549=CARTESIAN_POINT('Ctrl Pts',(0.731963238685357,-1.,1.69326921972915));
#22550=CARTESIAN_POINT('Ctrl Pts',(0.736799665716932,-1.,1.70473309004249));
#22551=CARTESIAN_POINT('Ctrl Pts',(0.74079516202821,-1.,1.71447789751001));
#22552=CARTESIAN_POINT('Ctrl Pts',(0.744021445433093,-1.,1.72268229916769));
#22553=CARTESIAN_POINT('Ctrl Pts',(0.746574710097752,-1.,1.72958533647714));
#22554=CARTESIAN_POINT('Ctrl Pts',(0.74858246295687,-1.,1.7355035168033));
#22555=CARTESIAN_POINT('Ctrl Pts',(0.750193435981249,-1.,1.74080458267114));
#22556=CARTESIAN_POINT('Ctrl Pts',(0.751555614164482,-1.,1.74585086852502));
#22557=CARTESIAN_POINT('Ctrl Pts',(0.752797683531314,-1.,1.75095139468794));
#22558=CARTESIAN_POINT('Ctrl Pts',(0.754009254027828,-1.,1.75631083600019));
#22559=CARTESIAN_POINT('Ctrl Pts',(0.755220979974461,-1.,1.76197817240128));
#22560=CARTESIAN_POINT('Ctrl Pts',(0.75642189602781,-1.,1.76789396002998));
#22561=CARTESIAN_POINT('Ctrl Pts',(0.757578264077028,-1.,1.77394167108292));
#22562=CARTESIAN_POINT('Ctrl Pts',(0.758650626677518,-1.,1.77999411220945));
#22563=CARTESIAN_POINT('Ctrl Pts',(0.759614401110189,-1.,1.78596964884604));
#22564=CARTESIAN_POINT('Ctrl Pts',(0.760469555880749,-1.,1.7918581561088));
#22565=CARTESIAN_POINT('Ctrl Pts',(0.761229695230558,-1.,1.79768986997783));
#22566=CARTESIAN_POINT('Ctrl Pts',(0.761915336443547,-1.,1.80351583877342));
#22567=CARTESIAN_POINT('Ctrl Pts',(0.762546129463938,-1.,1.80938551463965));
#22568=CARTESIAN_POINT('Ctrl Pts',(0.763132003836634,-1.,1.8153211840553));
#22569=CARTESIAN_POINT('Ctrl Pts',(0.763673465462726,-1.,1.82131873145266));
#22570=CARTESIAN_POINT('Ctrl Pts',(0.764165902605995,-1.,1.82735991200065));
#22571=CARTESIAN_POINT('Ctrl Pts',(0.764602549687853,-1.,1.83342077227142));
#22572=CARTESIAN_POINT('Ctrl Pts',(0.764978057881737,-1.,1.83948181064835));
#22573=CARTESIAN_POINT('Ctrl Pts',(0.765291664862029,-1.,1.84553698875924));
#22574=CARTESIAN_POINT('Ctrl Pts',(0.765545710619062,-1.,1.85158945130063));
#22575=CARTESIAN_POINT('Ctrl Pts',(0.765744212909318,-1.,1.85764741390394));
#22576=CARTESIAN_POINT('Ctrl Pts',(0.765891519092547,-1.,1.86372027063312));
#22577=CARTESIAN_POINT('Ctrl Pts',(0.765990708546091,-1.,1.86981398314341));
#22578=CARTESIAN_POINT('Ctrl Pts',(0.766042837036744,-1.,1.87592888967883));
#22579=CARTESIAN_POINT('Ctrl Pts',(0.766047794851864,-1.,1.88206215302561));
#22580=CARTESIAN_POINT('Ctrl Pts',(0.766004837062091,-1.,1.88820926433409));
#22581=CARTESIAN_POINT('Ctrl Pts',(0.765913193856978,-1.,1.89436577771388));
#22582=CARTESIAN_POINT('Ctrl Pts',(0.765772772593386,-1.,1.90052930393596));
#22583=CARTESIAN_POINT('Ctrl Pts',(0.765584196937919,-1.,1.90669961402356));
#22584=CARTESIAN_POINT('Ctrl Pts',(0.765348465884722,-1.,1.91287765805169));
#22585=CARTESIAN_POINT('Ctrl Pts',(0.765066729667088,-1.,1.91906491634196));
#22586=CARTESIAN_POINT('Ctrl Pts',(0.764740025488211,-1.,1.92526263537048));
#22587=CARTESIAN_POINT('Ctrl Pts',(0.76436901067394,-1.,1.93147105496382));
#22588=CARTESIAN_POINT('Ctrl Pts',(0.763954049121458,-1.,1.93768964875886));
#22589=CARTESIAN_POINT('Ctrl Pts',(0.763495333538629,-1.,1.9439174661764));
#22590=CARTESIAN_POINT('Ctrl Pts',(0.762992990878769,-1.,1.95015342590024));
#22591=CARTESIAN_POINT('Ctrl Pts',(0.762447203806178,-1.,1.95639665309869));
#22592=CARTESIAN_POINT('Ctrl Pts',(0.761858300014423,-1.,1.96264672744186));
#22593=CARTESIAN_POINT('Ctrl Pts',(0.76122669048382,-1.,1.96890351582499));
#22594=CARTESIAN_POINT('Ctrl Pts',(0.760552825409757,-1.,1.97516705321494));
#22595=CARTESIAN_POINT('Ctrl Pts',(0.75983714745219,-1.,1.98143741418172));
#22596=CARTESIAN_POINT('Ctrl Pts',(0.759080037802488,-1.,1.98771456680874));
#22597=CARTESIAN_POINT('Ctrl Pts',(0.758281796766761,-1.,1.99399831098817));
#22598=CARTESIAN_POINT('Ctrl Pts',(0.757442676862724,-1.,2.00028834739178));
#22599=CARTESIAN_POINT('Ctrl Pts',(0.75656290464667,-1.,2.0065843158773));
#22600=CARTESIAN_POINT('Ctrl Pts',(0.755642704957865,-1.,2.01288584328084));
#22601=CARTESIAN_POINT('Ctrl Pts',(0.754682330722816,-1.,2.01919259405809));
#22602=CARTESIAN_POINT('Ctrl Pts',(0.753682061112768,-1.,2.02550428623313));
#22603=CARTESIAN_POINT('Ctrl Pts',(0.75264218048721,-1.,2.03182068456221));
#22604=CARTESIAN_POINT('Ctrl Pts',(0.751562963361115,-1.,2.03814160092099));
#22605=CARTESIAN_POINT('Ctrl Pts',(0.750444657875575,-1.,2.04446689147979));
#22606=CARTESIAN_POINT('Ctrl Pts',(0.749287468665046,-1.,2.05079645592154));
#22607=CARTESIAN_POINT('Ctrl Pts',(0.748091554183802,-1.,2.05713023031007));
#22608=CARTESIAN_POINT('Ctrl Pts',(0.747103932787919,-1.,2.06220058927826));
#22609=CARTESIAN_POINT('Ctrl Pts',(0.7463458715442,-1.,2.06600523016815));
#22610=CARTESIAN_POINT('Ctrl Pts',(0.745832791378367,-1.,2.06854248895728));
#22611=CARTESIAN_POINT('Ctrl Pts',(0.7455743247944,-1.,2.0698113262342));
#22612=CARTESIAN_POINT('',(0.61342227326009,-1.,2.11275013067528));
#22613=CARTESIAN_POINT('',(0.7455743247944,-1.,2.0698113262342));
#22614=CARTESIAN_POINT('',(0.383122945602004,-1.,1.7075470150345));
#22615=CARTESIAN_POINT('Ctrl Pts',(0.61342227326009,-1.,2.11275013067528));
#22616=CARTESIAN_POINT('Ctrl Pts',(0.6124673655618,-1.,2.11187554259986));
#22617=CARTESIAN_POINT('Ctrl Pts',(0.610560911689898,-1.,2.11012443807238));
#22618=CARTESIAN_POINT('Ctrl Pts',(0.607711315454876,-1.,2.1074919961518));
#22619=CARTESIAN_POINT('Ctrl Pts',(0.60393203073603,-1.,2.10397049886949));
#22620=CARTESIAN_POINT('Ctrl Pts',(0.599241616420533,-1.,2.0995493086477));
#22621=CARTESIAN_POINT('Ctrl Pts',(0.594585006052162,-1.,2.0951087622027));
#22622=CARTESIAN_POINT('Ctrl Pts',(0.589962365403406,-1.,2.09064881812129));
#22623=CARTESIAN_POINT('Ctrl Pts',(0.585373918991617,-1.,2.08616943727951));
#22624=CARTESIAN_POINT('Ctrl Pts',(0.580819952108063,-1.,2.08167059018418));
#22625=CARTESIAN_POINT('Ctrl Pts',(0.576300797416844,-1.,2.07715226767559));
#22626=CARTESIAN_POINT('Ctrl Pts',(0.571816823242602,-1.,2.07261449292824));
#22627=CARTESIAN_POINT('Ctrl Pts',(0.567368421181087,-1.,2.06805732997334));
#22628=CARTESIAN_POINT('Ctrl Pts',(0.562955993082261,-1.,2.06348090160589));
#22629=CARTESIAN_POINT('Ctrl Pts',(0.558579940185151,-1.,2.05888537756462));
#22630=CARTESIAN_POINT('Ctrl Pts',(0.554240657463906,-1.,2.05427091604413));
#22631=CARTESIAN_POINT('Ctrl Pts',(0.549938525150295,-1.,2.04963761077958));
#22632=CARTESIAN_POINT('Ctrl Pts',(0.54567390381743,-1.,2.04498544714588));
#22633=CARTESIAN_POINT('Ctrl Pts',(0.541447120615659,-1.,2.04031422690527));
#22634=CARTESIAN_POINT('Ctrl Pts',(0.537258489833262,-1.,2.03562362954037));
#22635=CARTESIAN_POINT('Ctrl Pts',(0.533108355132976,-1.,2.03091336214426));
#22636=CARTESIAN_POINT('Ctrl Pts',(0.528997127241914,-1.,2.0261832908329));
#22637=CARTESIAN_POINT('Ctrl Pts',(0.524925318333476,-1.,2.02143356304698));
#22638=CARTESIAN_POINT('Ctrl Pts',(0.52089359039937,-1.,2.01666477917286));
#22639=CARTESIAN_POINT('Ctrl Pts',(0.516902681728687,-1.,2.01187773939242));
#22640=CARTESIAN_POINT('Ctrl Pts',(0.512953306961792,-1.,2.00707309946949));
#22641=CARTESIAN_POINT('Ctrl Pts',(0.509046069886157,-1.,2.00225107134734));
#22642=CARTESIAN_POINT('Ctrl Pts',(0.505181361323026,-1.,1.99741107463572));
#22643=CARTESIAN_POINT('Ctrl Pts',(0.501359287727146,-1.,1.99255149126155));
#22644=CARTESIAN_POINT('Ctrl Pts',(0.497579909545574,-1.,1.98767044752932));
#22645=CARTESIAN_POINT('Ctrl Pts',(0.493843476541494,-1.,1.98276658761821));
#22646=CARTESIAN_POINT('Ctrl Pts',(0.490150627860952,-1.,1.97783973019229));
#22647=CARTESIAN_POINT('Ctrl Pts',(0.486502692907658,-1.,1.97289186263272));
#22648=CARTESIAN_POINT('Ctrl Pts',(0.48290166212069,-1.,1.96792703422362));
#22649=CARTESIAN_POINT('Ctrl Pts',(0.479349583074855,-1.,1.96294933055943));
#22650=CARTESIAN_POINT('Ctrl Pts',(0.475848034683176,-1.,1.95796111148177));
#22651=CARTESIAN_POINT('Ctrl Pts',(0.472397672264072,-1.,1.95296148278133));
#22652=CARTESIAN_POINT('Ctrl Pts',(0.468997482913135,-1.,1.94794381136514));
#22653=CARTESIAN_POINT('Ctrl Pts',(0.46564546202603,-1.,1.9428979419619));
#22654=CARTESIAN_POINT('Ctrl Pts',(0.462340031009056,-1.,1.93781486640821));
#22655=CARTESIAN_POINT('Ctrl Pts',(0.459081234547926,-1.,1.93269066517934));
#22656=CARTESIAN_POINT('Ctrl Pts',(0.45587200517437,-1.,1.92753067150476));
#22657=CARTESIAN_POINT('Ctrl Pts',(0.452719478359432,-1.,1.92235380648502));
#22658=CARTESIAN_POINT('Ctrl Pts',(0.449632260106662,-1.,1.91718342555755));
#22659=CARTESIAN_POINT('Ctrl Pts',(0.446617343485711,-1.,1.9120369998112));
#22660=CARTESIAN_POINT('Ctrl Pts',(0.44367755684915,-1.,1.90691756144898));
#22661=CARTESIAN_POINT('Ctrl Pts',(0.440807833704038,-1.,1.90180124389086));
#22662=CARTESIAN_POINT('Ctrl Pts',(0.437995003948244,-1.,1.89663648956466));
#22663=CARTESIAN_POINT('Ctrl Pts',(0.435225660963383,-1.,1.89136993975504));
#22664=CARTESIAN_POINT('Ctrl Pts',(0.432493038548748,-1.,1.88596913666793));
#22665=CARTESIAN_POINT('Ctrl Pts',(0.429803062482344,-1.,1.88044229001832));
#22666=CARTESIAN_POINT('Ctrl Pts',(0.427183828519102,-1.,1.87486989291484));
#22667=CARTESIAN_POINT('Ctrl Pts',(0.424678177291358,-1.,1.86937803944323));
#22668=CARTESIAN_POINT('Ctrl Pts',(0.422327307418275,-1.,1.86408083334028));
#22669=CARTESIAN_POINT('Ctrl Pts',(0.420157287975619,-1.,1.85903281096686));
#22670=CARTESIAN_POINT('Ctrl Pts',(0.418164129143534,-1.,1.85417632856234));
#22671=CARTESIAN_POINT('Ctrl Pts',(0.416300022038864,-1.,1.84929312929882));
#22672=CARTESIAN_POINT('Ctrl Pts',(0.41448743825434,-1.,1.8440575707371));
#22673=CARTESIAN_POINT('Ctrl Pts',(0.412633125322161,-1.,1.83808953475839));
#22674=CARTESIAN_POINT('Ctrl Pts',(0.410641256301674,-1.,1.83100408895216));
#22675=CARTESIAN_POINT('Ctrl Pts',(0.408428948108533,-1.,1.8224702267854));
#22676=CARTESIAN_POINT('Ctrl Pts',(0.405933518411838,-1.,1.81223801813988));
#22677=CARTESIAN_POINT('Ctrl Pts',(0.403107976170441,-1.,1.80012077176221));
#22678=CARTESIAN_POINT('Ctrl Pts',(0.39991940378308,-1.,1.78598826347533));
#22679=CARTESIAN_POINT('Ctrl Pts',(0.39634619612042,-1.,1.7697556004756));
#22680=CARTESIAN_POINT('Ctrl Pts',(0.392375812294307,-1.,1.75137405313962));
#22681=CARTESIAN_POINT('Ctrl Pts',(0.388877023509191,-1.,1.7349317097561));
#22682=CARTESIAN_POINT('Ctrl Pts',(0.38607079032701,-1.,1.72162022246158));
#22683=CARTESIAN_POINT('Ctrl Pts',(0.384119047315541,-1.,1.71231062891958));
#22684=CARTESIAN_POINT('Ctrl Pts',(0.383122945602004,-1.,1.7075470150345));
#22685=CARTESIAN_POINT('',(0.163289472382896,-1.,1.74236521665491));
#22686=CARTESIAN_POINT('Origin',(0.,-1.,0.));
#22687=CARTESIAN_POINT('',(0.0694764450219578,-1.,2.19890268624765));
#22688=CARTESIAN_POINT('Ctrl Pts',(0.163289472382896,-1.,1.74236521665491));
#22689=CARTESIAN_POINT('Ctrl Pts',(0.163814161002002,-1.,1.7472034950333));
#22690=CARTESIAN_POINT('Ctrl Pts',(0.164834765707158,-1.,1.75666056638427));
#22691=CARTESIAN_POINT('Ctrl Pts',(0.1662793551464,-1.,1.77018771684844));
#22692=CARTESIAN_POINT('Ctrl Pts',(0.168032772805197,-1.,1.7869064998507));
#22693=CARTESIAN_POINT('Ctrl Pts',(0.169936923904608,-1.,1.80561530629706));
#22694=CARTESIAN_POINT('Ctrl Pts',(0.171554770204119,-1.,1.82215766811545));
#22695=CARTESIAN_POINT('Ctrl Pts',(0.1728894428919,-1.,1.83658380527692));
#22696=CARTESIAN_POINT('Ctrl Pts',(0.173946627587731,-1.,1.8489811319852));
#22697=CARTESIAN_POINT('Ctrl Pts',(0.17473525927603,-1.,1.85948367088837));
#22698=CARTESIAN_POINT('Ctrl Pts',(0.175268337590757,-1.,1.86828349694799));
#22699=CARTESIAN_POINT('Ctrl Pts',(0.175563480746485,-1.,1.87563767773588));
#22700=CARTESIAN_POINT('Ctrl Pts',(0.175644148889698,-1.,1.88188663145367));
#22701=CARTESIAN_POINT('Ctrl Pts',(0.175538155840648,-1.,1.88742606273259));
#22702=CARTESIAN_POINT('Ctrl Pts',(0.175274276190844,-1.,1.892646301985));
#22703=CARTESIAN_POINT('Ctrl Pts',(0.174879405091263,-1.,1.89788101117132));
#22704=CARTESIAN_POINT('Ctrl Pts',(0.174375518661085,-1.,1.90335253862834));
#22705=CARTESIAN_POINT('Ctrl Pts',(0.173776635257816,-1.,1.90911693975267));
#22706=CARTESIAN_POINT('Ctrl Pts',(0.173090695383496,-1.,1.91511429159527));
#22707=CARTESIAN_POINT('Ctrl Pts',(0.172321621259513,-1.,1.9212233439798));
#22708=CARTESIAN_POINT('Ctrl Pts',(0.171471191532988,-1.,1.92731093582036));
#22709=CARTESIAN_POINT('Ctrl Pts',(0.170541253116201,-1.,1.93329183155539));
#22710=CARTESIAN_POINT('Ctrl Pts',(0.16953490481749,-1.,1.93915639211581));
#22711=CARTESIAN_POINT('Ctrl Pts',(0.168455741607556,-1.,1.94493757756931));
#22712=CARTESIAN_POINT('Ctrl Pts',(0.167307501784475,-1.,1.95069027794294));
#22713=CARTESIAN_POINT('Ctrl Pts',(0.166093592002812,-1.,1.9564675971873));
#22714=CARTESIAN_POINT('Ctrl Pts',(0.164816568920269,-1.,1.96229379940136));
#22715=CARTESIAN_POINT('Ctrl Pts',(0.163478185457734,-1.,1.96816512677967));
#22716=CARTESIAN_POINT('Ctrl Pts',(0.162079693556288,-1.,1.97406280235188));
#22717=CARTESIAN_POINT('Ctrl Pts',(0.160622060784611,-1.,1.97996195437559));
#22718=CARTESIAN_POINT('Ctrl Pts',(0.159106226437299,-1.,1.98584238283292));
#22719=CARTESIAN_POINT('Ctrl Pts',(0.157533331459227,-1.,1.99169810931908));
#22720=CARTESIAN_POINT('Ctrl Pts',(0.155904629548783,-1.,1.99753284771497));
#22721=CARTESIAN_POINT('Ctrl Pts',(0.154221403049722,-1.,2.00335565310543));
#22722=CARTESIAN_POINT('Ctrl Pts',(0.152484883621449,-1.,2.00917680318424));
#22723=CARTESIAN_POINT('Ctrl Pts',(0.150696157673078,-1.,2.01500291940238));
#22724=CARTESIAN_POINT('Ctrl Pts',(0.148856124775337,-1.,2.02083464969894));
#22725=CARTESIAN_POINT('Ctrl Pts',(0.146965557332583,-1.,2.02666926182017));
#22726=CARTESIAN_POINT('Ctrl Pts',(0.145025140186057,-1.,2.03250223739942));
#22727=CARTESIAN_POINT('Ctrl Pts',(0.143035515058208,-1.,2.03832911025912));
#22728=CARTESIAN_POINT('Ctrl Pts',(0.140997332152546,-1.,2.04414757947916));
#22729=CARTESIAN_POINT('Ctrl Pts',(0.138911255368966,-1.,2.04995762001328));
#22730=CARTESIAN_POINT('Ctrl Pts',(0.136777941218043,-1.,2.05576044414264));
#22731=CARTESIAN_POINT('Ctrl Pts',(0.134598026192106,-1.,2.06155781517842));
#22732=CARTESIAN_POINT('Ctrl Pts',(0.13237211154771,-1.,2.06735123910326));
#22733=CARTESIAN_POINT('Ctrl Pts',(0.130100748328403,-1.,2.07314114713063));
#22734=CARTESIAN_POINT('Ctrl Pts',(0.12778444527612,-1.,2.07892715110987));
#22735=CARTESIAN_POINT('Ctrl Pts',(0.125423679412061,-1.,2.08470840653643));
#22736=CARTESIAN_POINT('Ctrl Pts',(0.123018905621083,-1.,2.09048392424825));
#22737=CARTESIAN_POINT('Ctrl Pts',(0.120570567965122,-1.,2.0962529286773));
#22738=CARTESIAN_POINT('Ctrl Pts',(0.118079107988355,-1.,2.102015121329));
#22739=CARTESIAN_POINT('Ctrl Pts',(0.115544957687926,-1.,2.10777050261309));
#22740=CARTESIAN_POINT('Ctrl Pts',(0.112968534419737,-1.,2.11351924490306));
#22741=CARTESIAN_POINT('Ctrl Pts',(0.110350236135025,-1.,2.11926155590865));
#22742=CARTESIAN_POINT('Ctrl Pts',(0.10769043523109,-1.,2.12499752307));
#22743=CARTESIAN_POINT('Ctrl Pts',(0.104989479152739,-1.,2.13072704887293));
#22744=CARTESIAN_POINT('Ctrl Pts',(0.1022477005561,-1.,2.13644992667165));
#22745=CARTESIAN_POINT('Ctrl Pts',(0.0994654261990913,-1.,2.14216588396025));
#22746=CARTESIAN_POINT('Ctrl Pts',(0.0966429852305456,-1.,2.14787463531795));
#22747=CARTESIAN_POINT('Ctrl Pts',(0.0937807218867641,-1.,2.1535759397817));
#22748=CARTESIAN_POINT('Ctrl Pts',(0.0908789888107263,-1.,2.15926961544516));
#22749=CARTESIAN_POINT('Ctrl Pts',(0.087938129138692,-1.,2.16495552645014));
#22750=CARTESIAN_POINT('Ctrl Pts',(0.084958462083537,-1.,2.17063357870952));
#22751=CARTESIAN_POINT('Ctrl Pts',(0.0819402680872763,-1.,2.176303712113));
#22752=CARTESIAN_POINT('Ctrl Pts',(0.078883772768524,-1.,2.18196589448887));
#22753=CARTESIAN_POINT('Ctrl Pts',(0.0757891465836145,-1.,2.1876201139953));
#22754=CARTESIAN_POINT('Ctrl Pts',(0.0732830357306722,-1.,2.19213712013662));
#22755=CARTESIAN_POINT('Ctrl Pts',(0.0713863779526151,-1.,2.19552129484002));
#22756=CARTESIAN_POINT('Ctrl Pts',(0.0701143536325487,-1.,2.19777582085423));
#22757=CARTESIAN_POINT('Ctrl Pts',(0.0694764450219578,-1.,2.19890268624765));
#22758=CARTESIAN_POINT('',(-0.0694764450219586,-1.,2.19890268624765));
#22759=CARTESIAN_POINT('',(0.0694764450219578,-1.,2.19890268624765));
#22760=CARTESIAN_POINT('',(-0.163289472382896,-1.,1.74236521665491));
#22761=CARTESIAN_POINT('Ctrl Pts',(-0.0694764450219586,-1.,2.19890268624765));
#22762=CARTESIAN_POINT('Ctrl Pts',(-0.0701143536324929,-1.,2.19777582085261));
#22763=CARTESIAN_POINT('Ctrl Pts',(-0.071386377952463,-1.,2.19552129483562));
#22764=CARTESIAN_POINT('Ctrl Pts',(-0.0732830357304279,-1.,2.19213712012956));
#22765=CARTESIAN_POINT('Ctrl Pts',(-0.0757891465833414,-1.,2.1876201139874));
#22766=CARTESIAN_POINT('Ctrl Pts',(-0.078883772768323,-1.,2.18196589448304));
#22767=CARTESIAN_POINT('Ctrl Pts',(-0.0819402680871942,-1.,2.1763037121106));
#22768=CARTESIAN_POINT('Ctrl Pts',(-0.0849584620835646,-1.,2.17063357871031));
#22769=CARTESIAN_POINT('Ctrl Pts',(-0.0879381291387825,-1.,2.16495552645275));
#22770=CARTESIAN_POINT('Ctrl Pts',(-0.0908789888108269,-1.,2.15926961544808));
#22771=CARTESIAN_POINT('Ctrl Pts',(-0.0937807218868348,-1.,2.15357593978377));
#22772=CARTESIAN_POINT('Ctrl Pts',(-0.0966429852305691,-1.,2.14787463531864));
#22773=CARTESIAN_POINT('Ctrl Pts',(-0.0994654261990745,-1.,2.14216588395974));
#22774=CARTESIAN_POINT('Ctrl Pts',(-0.102247700556064,-1.,2.13644992667052));
#22775=CARTESIAN_POINT('Ctrl Pts',(-0.104989479152703,-1.,2.1307270488718));
#22776=CARTESIAN_POINT('Ctrl Pts',(-0.107690435231068,-1.,2.12499752306927));
#22777=CARTESIAN_POINT('Ctrl Pts',(-0.11035023613502,-1.,2.11926155590849));
#22778=CARTESIAN_POINT('Ctrl Pts',(-0.112968534419746,-1.,2.11351924490335));
#22779=CARTESIAN_POINT('Ctrl Pts',(-0.115544957687941,-1.,2.10777050261359));
#22780=CARTESIAN_POINT('Ctrl Pts',(-0.118079107988368,-1.,2.10201512132945));
#22781=CARTESIAN_POINT('Ctrl Pts',(-0.120570567965129,-1.,2.09625292867756));
#22782=CARTESIAN_POINT('Ctrl Pts',(-0.123018905621083,-1.,2.09048392424826));
#22783=CARTESIAN_POINT('Ctrl Pts',(-0.125423679412058,-1.,2.08470840653628));
#22784=CARTESIAN_POINT('Ctrl Pts',(-0.127784445276116,-1.,2.07892715110967));
#22785=CARTESIAN_POINT('Ctrl Pts',(-0.130100748328401,-1.,2.07314114713047));
#22786=CARTESIAN_POINT('Ctrl Pts',(-0.13237211154771,-1.,2.06735123910319));
#22787=CARTESIAN_POINT('Ctrl Pts',(-0.134598026192107,-1.,2.06155781517844));
#22788=CARTESIAN_POINT('Ctrl Pts',(-0.136777941218044,-1.,2.0557604441427));
#22789=CARTESIAN_POINT('Ctrl Pts',(-0.138911255368966,-1.,2.04995762001333));
#22790=CARTESIAN_POINT('Ctrl Pts',(-0.140997332152546,-1.,2.04414757947919));
#22791=CARTESIAN_POINT('Ctrl Pts',(-0.143035515058208,-1.,2.03832911025913));
#22792=CARTESIAN_POINT('Ctrl Pts',(-0.145025140186058,-1.,2.03250223739941));
#22793=CARTESIAN_POINT('Ctrl Pts',(-0.146965557332586,-1.,2.02666926182017));
#22794=CARTESIAN_POINT('Ctrl Pts',(-0.148856124775343,-1.,2.02083464969897));
#22795=CARTESIAN_POINT('Ctrl Pts',(-0.150696157673084,-1.,2.01500291940243));
#22796=CARTESIAN_POINT('Ctrl Pts',(-0.152484883621452,-1.,2.00917680318426));
#22797=CARTESIAN_POINT('Ctrl Pts',(-0.154221403049719,-1.,2.00335565310539));
#22798=CARTESIAN_POINT('Ctrl Pts',(-0.155904629548775,-1.,1.99753284771487));
#22799=CARTESIAN_POINT('Ctrl Pts',(-0.157533331459215,-1.,1.99169810931893));
#22800=CARTESIAN_POINT('Ctrl Pts',(-0.159106226437289,-1.,1.98584238283279));
#22801=CARTESIAN_POINT('Ctrl Pts',(-0.16062206078461,-1.,1.97996195437557));
#22802=CARTESIAN_POINT('Ctrl Pts',(-0.162079693556302,-1.,1.97406280235204));
#22803=CARTESIAN_POINT('Ctrl Pts',(-0.16347818545776,-1.,1.96816512678));
#22804=CARTESIAN_POINT('Ctrl Pts',(-0.1648165689203,-1.,1.96229379940174));
#22805=CARTESIAN_POINT('Ctrl Pts',(-0.166093592002833,-1.,1.95646759718755));
#22806=CARTESIAN_POINT('Ctrl Pts',(-0.167307501784469,-1.,1.95069027794286));
#22807=CARTESIAN_POINT('Ctrl Pts',(-0.168455741607516,-1.,1.94493757756879));
#22808=CARTESIAN_POINT('Ctrl Pts',(-0.169534904817425,-1.,1.93915639211497));
#22809=CARTESIAN_POINT('Ctrl Pts',(-0.170541253116136,-1.,1.93329183155455));
#22810=CARTESIAN_POINT('Ctrl Pts',(-0.17147119153296,-1.,1.92731093582));
#22811=CARTESIAN_POINT('Ctrl Pts',(-0.172321621259557,-1.,1.92122334398034));
#22812=CARTESIAN_POINT('Ctrl Pts',(-0.173090695383619,-1.,1.91511429159681));
#22813=CARTESIAN_POINT('Ctrl Pts',(-0.173776635257984,-1.,1.90911693975475));
#22814=CARTESIAN_POINT('Ctrl Pts',(-0.174375518661222,-1.,1.90335253863003));
#22815=CARTESIAN_POINT('Ctrl Pts',(-0.174879405091277,-1.,1.89788101117148));
#22816=CARTESIAN_POINT('Ctrl Pts',(-0.175274276190664,-1.,1.89264630198279));
#22817=CARTESIAN_POINT('Ctrl Pts',(-0.175538155840286,-1.,1.88742606272818));
#22818=CARTESIAN_POINT('Ctrl Pts',(-0.175644148889271,-1.,1.88188663144846));
#22819=CARTESIAN_POINT('Ctrl Pts',(-0.175563480746206,-1.,1.87563767773249));
#22820=CARTESIAN_POINT('Ctrl Pts',(-0.175268337590901,-1.,1.86828349694972));
#22821=CARTESIAN_POINT('Ctrl Pts',(-0.174735259276856,-1.,1.85948367089838));
#22822=CARTESIAN_POINT('Ctrl Pts',(-0.173946627589401,-1.,1.84898113200543));
#22823=CARTESIAN_POINT('Ctrl Pts',(-0.17288944289442,-1.,1.83658380530747));
#22824=CARTESIAN_POINT('Ctrl Pts',(-0.171554770207306,-1.,1.82215766815414));
#22825=CARTESIAN_POINT('Ctrl Pts',(-0.169936923908078,-1.,1.80561530633924));
#22826=CARTESIAN_POINT('Ctrl Pts',(-0.16803277280837,-1.,1.78690649988931));
#22827=CARTESIAN_POINT('Ctrl Pts',(-0.166279355148738,-1.,1.77018771687692));
#22828=CARTESIAN_POINT('Ctrl Pts',(-0.164834765708484,-1.,1.75666056640041));
#22829=CARTESIAN_POINT('Ctrl Pts',(-0.163814161002474,-1.,1.74720349503904));
#22830=CARTESIAN_POINT('Ctrl Pts',(-0.163289472382896,-1.,1.74236521665491));
#22831=CARTESIAN_POINT('',(-0.383122945602004,-1.,1.7075470150345));
#22832=CARTESIAN_POINT('Origin',(0.,-1.,0.));
#22833=CARTESIAN_POINT('',(-0.61342227326009,-1.,2.11275013067528));
#22834=CARTESIAN_POINT('Ctrl Pts',(-0.383122945602004,-1.,1.7075470150345));
#22835=CARTESIAN_POINT('Ctrl Pts',(-0.384119047314215,-1.,1.71231062891398));
#22836=CARTESIAN_POINT('Ctrl Pts',(-0.386070790323281,-1.,1.72162022244582));
#22837=CARTESIAN_POINT('Ctrl Pts',(-0.388877023502615,-1.,1.73493170972829));
#22838=CARTESIAN_POINT('Ctrl Pts',(-0.392375812285395,-1.,1.75137405310193));
#22839=CARTESIAN_POINT('Ctrl Pts',(-0.396346196110688,-1.,1.76975560043442));
#22840=CARTESIAN_POINT('Ctrl Pts',(-0.399919403774155,-1.,1.78598826343754));
#22841=CARTESIAN_POINT('Ctrl Pts',(-0.403107976163396,-1.,1.80012077173238));
#22842=CARTESIAN_POINT('Ctrl Pts',(-0.405933518407175,-1.,1.81223801812013));
#22843=CARTESIAN_POINT('Ctrl Pts',(-0.408428948106227,-1.,1.82247022677562));
#22844=CARTESIAN_POINT('Ctrl Pts',(-0.410641256301276,-1.,1.83100408895047));
#22845=CARTESIAN_POINT('Ctrl Pts',(-0.412633125322945,-1.,1.8380895347617));
#22846=CARTESIAN_POINT('Ctrl Pts',(-0.414487438255542,-1.,1.84405757074218));
#22847=CARTESIAN_POINT('Ctrl Pts',(-0.416300022039885,-1.,1.84929312930314));
#22848=CARTESIAN_POINT('Ctrl Pts',(-0.418164129144045,-1.,1.8541763285645));
#22849=CARTESIAN_POINT('Ctrl Pts',(-0.420157287975583,-1.,1.8590328109667));
#22850=CARTESIAN_POINT('Ctrl Pts',(-0.422327307417885,-1.,1.86408083333863));
#22851=CARTESIAN_POINT('Ctrl Pts',(-0.424678177290876,-1.,1.8693780394412));
#22852=CARTESIAN_POINT('Ctrl Pts',(-0.427183828518743,-1.,1.87486989291333));
#22853=CARTESIAN_POINT('Ctrl Pts',(-0.429803062482217,-1.,1.88044229001778));
#22854=CARTESIAN_POINT('Ctrl Pts',(-0.432493038548833,-1.,1.88596913666828));
#22855=CARTESIAN_POINT('Ctrl Pts',(-0.43522566096358,-1.,1.89136993975585));
#22856=CARTESIAN_POINT('Ctrl Pts',(-0.437995003948443,-1.,1.89663648956549));
#22857=CARTESIAN_POINT('Ctrl Pts',(-0.440807833704161,-1.,1.90180124389137));
#22858=CARTESIAN_POINT('Ctrl Pts',(-0.44367755684917,-1.,1.90691756144906));
#22859=CARTESIAN_POINT('Ctrl Pts',(-0.446617343485651,-1.,1.91203699981095));
#22860=CARTESIAN_POINT('Ctrl Pts',(-0.449632260106572,-1.,1.91718342555717));
#22861=CARTESIAN_POINT('Ctrl Pts',(-0.452719478359356,-1.,1.9223538064847));
#22862=CARTESIAN_POINT('Ctrl Pts',(-0.455872005174335,-1.,1.92753067150461));
#22863=CARTESIAN_POINT('Ctrl Pts',(-0.459081234547931,-1.,1.93269066517936));
#22864=CARTESIAN_POINT('Ctrl Pts',(-0.462340031009087,-1.,1.93781486640834));
#22865=CARTESIAN_POINT('Ctrl Pts',(-0.465645462026065,-1.,1.94289794196205));
#22866=CARTESIAN_POINT('Ctrl Pts',(-0.468997482913158,-1.,1.94794381136524));
#22867=CARTESIAN_POINT('Ctrl Pts',(-0.47239767226408,-1.,1.95296148278136));
#22868=CARTESIAN_POINT('Ctrl Pts',(-0.475848034683172,-1.,1.95796111148175));
#22869=CARTESIAN_POINT('Ctrl Pts',(-0.479349583074846,-1.,1.96294933055938));
#22870=CARTESIAN_POINT('Ctrl Pts',(-0.482901662120687,-1.,1.96792703422358));
#22871=CARTESIAN_POINT('Ctrl Pts',(-0.486502692907661,-1.,1.97289186263272));
#22872=CARTESIAN_POINT('Ctrl Pts',(-0.490150627860955,-1.,1.97783973019229));
#22873=CARTESIAN_POINT('Ctrl Pts',(-0.493843476541492,-1.,1.9827665876182));
#22874=CARTESIAN_POINT('Ctrl Pts',(-0.497579909545564,-1.,1.98767044752929));
#22875=CARTESIAN_POINT('Ctrl Pts',(-0.501359287727129,-1.,1.9925514912615));
#22876=CARTESIAN_POINT('Ctrl Pts',(-0.505181361323011,-1.,1.99741107463567));
#22877=CARTESIAN_POINT('Ctrl Pts',(-0.509046069886152,-1.,2.00225107134733));
#22878=CARTESIAN_POINT('Ctrl Pts',(-0.512953306961814,-1.,2.00707309946955));
#22879=CARTESIAN_POINT('Ctrl Pts',(-0.516902681728733,-1.,2.01187773939257));
#22880=CARTESIAN_POINT('Ctrl Pts',(-0.520893590399428,-1.,2.01666477917305));
#22881=CARTESIAN_POINT('Ctrl Pts',(-0.524925318333518,-1.,2.02143356304712));
#22882=CARTESIAN_POINT('Ctrl Pts',(-0.528997127241911,-1.,2.02618329083289));
#22883=CARTESIAN_POINT('Ctrl Pts',(-0.533108355132905,-1.,2.03091336214401));
#22884=CARTESIAN_POINT('Ctrl Pts',(-0.537258489833134,-1.,2.03562362953993));
#22885=CARTESIAN_POINT('Ctrl Pts',(-0.54144712061552,-1.,2.0403142269048));
#22886=CARTESIAN_POINT('Ctrl Pts',(-0.545673903817348,-1.,2.0449854471456));
#22887=CARTESIAN_POINT('Ctrl Pts',(-0.549938525150342,-1.,2.04963761077974));
#22888=CARTESIAN_POINT('Ctrl Pts',(-0.55424065746411,-1.,2.05427091604482));
#22889=CARTESIAN_POINT('Ctrl Pts',(-0.558579940185467,-1.,2.05888537756571));
#22890=CARTESIAN_POINT('Ctrl Pts',(-0.562955993082574,-1.,2.06348090160697));
#22891=CARTESIAN_POINT('Ctrl Pts',(-0.567368421181229,-1.,2.06805732997383));
#22892=CARTESIAN_POINT('Ctrl Pts',(-0.571816823242411,-1.,2.07261449292757));
#22893=CARTESIAN_POINT('Ctrl Pts',(-0.576300797416275,-1.,2.07715226767361));
#22894=CARTESIAN_POINT('Ctrl Pts',(-0.580819952107257,-1.,2.08167059018138));
#22895=CARTESIAN_POINT('Ctrl Pts',(-0.585373918990895,-1.,2.086169437277));
#22896=CARTESIAN_POINT('Ctrl Pts',(-0.589962365403189,-1.,2.09064881812053));
#22897=CARTESIAN_POINT('Ctrl Pts',(-0.594585006052824,-1.,2.09510876220501));
#22898=CARTESIAN_POINT('Ctrl Pts',(-0.599241616422144,-1.,2.09954930865331));
#22899=CARTESIAN_POINT('Ctrl Pts',(-0.603932030738212,-1.,2.10397049887709));
#22900=CARTESIAN_POINT('Ctrl Pts',(-0.607711315456826,-1.,2.10749199615859));
#22901=CARTESIAN_POINT('Ctrl Pts',(-0.610560911691113,-1.,2.11012443807661));
#22902=CARTESIAN_POINT('Ctrl Pts',(-0.61246736556225,-1.,2.11187554260142));
#22903=CARTESIAN_POINT('Ctrl Pts',(-0.61342227326009,-1.,2.11275013067528));
#22904=CARTESIAN_POINT('',(-0.745574324794401,-1.,2.0698113262342));
#22905=CARTESIAN_POINT('',(-0.61342227326009,-1.,2.11275013067528));
#22906=CARTESIAN_POINT('',(-0.693717979106306,-1.,1.60662857109684));
#22907=CARTESIAN_POINT('Ctrl Pts',(-0.745574324794401,-1.,2.0698113262342));
#22908=CARTESIAN_POINT('Ctrl Pts',(-0.74583279137781,-1.,2.06854248895575));
#22909=CARTESIAN_POINT('Ctrl Pts',(-0.746345871542696,-1.,2.06600523016401));
#22910=CARTESIAN_POINT('Ctrl Pts',(-0.747103932785504,-1.,2.06220058927162));
#22911=CARTESIAN_POINT('Ctrl Pts',(-0.748091554181101,-1.,2.05713023030263));
#22912=CARTESIAN_POINT('Ctrl Pts',(-0.749287468663053,-1.,2.05079645591606));
#22913=CARTESIAN_POINT('Ctrl Pts',(-0.750444657874758,-1.,2.04446689147754));
#22914=CARTESIAN_POINT('Ctrl Pts',(-0.751562963361384,-1.,2.03814160092173));
#22915=CARTESIAN_POINT('Ctrl Pts',(-0.752642180488104,-1.,2.03182068456467));
#22916=CARTESIAN_POINT('Ctrl Pts',(-0.753682061113766,-1.,2.02550428623587));
#22917=CARTESIAN_POINT('Ctrl Pts',(-0.75468233072352,-1.,2.01919259406003));
#22918=CARTESIAN_POINT('Ctrl Pts',(-0.7556427049581,-1.,2.01288584328149));
#22919=CARTESIAN_POINT('Ctrl Pts',(-0.756562904646496,-1.,2.00658431587682));
#22920=CARTESIAN_POINT('Ctrl Pts',(-0.757442676862341,-1.,2.00028834739072));
#22921=CARTESIAN_POINT('Ctrl Pts',(-0.758281796766377,-1.,1.9939983109871));
#22922=CARTESIAN_POINT('Ctrl Pts',(-0.759080037802243,-1.,1.98771456680806));
#22923=CARTESIAN_POINT('Ctrl Pts',(-0.759837147452135,-1.,1.98143741418156));
#22924=CARTESIAN_POINT('Ctrl Pts',(-0.760552825409855,-1.,1.97516705321521));
#22925=CARTESIAN_POINT('Ctrl Pts',(-0.761226690483986,-1.,1.96890351582545));
#22926=CARTESIAN_POINT('Ctrl Pts',(-0.761858300014575,-1.,1.96264672744229));
#22927=CARTESIAN_POINT('Ctrl Pts',(-0.762447203806263,-1.,1.95639665309893));
#22928=CARTESIAN_POINT('Ctrl Pts',(-0.762992990878774,-1.,1.95015342590025));
#22929=CARTESIAN_POINT('Ctrl Pts',(-0.76349533353858,-1.,1.94391746617626));
#22930=CARTESIAN_POINT('Ctrl Pts',(-0.763954049121393,-1.,1.93768964875867));
#22931=CARTESIAN_POINT('Ctrl Pts',(-0.764369010673889,-1.,1.93147105496367));
#22932=CARTESIAN_POINT('Ctrl Pts',(-0.764740025488189,-1.,1.92526263537041));
#22933=CARTESIAN_POINT('Ctrl Pts',(-0.765066729667095,-1.,1.91906491634197));
#22934=CARTESIAN_POINT('Ctrl Pts',(-0.765348465884739,-1.,1.91287765805174));
#22935=CARTESIAN_POINT('Ctrl Pts',(-0.765584196937936,-1.,1.90669961402362));
#22936=CARTESIAN_POINT('Ctrl Pts',(-0.765772772593395,-1.,1.90052930393599));
#22937=CARTESIAN_POINT('Ctrl Pts',(-0.765913193856979,-1.,1.89436577771389));
#22938=CARTESIAN_POINT('Ctrl Pts',(-0.76600483706209,-1.,1.88820926433409));
#22939=CARTESIAN_POINT('Ctrl Pts',(-0.766047794851869,-1.,1.88206215302561));
#22940=CARTESIAN_POINT('Ctrl Pts',(-0.766042837036759,-1.,1.87592888967886));
#22941=CARTESIAN_POINT('Ctrl Pts',(-0.765990708546111,-1.,1.86981398314345));
#22942=CARTESIAN_POINT('Ctrl Pts',(-0.765891519092557,-1.,1.86372027063314));
#22943=CARTESIAN_POINT('Ctrl Pts',(-0.765744212909305,-1.,1.85764741390391));
#22944=CARTESIAN_POINT('Ctrl Pts',(-0.765545710619023,-1.,1.85158945130054));
#22945=CARTESIAN_POINT('Ctrl Pts',(-0.765291664861971,-1.,1.8455369887591));
#22946=CARTESIAN_POINT('Ctrl Pts',(-0.764978057881687,-1.,1.83948181064823));
#22947=CARTESIAN_POINT('Ctrl Pts',(-0.764602549687845,-1.,1.8334207722714));
#22948=CARTESIAN_POINT('Ctrl Pts',(-0.764165902606055,-1.,1.8273599120008));
#22949=CARTESIAN_POINT('Ctrl Pts',(-0.763673465462854,-1.,1.82131873145297));
#22950=CARTESIAN_POINT('Ctrl Pts',(-0.763132003836783,-1.,1.81532118405566));
#22951=CARTESIAN_POINT('Ctrl Pts',(-0.762546129464036,-1.,1.80938551463989));
#22952=CARTESIAN_POINT('Ctrl Pts',(-0.761915336443516,-1.,1.80351583877334));
#22953=CARTESIAN_POINT('Ctrl Pts',(-0.761229695230359,-1.,1.79768986997735));
#22954=CARTESIAN_POINT('Ctrl Pts',(-0.760469555880425,-1.,1.79185815610802));
#22955=CARTESIAN_POINT('Ctrl Pts',(-0.759614401109868,-1.,1.78596964884526));
#22956=CARTESIAN_POINT('Ctrl Pts',(-0.75865062667738,-1.,1.77999411220912));
#22957=CARTESIAN_POINT('Ctrl Pts',(-0.757578264077238,-1.,1.77394167108342));
#22958=CARTESIAN_POINT('Ctrl Pts',(-0.756421896028403,-1.,1.76789396003141));
#22959=CARTESIAN_POINT('Ctrl Pts',(-0.755220979975262,-1.,1.7619781724032));
#22960=CARTESIAN_POINT('Ctrl Pts',(-0.75400925402848,-1.,1.75631083600175));
#22961=CARTESIAN_POINT('Ctrl Pts',(-0.752797683531377,-1.,1.75095139468809));
#22962=CARTESIAN_POINT('Ctrl Pts',(-0.751555614163629,-1.,1.74585086852298));
#22963=CARTESIAN_POINT('Ctrl Pts',(-0.75019343597954,-1.,1.74080458266705));
#22964=CARTESIAN_POINT('Ctrl Pts',(-0.748582462954855,-1.,1.73550351679848));
#22965=CARTESIAN_POINT('Ctrl Pts',(-0.746574710096436,-1.,1.72958533647399));
#22966=CARTESIAN_POINT('Ctrl Pts',(-0.744021445433764,-1.,1.7226822991693));
#22967=CARTESIAN_POINT('Ctrl Pts',(-0.740795162032088,-1.,1.71447789751927));
#22968=CARTESIAN_POINT('Ctrl Pts',(-0.736799665724771,-1.,1.70473309006121));
#22969=CARTESIAN_POINT('Ctrl Pts',(-0.731963238697195,-1.,1.69326921975743));
#22970=CARTESIAN_POINT('Ctrl Pts',(-0.726235967997433,-1.,1.67996158455503));
#22971=CARTESIAN_POINT('Ctrl Pts',(-0.719585433804282,-1.,1.6647288055568));
#22972=CARTESIAN_POINT('Ctrl Pts',(-0.711993139355394,-1.,1.64752408832016));
#22973=CARTESIAN_POINT('Ctrl Pts',(-0.705159151988319,-1.,1.63216541664676));
#22974=CARTESIAN_POINT('Ctrl Pts',(-0.699605146405088,-1.,1.61974673472612));
#22975=CARTESIAN_POINT('Ctrl Pts',(-0.695712097881194,-1.,1.61106790958151));
#22976=CARTESIAN_POINT('Ctrl Pts',(-0.693717979106306,-1.,1.60662857109684));
#22977=CARTESIAN_POINT('',(-0.892032620296855,-1.,1.5055822144029));
#22978=CARTESIAN_POINT('Origin',(0.,-1.,0.));
#22979=CARTESIAN_POINT('',(-1.23627494547115,-1.,1.81978687191668));
#22980=CARTESIAN_POINT('Ctrl Pts',(-0.892032620296855,-1.,1.5055822144029));
#22981=CARTESIAN_POINT('Ctrl Pts',(-0.894452006964543,-1.,1.50980486806688));
#22982=CARTESIAN_POINT('Ctrl Pts',(-0.899185047483511,-1.,1.51805569590094));
#22983=CARTESIAN_POINT('Ctrl Pts',(-0.905967409625651,-1.,1.52984849887993));
#22984=CARTESIAN_POINT('Ctrl Pts',(-0.914375919026456,-1.,1.54440491149498));
#22985=CARTESIAN_POINT('Ctrl Pts',(-0.923832188944341,-1.,1.56065988578893));
#22986=CARTESIAN_POINT('Ctrl Pts',(-0.932246680108685,-1.,1.57499388382243));
#22987=CARTESIAN_POINT('Ctrl Pts',(-0.939646377893399,-1.,1.58744937487176));
#22988=CARTESIAN_POINT('Ctrl Pts',(-0.946078063315257,-1.,1.59810042043673));
#22989=CARTESIAN_POINT('Ctrl Pts',(-0.951613284356035,-1.,1.60706069896936));
#22990=CARTESIAN_POINT('Ctrl Pts',(-0.956354422920671,-1.,1.61449324337085));
#22991=CARTESIAN_POINT('Ctrl Pts',(-0.960438326101729,-1.,1.62061638140221));
#22992=CARTESIAN_POINT('Ctrl Pts',(-0.964046107040536,-1.,1.62571930670187));
#22993=CARTESIAN_POINT('Ctrl Pts',(-0.967387853230345,-1.,1.63013849959461));
#22994=CARTESIAN_POINT('Ctrl Pts',(-0.970669715997509,-1.,1.63420665729798));
#22995=CARTESIAN_POINT('Ctrl Pts',(-0.974066058287418,-1.,1.63820952658144));
#22996=CARTESIAN_POINT('Ctrl Pts',(-0.977689794119416,-1.,1.64233990826687));
#22997=CARTESIAN_POINT('Ctrl Pts',(-0.981562530939489,-1.,1.64665139190656));
#22998=CARTESIAN_POINT('Ctrl Pts',(-0.985642622920821,-1.,1.65110016612638));
#22999=CARTESIAN_POINT('Ctrl Pts',(-0.989855627854165,-1.,1.65559044289699));
#23000=CARTESIAN_POINT('Ctrl Pts',(-0.994121836661306,-1.,1.66001553809947));
#23001=CARTESIAN_POINT('Ctrl Pts',(-0.998389654952758,-1.,1.66430758030376));
#23002=CARTESIAN_POINT('Ctrl Pts',(-1.00265091003727,-1.,1.66846059277303));
#23003=CARTESIAN_POINT('Ctrl Pts',(-1.00692206696414,-1.,1.67250335383293));
#23004=CARTESIAN_POINT('Ctrl Pts',(-1.01123236493511,-1.,1.67648246776464));
#23005=CARTESIAN_POINT('Ctrl Pts',(-1.01561026162773,-1.,1.68044289894798));
#23006=CARTESIAN_POINT('Ctrl Pts',(-1.02006795074201,-1.,1.68440578021706));
#23007=CARTESIAN_POINT('Ctrl Pts',(-1.02460180535255,-1.,1.68836910178447));
#23008=CARTESIAN_POINT('Ctrl Pts',(-1.02919977579147,-1.,1.69231840863458));
#23009=CARTESIAN_POINT('Ctrl Pts',(-1.03384646003588,-1.,1.69623414782771));
#23010=CARTESIAN_POINT('Ctrl Pts',(-1.03852922490789,-1.,1.70010052930962));
#23011=CARTESIAN_POINT('Ctrl Pts',(-1.04324363334554,-1.,1.70391338707982));
#23012=CARTESIAN_POINT('Ctrl Pts',(-1.04799085404995,-1.,1.70767646263649));
#23013=CARTESIAN_POINT('Ctrl Pts',(-1.05277517202855,-1.,1.71139783543989));
#23014=CARTESIAN_POINT('Ctrl Pts',(-1.05760163192479,-1.,1.7150865442702));
#23015=CARTESIAN_POINT('Ctrl Pts',(-1.06247324680647,-1.,1.71874858456904));
#23016=CARTESIAN_POINT('Ctrl Pts',(-1.06738966975462,-1.,1.72238500928453));
#23017=CARTESIAN_POINT('Ctrl Pts',(-1.07234866990252,-1.,1.72599406198488));
#23018=CARTESIAN_POINT('Ctrl Pts',(-1.0773470373727,-1.,1.72957248977424));
#23019=CARTESIAN_POINT('Ctrl Pts',(-1.08238162784749,-1.,1.73311705663407));
#23020=CARTESIAN_POINT('Ctrl Pts',(-1.08745056285427,-1.,1.73662628326091));
#23021=CARTESIAN_POINT('Ctrl Pts',(-1.09255329056493,-1.,1.74010053962247));
#23022=CARTESIAN_POINT('Ctrl Pts',(-1.09768999241225,-1.,1.74354119236208));
#23023=CARTESIAN_POINT('Ctrl Pts',(-1.10286118991143,-1.,1.74695004214923));
#23024=CARTESIAN_POINT('Ctrl Pts',(-1.10806728183007,-1.,1.7503286607592));
#23025=CARTESIAN_POINT('Ctrl Pts',(-1.11330807582551,-1.,1.7536777209463));
#23026=CARTESIAN_POINT('Ctrl Pts',(-1.11858293216763,-1.,1.75699720772105));
#23027=CARTESIAN_POINT('Ctrl Pts',(-1.12389096855086,-1.,1.76028671825096));
#23028=CARTESIAN_POINT('Ctrl Pts',(-1.12923123555075,-1.,1.7635457196617));
#23029=CARTESIAN_POINT('Ctrl Pts',(-1.1346029180462,-1.,1.76677384551862));
#23030=CARTESIAN_POINT('Ctrl Pts',(-1.14000548336975,-1.,1.76997111386769));
#23031=CARTESIAN_POINT('Ctrl Pts',(-1.1454385822692,-1.,1.77313777896194));
#23032=CARTESIAN_POINT('Ctrl Pts',(-1.15090197841515,-1.,1.7762742255701));
#23033=CARTESIAN_POINT('Ctrl Pts',(-1.15639547194698,-1.,1.77938085564275));
#23034=CARTESIAN_POINT('Ctrl Pts',(-1.16191881298499,-1.,1.78245795881009));
#23035=CARTESIAN_POINT('Ctrl Pts',(-1.16747166312303,-1.,1.78550566040443));
#23036=CARTESIAN_POINT('Ctrl Pts',(-1.17305363177328,-1.,1.78852398877616));
#23037=CARTESIAN_POINT('Ctrl Pts',(-1.17866429440809,-1.,1.79151291552689));
#23038=CARTESIAN_POINT('Ctrl Pts',(-1.18430321697432,-1.,1.79447240321515));
#23039=CARTESIAN_POINT('Ctrl Pts',(-1.18996997934445,-1.,1.79740245923478));
#23040=CARTESIAN_POINT('Ctrl Pts',(-1.19566418930242,-1.,1.80030314369879));
#23041=CARTESIAN_POINT('Ctrl Pts',(-1.20138548938974,-1.,1.80317454838603));
#23042=CARTESIAN_POINT('Ctrl Pts',(-1.20713356605475,-1.,1.80601678480707));
#23043=CARTESIAN_POINT('Ctrl Pts',(-1.21290815708314,-1.,1.80882996917129));
#23044=CARTESIAN_POINT('Ctrl Pts',(-1.21870906103557,-1.,1.81161420806656));
#23045=CARTESIAN_POINT('Ctrl Pts',(-1.2245361330495,-1.,1.81436959210434));
#23046=CARTESIAN_POINT('Ctrl Pts',(-1.2292186489137,-1.,1.8165508718364));
#23047=CARTESIAN_POINT('Ctrl Pts',(-1.2327422452705,-1.,1.81817389921279));
#23048=CARTESIAN_POINT('Ctrl Pts',(-1.23509651170476,-1.,1.81925017193666));
#23049=CARTESIAN_POINT('Ctrl Pts',(-1.23627494547115,-1.,1.81978687191668));
#23050=CARTESIAN_POINT('',(-1.34869019493419,-1.,1.73811241238545));
#23051=CARTESIAN_POINT('',(-1.23627494547115,-1.,1.81978687191668));
#23052=CARTESIAN_POINT('',(-1.15624053661742,-1.,1.31362392696032));
#23053=CARTESIAN_POINT('Ctrl Pts',(-1.34869019493419,-1.,1.73811241238545));
#23054=CARTESIAN_POINT('Ctrl Pts',(-1.34854391898045,-1.,1.73682580585691));
#23055=CARTESIAN_POINT('Ctrl Pts',(-1.34824783112887,-1.,1.73425417885907));
#23056=CARTESIAN_POINT('Ctrl Pts',(-1.34779309152035,-1.,1.7304014965394));
#23057=CARTESIAN_POINT('Ctrl Pts',(-1.34716554819527,-1.,1.72527410680674));
#23058=CARTESIAN_POINT('Ctrl Pts',(-1.34634568653227,-1.,1.7188807715049));
#23059=CARTESIAN_POINT('Ctrl Pts',(-1.34549029589416,-1.,1.71250340686822));
#23060=CARTESIAN_POINT('Ctrl Pts',(-1.34459924533831,-1.,1.70614212266738));
#23061=CARTESIAN_POINT('Ctrl Pts',(-1.34367237124483,-1.,1.69979707754427));
#23062=CARTESIAN_POINT('Ctrl Pts',(-1.34270948206319,-1.,1.6934684849687));
#23063=CARTESIAN_POINT('Ctrl Pts',(-1.341710374848,-1.,1.68715660868764));
#23064=CARTESIAN_POINT('Ctrl Pts',(-1.34067485185203,-1.,1.68086176030362));
#23065=CARTESIAN_POINT('Ctrl Pts',(-1.3396027347034,-1.,1.67458429426086));
#23066=CARTESIAN_POINT('Ctrl Pts',(-1.33849388654388,-1.,1.66832460783989));
#23067=CARTESIAN_POINT('Ctrl Pts',(-1.33734820885262,-1.,1.66208312541983));
#23068=CARTESIAN_POINT('Ctrl Pts',(-1.33616559745172,-1.,1.65586025952593));
#23069=CARTESIAN_POINT('Ctrl Pts',(-1.33494590467993,-1.,1.6496563728683));
#23070=CARTESIAN_POINT('Ctrl Pts',(-1.33368890676572,-1.,1.6434717485603));
#23071=CARTESIAN_POINT('Ctrl Pts',(-1.33239425103724,-1.,1.63730653475089));
#23072=CARTESIAN_POINT('Ctrl Pts',(-1.33106149345645,-1.,1.63116079730923));
#23073=CARTESIAN_POINT('Ctrl Pts',(-1.3296901950568,-1.,1.62503464209797));
#23074=CARTESIAN_POINT('Ctrl Pts',(-1.32828000610449,-1.,1.61892832270724));
#23075=CARTESIAN_POINT('Ctrl Pts',(-1.32683074483356,-1.,1.6128423401575));
#23076=CARTESIAN_POINT('Ctrl Pts',(-1.32534250785782,-1.,1.60677758290954));
#23077=CARTESIAN_POINT('Ctrl Pts',(-1.32381550858256,-1.,1.60073511858687));
#23078=CARTESIAN_POINT('Ctrl Pts',(-1.32224985747682,-1.,1.59471591079403));
#23079=CARTESIAN_POINT('Ctrl Pts',(-1.32064537110892,-1.,1.58872057258245));
#23080=CARTESIAN_POINT('Ctrl Pts',(-1.31900135021432,-1.,1.58274907898834));
#23081=CARTESIAN_POINT('Ctrl Pts',(-1.31731642317187,-1.,1.5768005650559));
#23082=CARTESIAN_POINT('Ctrl Pts',(-1.31558903860016,-1.,1.57087397835723));
#23083=CARTESIAN_POINT('Ctrl Pts',(-1.31381795281002,-1.,1.56496872402353));
#23084=CARTESIAN_POINT('Ctrl Pts',(-1.31200264341696,-1.,1.55908521254821));
#23085=CARTESIAN_POINT('Ctrl Pts',(-1.31014393684222,-1.,1.55322568759481));
#23086=CARTESIAN_POINT('Ctrl Pts',(-1.30824393907473,-1.,1.54739413957185));
#23087=CARTESIAN_POINT('Ctrl Pts',(-1.30630475189556,-1.,1.54159462645432));
#23088=CARTESIAN_POINT('Ctrl Pts',(-1.30432735639489,-1.,1.53582981268977));
#23089=CARTESIAN_POINT('Ctrl Pts',(-1.30231064395568,-1.,1.53009970283891));
#23090=CARTESIAN_POINT('Ctrl Pts',(-1.30024984366328,-1.,1.52439957861062));
#23091=CARTESIAN_POINT('Ctrl Pts',(-1.29813791800747,-1.,1.51872184912724));
#23092=CARTESIAN_POINT('Ctrl Pts',(-1.29596850710509,-1.,1.51305994241402));
#23093=CARTESIAN_POINT('Ctrl Pts',(-1.29373841372842,-1.,1.50741159078365));
#23094=CARTESIAN_POINT('Ctrl Pts',(-1.29145022885181,-1.,1.50178230149776));
#23095=CARTESIAN_POINT('Ctrl Pts',(-1.28911506584254,-1.,1.49618896881754));
#23096=CARTESIAN_POINT('Ctrl Pts',(-1.2867467611644,-1.,1.4906522831278));
#23097=CARTESIAN_POINT('Ctrl Pts',(-1.28435533880201,-1.,1.4851881711891));
#23098=CARTESIAN_POINT('Ctrl Pts',(-1.28194158939517,-1.,1.47980070347095));
#23099=CARTESIAN_POINT('Ctrl Pts',(-1.2794891824849,-1.,1.4744717526707));
#23100=CARTESIAN_POINT('Ctrl Pts',(-1.27696414831089,-1.,1.46916035917133));
#23101=CARTESIAN_POINT('Ctrl Pts',(-1.27433119897822,-1.,1.46382431332476));
#23102=CARTESIAN_POINT('Ctrl Pts',(-1.27156805265289,-1.,1.45843906294697));
#23103=CARTESIAN_POINT('Ctrl Pts',(-1.2686778680489,-1.,1.45301422764247));
#23104=CARTESIAN_POINT('Ctrl Pts',(-1.26570925118868,-1.,1.44761985001662));
#23105=CARTESIAN_POINT('Ctrl Pts',(-1.26273903323859,-1.,1.44236470511303));
#23106=CARTESIAN_POINT('Ctrl Pts',(-1.25983531012005,-1.,1.43734919180848));
#23107=CARTESIAN_POINT('Ctrl Pts',(-1.25702687965755,-1.,1.43262645609691));
#23108=CARTESIAN_POINT('Ctrl Pts',(-1.25426945222639,-1.,1.42815938799387));
#23109=CARTESIAN_POINT('Ctrl Pts',(-1.2514145557001,-1.,1.42378102115575));
#23110=CARTESIAN_POINT('Ctrl Pts',(-1.24824430986571,-1.,1.41923722596025));
#23111=CARTESIAN_POINT('Ctrl Pts',(-1.24450600513056,-1.,1.41422913175179));
#23112=CARTESIAN_POINT('Ctrl Pts',(-1.23994455029534,-1.,1.40845295531283));
#23113=CARTESIAN_POINT('Ctrl Pts',(-1.23434087290423,-1.,1.40164708206106));
#23114=CARTESIAN_POINT('Ctrl Pts',(-1.22752961899387,-1.,1.39361389568796));
#23115=CARTESIAN_POINT('Ctrl Pts',(-1.21938737280852,-1.,1.38420564527715));
#23116=CARTESIAN_POINT('Ctrl Pts',(-1.20982812925645,-1.,1.37331915607905));
#23117=CARTESIAN_POINT('Ctrl Pts',(-1.1987959077932,-1.,1.36088705043885));
#23118=CARTESIAN_POINT('Ctrl Pts',(-1.18625865667441,-1.,1.34687054001093));
#23119=CARTESIAN_POINT('Ctrl Pts',(-1.17501305789857,-1.,1.33437539347008));
#23120=CARTESIAN_POINT('Ctrl Pts',(-1.16589330093588,-1.,1.32428080721772));
#23121=CARTESIAN_POINT('Ctrl Pts',(-1.15950888730809,-1.,1.31722977216397));
#23122=CARTESIAN_POINT('Ctrl Pts',(-1.15624053661742,-1.,1.31362392696032));
#23123=CARTESIAN_POINT('',(-1.31362392696033,-1.,1.15624053661742));
#23124=CARTESIAN_POINT('Origin',(0.,-1.,0.));
#23125=CARTESIAN_POINT('',(-1.73811241238545,-1.,1.34869019493419));
#23126=CARTESIAN_POINT('Ctrl Pts',(-1.31362392696033,-1.,1.15624053661742));
#23127=CARTESIAN_POINT('Ctrl Pts',(-1.3172297721596,-1.,1.15950888730433));
#23128=CARTESIAN_POINT('Ctrl Pts',(-1.32428080720544,-1.,1.16589330092532));
#23129=CARTESIAN_POINT('Ctrl Pts',(-1.33437539344842,-1.,1.17501305787994));
#23130=CARTESIAN_POINT('Ctrl Pts',(-1.34687053998157,-1.,1.18625865664915));
#23131=CARTESIAN_POINT('Ctrl Pts',(-1.36088705040677,-1.,1.1987959077656));
#23132=CARTESIAN_POINT('Ctrl Pts',(-1.37331915604962,-1.,1.20982812923113));
#23133=CARTESIAN_POINT('Ctrl Pts',(-1.38420564525391,-1.,1.21938737278853));
#23134=CARTESIAN_POINT('Ctrl Pts',(-1.39361389567257,-1.,1.22752961898063));
#23135=CARTESIAN_POINT('Ctrl Pts',(-1.40164708205345,-1.,1.23434087289768));
#23136=CARTESIAN_POINT('Ctrl Pts',(-1.40845295531151,-1.,1.23994455029421));
#23137=CARTESIAN_POINT('Ctrl Pts',(-1.41422913175437,-1.,1.24450600513278));
#23138=CARTESIAN_POINT('Ctrl Pts',(-1.41923722596421,-1.,1.24824430986911));
#23139=CARTESIAN_POINT('Ctrl Pts',(-1.42378102115911,-1.,1.25141455570299));
#23140=CARTESIAN_POINT('Ctrl Pts',(-1.42815938799555,-1.,1.25426945222783));
#23141=CARTESIAN_POINT('Ctrl Pts',(-1.43262645609679,-1.,1.25702687965744));
#23142=CARTESIAN_POINT('Ctrl Pts',(-1.43734919180719,-1.,1.25983531011894));
#23143=CARTESIAN_POINT('Ctrl Pts',(-1.44236470511145,-1.,1.26273903323723));
#23144=CARTESIAN_POINT('Ctrl Pts',(-1.44761985001544,-1.,1.26570925118767));
#23145=CARTESIAN_POINT('Ctrl Pts',(-1.45301422764205,-1.,1.26867786804854));
#23146=CARTESIAN_POINT('Ctrl Pts',(-1.45843906294725,-1.,1.27156805265312));
#23147=CARTESIAN_POINT('Ctrl Pts',(-1.4638243133254,-1.,1.27433119897877));
#23148=CARTESIAN_POINT('Ctrl Pts',(-1.46916035917197,-1.,1.27696414831144));
#23149=CARTESIAN_POINT('Ctrl Pts',(-1.4744717526711,-1.,1.27948918248524));
#23150=CARTESIAN_POINT('Ctrl Pts',(-1.47980070347102,-1.,1.28194158939522));
#23151=CARTESIAN_POINT('Ctrl Pts',(-1.48518817118891,-1.,1.28435533880184));
#23152=CARTESIAN_POINT('Ctrl Pts',(-1.4906522831275,-1.,1.28674676116415));
#23153=CARTESIAN_POINT('Ctrl Pts',(-1.49618896881729,-1.,1.28911506584232));
#23154=CARTESIAN_POINT('Ctrl Pts',(-1.50178230149764,-1.,1.29145022885171));
#23155=CARTESIAN_POINT('Ctrl Pts',(-1.50741159078367,-1.,1.29373841372843));
#23156=CARTESIAN_POINT('Ctrl Pts',(-1.51305994241412,-1.,1.29596850710518));
#23157=CARTESIAN_POINT('Ctrl Pts',(-1.51872184912735,-1.,1.29813791800757));
#23158=CARTESIAN_POINT('Ctrl Pts',(-1.5243995786107,-1.,1.30024984366334));
#23159=CARTESIAN_POINT('Ctrl Pts',(-1.53009970283893,-1.,1.3023106439557));
#23160=CARTESIAN_POINT('Ctrl Pts',(-1.53582981268976,-1.,1.30432735639487));
#23161=CARTESIAN_POINT('Ctrl Pts',(-1.54159462645428,-1.,1.30630475189553));
#23162=CARTESIAN_POINT('Ctrl Pts',(-1.54739413957183,-1.,1.30824393907471));
#23163=CARTESIAN_POINT('Ctrl Pts',(-1.55322568759481,-1.,1.31014393684221));
#23164=CARTESIAN_POINT('Ctrl Pts',(-1.55908521254822,-1.,1.31200264341696));
#23165=CARTESIAN_POINT('Ctrl Pts',(-1.56496872402352,-1.,1.31381795281002));
#23166=CARTESIAN_POINT('Ctrl Pts',(-1.57087397835721,-1.,1.31558903860015));
#23167=CARTESIAN_POINT('Ctrl Pts',(-1.57680056505585,-1.,1.31731642317183));
#23168=CARTESIAN_POINT('Ctrl Pts',(-1.58274907898829,-1.,1.31900135021428));
#23169=CARTESIAN_POINT('Ctrl Pts',(-1.58872057258244,-1.,1.32064537110891));
#23170=CARTESIAN_POINT('Ctrl Pts',(-1.59471591079408,-1.,1.32224985747686));
#23171=CARTESIAN_POINT('Ctrl Pts',(-1.600735118587,-1.,1.32381550858266));
#23172=CARTESIAN_POINT('Ctrl Pts',(-1.6067775829097,-1.,1.32534250785794));
#23173=CARTESIAN_POINT('Ctrl Pts',(-1.61284234015762,-1.,1.32683074483365));
#23174=CARTESIAN_POINT('Ctrl Pts',(-1.61892832270723,-1.,1.32828000610448));
#23175=CARTESIAN_POINT('Ctrl Pts',(-1.62503464209777,-1.,1.32969019505665));
#23176=CARTESIAN_POINT('Ctrl Pts',(-1.63116079730887,-1.,1.33106149345618));
#23177=CARTESIAN_POINT('Ctrl Pts',(-1.6373065347505,-1.,1.33239425103694));
#23178=CARTESIAN_POINT('Ctrl Pts',(-1.64347174856007,-1.,1.33368890676554));
#23179=CARTESIAN_POINT('Ctrl Pts',(-1.64965637286843,-1.,1.33494590468003));
#23180=CARTESIAN_POINT('Ctrl Pts',(-1.65586025952651,-1.,1.33616559745217));
#23181=CARTESIAN_POINT('Ctrl Pts',(-1.66208312542073,-1.,1.33734820885331));
#23182=CARTESIAN_POINT('Ctrl Pts',(-1.66832460784078,-1.,1.33849388654458));
#23183=CARTESIAN_POINT('Ctrl Pts',(-1.67458429426126,-1.,1.33960273470372));
#23184=CARTESIAN_POINT('Ctrl Pts',(-1.68086176030308,-1.,1.3406748518516));
#23185=CARTESIAN_POINT('Ctrl Pts',(-1.68715660868602,-1.,1.34171037484673));
#23186=CARTESIAN_POINT('Ctrl Pts',(-1.6934684849664,-1.,1.34270948206139));
#23187=CARTESIAN_POINT('Ctrl Pts',(-1.69979707754221,-1.,1.34367237124322));
#23188=CARTESIAN_POINT('Ctrl Pts',(-1.70614212266676,-1.,1.34459924533783));
#23189=CARTESIAN_POINT('Ctrl Pts',(-1.71250340687011,-1.,1.34549029589563));
#23190=CARTESIAN_POINT('Ctrl Pts',(-1.7188807715095,-1.,1.34634568653586));
#23191=CARTESIAN_POINT('Ctrl Pts',(-1.72527410681298,-1.,1.34716554820013));
#23192=CARTESIAN_POINT('Ctrl Pts',(-1.73040149654497,-1.,1.3477930915247));
#23193=CARTESIAN_POINT('Ctrl Pts',(-1.73425417886255,-1.,1.34824783113158));
#23194=CARTESIAN_POINT('Ctrl Pts',(-1.73682580585819,-1.,1.34854391898145));
#23195=CARTESIAN_POINT('Ctrl Pts',(-1.73811241238545,-1.,1.34869019493419));
#23196=CARTESIAN_POINT('',(-1.81978687191668,-1.,1.23627494547115));
#23197=CARTESIAN_POINT('',(-1.73811241238545,-1.,1.34869019493419));
#23198=CARTESIAN_POINT('',(-1.5055822144029,-1.,0.892032620296855));
#23199=CARTESIAN_POINT('Ctrl Pts',(-1.81978687191668,-1.,1.23627494547115));
#23200=CARTESIAN_POINT('Ctrl Pts',(-1.81925017193531,-1.,1.23509651170384));
#23201=CARTESIAN_POINT('Ctrl Pts',(-1.81817389920914,-1.,1.23274224526804));
#23202=CARTESIAN_POINT('Ctrl Pts',(-1.81655087183054,-1.,1.22921864890975));
#23203=CARTESIAN_POINT('Ctrl Pts',(-1.81436959209778,-1.,1.22453613304507));
#23204=CARTESIAN_POINT('Ctrl Pts',(-1.81161420806172,-1.,1.2187090610323));
#23205=CARTESIAN_POINT('Ctrl Pts',(-1.80882996916931,-1.,1.2129081570818));
#23206=CARTESIAN_POINT('Ctrl Pts',(-1.80601678480772,-1.,1.20713356605519));
#23207=CARTESIAN_POINT('Ctrl Pts',(-1.8031745483882,-1.,1.2013854893912));
#23208=CARTESIAN_POINT('Ctrl Pts',(-1.80030314370121,-1.,1.19566418930405));
#23209=CARTESIAN_POINT('Ctrl Pts',(-1.79740245923649,-1.,1.1899699793456));
#23210=CARTESIAN_POINT('Ctrl Pts',(-1.79447240321572,-1.,1.18430321697471));
#23211=CARTESIAN_POINT('Ctrl Pts',(-1.79151291552646,-1.,1.17866429440781));
#23212=CARTESIAN_POINT('Ctrl Pts',(-1.78852398877523,-1.,1.17305363177265));
#23213=CARTESIAN_POINT('Ctrl Pts',(-1.78550566040349,-1.,1.16747166312239));
#23214=CARTESIAN_POINT('Ctrl Pts',(-1.78245795880949,-1.,1.16191881298458));
#23215=CARTESIAN_POINT('Ctrl Pts',(-1.77938085564261,-1.,1.15639547194689));
#23216=CARTESIAN_POINT('Ctrl Pts',(-1.77627422557034,-1.,1.15090197841531));
#23217=CARTESIAN_POINT('Ctrl Pts',(-1.77313777896234,-1.,1.14543858226948));
#23218=CARTESIAN_POINT('Ctrl Pts',(-1.76997111386806,-1.,1.14000548337));
#23219=CARTESIAN_POINT('Ctrl Pts',(-1.76677384551883,-1.,1.13460291804635));
#23220=CARTESIAN_POINT('Ctrl Pts',(-1.76354571966171,-1.,1.12923123555076));
#23221=CARTESIAN_POINT('Ctrl Pts',(-1.76028671825084,-1.,1.12389096855078));
#23222=CARTESIAN_POINT('Ctrl Pts',(-1.75699720772089,-1.,1.11858293216752));
#23223=CARTESIAN_POINT('Ctrl Pts',(-1.75367772094617,-1.,1.11330807582542));
#23224=CARTESIAN_POINT('Ctrl Pts',(-1.75032866075914,-1.,1.10806728183003));
#23225=CARTESIAN_POINT('Ctrl Pts',(-1.74695004214924,-1.,1.10286118991144));
#23226=CARTESIAN_POINT('Ctrl Pts',(-1.74354119236212,-1.,1.09768999241229));
#23227=CARTESIAN_POINT('Ctrl Pts',(-1.74010053962252,-1.,1.09255329056496));
#23228=CARTESIAN_POINT('Ctrl Pts',(-1.73662628326093,-1.,1.08745056285429));
#23229=CARTESIAN_POINT('Ctrl Pts',(-1.73311705663407,-1.,1.08238162784749));
#23230=CARTESIAN_POINT('Ctrl Pts',(-1.72957248977424,-1.,1.0773470373727));
#23231=CARTESIAN_POINT('Ctrl Pts',(-1.72599406198489,-1.,1.07234866990252));
#23232=CARTESIAN_POINT('Ctrl Pts',(-1.72238500928456,-1.,1.06738966975463));
#23233=CARTESIAN_POINT('Ctrl Pts',(-1.71874858456908,-1.,1.0624732468065));
#23234=CARTESIAN_POINT('Ctrl Pts',(-1.71508654427022,-1.,1.05760163192481));
#23235=CARTESIAN_POINT('Ctrl Pts',(-1.71139783543986,-1.,1.05277517202854));
#23236=CARTESIAN_POINT('Ctrl Pts',(-1.70767646263641,-1.,1.0479908540499));
#23237=CARTESIAN_POINT('Ctrl Pts',(-1.70391338707969,-1.,1.04324363334546));
#23238=CARTESIAN_POINT('Ctrl Pts',(-1.70010052930951,-1.,1.03852922490782));
#23239=CARTESIAN_POINT('Ctrl Pts',(-1.69623414782769,-1.,1.03384646003587));
#23240=CARTESIAN_POINT('Ctrl Pts',(-1.69231840863471,-1.,1.02919977579155));
#23241=CARTESIAN_POINT('Ctrl Pts',(-1.68836910178475,-1.,1.02460180535272));
#23242=CARTESIAN_POINT('Ctrl Pts',(-1.68440578021739,-1.,1.02006795074222));
#23243=CARTESIAN_POINT('Ctrl Pts',(-1.6804428989482,-1.,1.01561026162787));
#23244=CARTESIAN_POINT('Ctrl Pts',(-1.67648246776457,-1.,1.01123236493507));
#23245=CARTESIAN_POINT('Ctrl Pts',(-1.67250335383248,-1.,1.00692206696387));
#23246=CARTESIAN_POINT('Ctrl Pts',(-1.66846059277231,-1.,1.00265091003682));
#23247=CARTESIAN_POINT('Ctrl Pts',(-1.66430758030304,-1.,0.998389654952317));
#23248=CARTESIAN_POINT('Ctrl Pts',(-1.66001553809916,-1.,0.994121836661116));
#23249=CARTESIAN_POINT('Ctrl Pts',(-1.65559044289746,-1.,0.98985562785445));
#23250=CARTESIAN_POINT('Ctrl Pts',(-1.6511001661277,-1.,0.985642622921626));
#23251=CARTESIAN_POINT('Ctrl Pts',(-1.64665139190834,-1.,0.981562530940574));
#23252=CARTESIAN_POINT('Ctrl Pts',(-1.64233990826831,-1.,0.977689794120297));
#23253=CARTESIAN_POINT('Ctrl Pts',(-1.63820952658157,-1.,0.974066058287501));
#23254=CARTESIAN_POINT('Ctrl Pts',(-1.63420665729609,-1.,0.970669715996356));
#23255=CARTESIAN_POINT('Ctrl Pts',(-1.63013849959083,-1.,0.967387853228041));
#23256=CARTESIAN_POINT('Ctrl Pts',(-1.6257193066974,-1.,0.964046107037821));
#23257=CARTESIAN_POINT('Ctrl Pts',(-1.62061638139929,-1.,0.960438326099958));
#23258=CARTESIAN_POINT('Ctrl Pts',(-1.61449324337233,-1.,0.956354422921573));
#23259=CARTESIAN_POINT('Ctrl Pts',(-1.60706069897794,-1.,0.951613284361248));
#23260=CARTESIAN_POINT('Ctrl Pts',(-1.59810042045408,-1.,0.946078063325796));
#23261=CARTESIAN_POINT('Ctrl Pts',(-1.58744937489796,-1.,0.939646377909319));
#23262=CARTESIAN_POINT('Ctrl Pts',(-1.57499388385561,-1.,0.932246680128849));
#23263=CARTESIAN_POINT('Ctrl Pts',(-1.56065988582509,-1.,0.923832188966322));
#23264=CARTESIAN_POINT('Ctrl Pts',(-1.54440491152808,-1.,0.91437591904658));
#23265=CARTESIAN_POINT('Ctrl Pts',(-1.52984849890434,-1.,0.905967409640499));
#23266=CARTESIAN_POINT('Ctrl Pts',(-1.51805569591479,-1.,0.89918504749193));
#23267=CARTESIAN_POINT('Ctrl Pts',(-1.50980486807181,-1.,0.894452006967538));
#23268=CARTESIAN_POINT('Ctrl Pts',(-1.5055822144029,-1.,0.892032620296855));
#23269=CARTESIAN_POINT('',(-1.60662857109684,-1.,0.693717979106305));
#23270=CARTESIAN_POINT('Origin',(0.,-1.,0.));
#23271=CARTESIAN_POINT('',(-2.0698113262342,-1.,0.7455743247944));
#23272=CARTESIAN_POINT('Ctrl Pts',(-1.60662857109684,-1.,0.693717979106305));
#23273=CARTESIAN_POINT('Ctrl Pts',(-1.61106790957619,-1.,0.69571209787897));
#23274=CARTESIAN_POINT('Ctrl Pts',(-1.61974673471117,-1.,0.699605146398837));
#23275=CARTESIAN_POINT('Ctrl Pts',(-1.6321654166204,-1.,0.705159151977294));
#23276=CARTESIAN_POINT('Ctrl Pts',(-1.64752408828442,-1.,0.711993139340447));
#23277=CARTESIAN_POINT('Ctrl Pts',(-1.66472880551777,-1.,0.71958543378795));
#23278=CARTESIAN_POINT('Ctrl Pts',(-1.67996158451922,-1.,0.726235967982445));
#23279=CARTESIAN_POINT('Ctrl Pts',(-1.69326921972915,-1.,0.731963238685357));
#23280=CARTESIAN_POINT('Ctrl Pts',(-1.70473309004249,-1.,0.736799665716932));
#23281=CARTESIAN_POINT('Ctrl Pts',(-1.71447789751001,-1.,0.74079516202821));
#23282=CARTESIAN_POINT('Ctrl Pts',(-1.72268229916769,-1.,0.744021445433093));
#23283=CARTESIAN_POINT('Ctrl Pts',(-1.72958533647714,-1.,0.746574710097752));
#23284=CARTESIAN_POINT('Ctrl Pts',(-1.7355035168033,-1.,0.74858246295687));
#23285=CARTESIAN_POINT('Ctrl Pts',(-1.74080458267114,-1.,0.750193435981249));
#23286=CARTESIAN_POINT('Ctrl Pts',(-1.74585086852502,-1.,0.751555614164482));
#23287=CARTESIAN_POINT('Ctrl Pts',(-1.75095139468794,-1.,0.752797683531314));
#23288=CARTESIAN_POINT('Ctrl Pts',(-1.75631083600019,-1.,0.754009254027829));
#23289=CARTESIAN_POINT('Ctrl Pts',(-1.76197817240128,-1.,0.755220979974461));
#23290=CARTESIAN_POINT('Ctrl Pts',(-1.76789396002998,-1.,0.75642189602781));
#23291=CARTESIAN_POINT('Ctrl Pts',(-1.77394167108292,-1.,0.757578264077029));
#23292=CARTESIAN_POINT('Ctrl Pts',(-1.77999411220945,-1.,0.758650626677518));
#23293=CARTESIAN_POINT('Ctrl Pts',(-1.78596964884604,-1.,0.759614401110189));
#23294=CARTESIAN_POINT('Ctrl Pts',(-1.7918581561088,-1.,0.760469555880749));
#23295=CARTESIAN_POINT('Ctrl Pts',(-1.79768986997783,-1.,0.761229695230558));
#23296=CARTESIAN_POINT('Ctrl Pts',(-1.80351583877342,-1.,0.761915336443547));
#23297=CARTESIAN_POINT('Ctrl Pts',(-1.80938551463965,-1.,0.762546129463938));
#23298=CARTESIAN_POINT('Ctrl Pts',(-1.8153211840553,-1.,0.763132003836634));
#23299=CARTESIAN_POINT('Ctrl Pts',(-1.82131873145266,-1.,0.763673465462726));
#23300=CARTESIAN_POINT('Ctrl Pts',(-1.82735991200065,-1.,0.764165902605995));
#23301=CARTESIAN_POINT('Ctrl Pts',(-1.83342077227142,-1.,0.764602549687853));
#23302=CARTESIAN_POINT('Ctrl Pts',(-1.83948181064835,-1.,0.764978057881737));
#23303=CARTESIAN_POINT('Ctrl Pts',(-1.84553698875924,-1.,0.765291664862029));
#23304=CARTESIAN_POINT('Ctrl Pts',(-1.85158945130063,-1.,0.765545710619062));
#23305=CARTESIAN_POINT('Ctrl Pts',(-1.85764741390394,-1.,0.765744212909318));
#23306=CARTESIAN_POINT('Ctrl Pts',(-1.86372027063312,-1.,0.765891519092547));
#23307=CARTESIAN_POINT('Ctrl Pts',(-1.86981398314341,-1.,0.765990708546091));
#23308=CARTESIAN_POINT('Ctrl Pts',(-1.87592888967883,-1.,0.766042837036744));
#23309=CARTESIAN_POINT('Ctrl Pts',(-1.88206215302561,-1.,0.766047794851864));
#23310=CARTESIAN_POINT('Ctrl Pts',(-1.88820926433409,-1.,0.766004837062091));
#23311=CARTESIAN_POINT('Ctrl Pts',(-1.89436577771388,-1.,0.765913193856978));
#23312=CARTESIAN_POINT('Ctrl Pts',(-1.90052930393596,-1.,0.765772772593386));
#23313=CARTESIAN_POINT('Ctrl Pts',(-1.90669961402356,-1.,0.765584196937919));
#23314=CARTESIAN_POINT('Ctrl Pts',(-1.91287765805169,-1.,0.765348465884722));
#23315=CARTESIAN_POINT('Ctrl Pts',(-1.91906491634196,-1.,0.765066729667088));
#23316=CARTESIAN_POINT('Ctrl Pts',(-1.92526263537048,-1.,0.764740025488211));
#23317=CARTESIAN_POINT('Ctrl Pts',(-1.93147105496382,-1.,0.76436901067394));
#23318=CARTESIAN_POINT('Ctrl Pts',(-1.93768964875886,-1.,0.763954049121458));
#23319=CARTESIAN_POINT('Ctrl Pts',(-1.9439174661764,-1.,0.763495333538629));
#23320=CARTESIAN_POINT('Ctrl Pts',(-1.95015342590024,-1.,0.762992990878769));
#23321=CARTESIAN_POINT('Ctrl Pts',(-1.95639665309869,-1.,0.762447203806179));
#23322=CARTESIAN_POINT('Ctrl Pts',(-1.96264672744186,-1.,0.761858300014423));
#23323=CARTESIAN_POINT('Ctrl Pts',(-1.96890351582499,-1.,0.76122669048382));
#23324=CARTESIAN_POINT('Ctrl Pts',(-1.97516705321494,-1.,0.760552825409757));
#23325=CARTESIAN_POINT('Ctrl Pts',(-1.98143741418172,-1.,0.75983714745219));
#23326=CARTESIAN_POINT('Ctrl Pts',(-1.98771456680874,-1.,0.759080037802488));
#23327=CARTESIAN_POINT('Ctrl Pts',(-1.99399831098817,-1.,0.758281796766761));
#23328=CARTESIAN_POINT('Ctrl Pts',(-2.00028834739178,-1.,0.757442676862724));
#23329=CARTESIAN_POINT('Ctrl Pts',(-2.0065843158773,-1.,0.75656290464667));
#23330=CARTESIAN_POINT('Ctrl Pts',(-2.01288584328084,-1.,0.755642704957865));
#23331=CARTESIAN_POINT('Ctrl Pts',(-2.01919259405809,-1.,0.754682330722816));
#23332=CARTESIAN_POINT('Ctrl Pts',(-2.02550428623313,-1.,0.753682061112768));
#23333=CARTESIAN_POINT('Ctrl Pts',(-2.03182068456221,-1.,0.752642180487211));
#23334=CARTESIAN_POINT('Ctrl Pts',(-2.03814160092099,-1.,0.751562963361115));
#23335=CARTESIAN_POINT('Ctrl Pts',(-2.04446689147979,-1.,0.750444657875576));
#23336=CARTESIAN_POINT('Ctrl Pts',(-2.05079645592154,-1.,0.749287468665046));
#23337=CARTESIAN_POINT('Ctrl Pts',(-2.05713023031006,-1.,0.748091554183802));
#23338=CARTESIAN_POINT('Ctrl Pts',(-2.06220058927826,-1.,0.747103932787919));
#23339=CARTESIAN_POINT('Ctrl Pts',(-2.06600523016815,-1.,0.7463458715442));
#23340=CARTESIAN_POINT('Ctrl Pts',(-2.06854248895728,-1.,0.745832791378367));
#23341=CARTESIAN_POINT('Ctrl Pts',(-2.0698113262342,-1.,0.7455743247944));
#23342=CARTESIAN_POINT('',(-2.11275013067528,-1.,0.61342227326009));
#23343=CARTESIAN_POINT('',(-2.0698113262342,-1.,0.7455743247944));
#23344=CARTESIAN_POINT('',(-1.7075470150345,-1.,0.383122945602004));
#23345=CARTESIAN_POINT('Ctrl Pts',(-2.11275013067528,-1.,0.61342227326009));
#23346=CARTESIAN_POINT('Ctrl Pts',(-2.11187554259986,-1.,0.6124673655618));
#23347=CARTESIAN_POINT('Ctrl Pts',(-2.11012443807238,-1.,0.610560911689899));
#23348=CARTESIAN_POINT('Ctrl Pts',(-2.1074919961518,-1.,0.607711315454876));
#23349=CARTESIAN_POINT('Ctrl Pts',(-2.10397049886949,-1.,0.60393203073603));
#23350=CARTESIAN_POINT('Ctrl Pts',(-2.0995493086477,-1.,0.599241616420533));
#23351=CARTESIAN_POINT('Ctrl Pts',(-2.0951087622027,-1.,0.594585006052162));
#23352=CARTESIAN_POINT('Ctrl Pts',(-2.09064881812129,-1.,0.589962365403406));
#23353=CARTESIAN_POINT('Ctrl Pts',(-2.08616943727951,-1.,0.585373918991617));
#23354=CARTESIAN_POINT('Ctrl Pts',(-2.08167059018418,-1.,0.580819952108063));
#23355=CARTESIAN_POINT('Ctrl Pts',(-2.07715226767559,-1.,0.576300797416844));
#23356=CARTESIAN_POINT('Ctrl Pts',(-2.07261449292824,-1.,0.571816823242603));
#23357=CARTESIAN_POINT('Ctrl Pts',(-2.06805732997334,-1.,0.567368421181087));
#23358=CARTESIAN_POINT('Ctrl Pts',(-2.06348090160589,-1.,0.562955993082261));
#23359=CARTESIAN_POINT('Ctrl Pts',(-2.05888537756462,-1.,0.558579940185151));
#23360=CARTESIAN_POINT('Ctrl Pts',(-2.05427091604413,-1.,0.554240657463906));
#23361=CARTESIAN_POINT('Ctrl Pts',(-2.04963761077958,-1.,0.549938525150295));
#23362=CARTESIAN_POINT('Ctrl Pts',(-2.04498544714588,-1.,0.54567390381743));
#23363=CARTESIAN_POINT('Ctrl Pts',(-2.04031422690527,-1.,0.541447120615659));
#23364=CARTESIAN_POINT('Ctrl Pts',(-2.03562362954037,-1.,0.537258489833262));
#23365=CARTESIAN_POINT('Ctrl Pts',(-2.03091336214426,-1.,0.533108355132976));
#23366=CARTESIAN_POINT('Ctrl Pts',(-2.0261832908329,-1.,0.528997127241914));
#23367=CARTESIAN_POINT('Ctrl Pts',(-2.02143356304698,-1.,0.524925318333476));
#23368=CARTESIAN_POINT('Ctrl Pts',(-2.01666477917286,-1.,0.52089359039937));
#23369=CARTESIAN_POINT('Ctrl Pts',(-2.01187773939242,-1.,0.516902681728687));
#23370=CARTESIAN_POINT('Ctrl Pts',(-2.00707309946949,-1.,0.512953306961792));
#23371=CARTESIAN_POINT('Ctrl Pts',(-2.00225107134734,-1.,0.509046069886157));
#23372=CARTESIAN_POINT('Ctrl Pts',(-1.99741107463572,-1.,0.505181361323026));
#23373=CARTESIAN_POINT('Ctrl Pts',(-1.99255149126155,-1.,0.501359287727146));
#23374=CARTESIAN_POINT('Ctrl Pts',(-1.98767044752932,-1.,0.497579909545574));
#23375=CARTESIAN_POINT('Ctrl Pts',(-1.98276658761821,-1.,0.493843476541494));
#23376=CARTESIAN_POINT('Ctrl Pts',(-1.97783973019229,-1.,0.490150627860952));
#23377=CARTESIAN_POINT('Ctrl Pts',(-1.97289186263272,-1.,0.486502692907659));
#23378=CARTESIAN_POINT('Ctrl Pts',(-1.96792703422362,-1.,0.48290166212069));
#23379=CARTESIAN_POINT('Ctrl Pts',(-1.96294933055943,-1.,0.479349583074855));
#23380=CARTESIAN_POINT('Ctrl Pts',(-1.95796111148177,-1.,0.475848034683176));
#23381=CARTESIAN_POINT('Ctrl Pts',(-1.95296148278133,-1.,0.472397672264072));
#23382=CARTESIAN_POINT('Ctrl Pts',(-1.94794381136514,-1.,0.468997482913135));
#23383=CARTESIAN_POINT('Ctrl Pts',(-1.9428979419619,-1.,0.46564546202603));
#23384=CARTESIAN_POINT('Ctrl Pts',(-1.93781486640821,-1.,0.462340031009056));
#23385=CARTESIAN_POINT('Ctrl Pts',(-1.93269066517934,-1.,0.459081234547926));
#23386=CARTESIAN_POINT('Ctrl Pts',(-1.92753067150476,-1.,0.455872005174371));
#23387=CARTESIAN_POINT('Ctrl Pts',(-1.92235380648502,-1.,0.452719478359432));
#23388=CARTESIAN_POINT('Ctrl Pts',(-1.91718342555755,-1.,0.449632260106662));
#23389=CARTESIAN_POINT('Ctrl Pts',(-1.9120369998112,-1.,0.446617343485711));
#23390=CARTESIAN_POINT('Ctrl Pts',(-1.90691756144898,-1.,0.44367755684915));
#23391=CARTESIAN_POINT('Ctrl Pts',(-1.90180124389086,-1.,0.440807833704038));
#23392=CARTESIAN_POINT('Ctrl Pts',(-1.89663648956466,-1.,0.437995003948244));
#23393=CARTESIAN_POINT('Ctrl Pts',(-1.89136993975504,-1.,0.435225660963383));
#23394=CARTESIAN_POINT('Ctrl Pts',(-1.88596913666793,-1.,0.432493038548748));
#23395=CARTESIAN_POINT('Ctrl Pts',(-1.88044229001832,-1.,0.429803062482344));
#23396=CARTESIAN_POINT('Ctrl Pts',(-1.87486989291484,-1.,0.427183828519102));
#23397=CARTESIAN_POINT('Ctrl Pts',(-1.86937803944323,-1.,0.424678177291359));
#23398=CARTESIAN_POINT('Ctrl Pts',(-1.86408083334028,-1.,0.422327307418275));
#23399=CARTESIAN_POINT('Ctrl Pts',(-1.85903281096686,-1.,0.420157287975619));
#23400=CARTESIAN_POINT('Ctrl Pts',(-1.85417632856234,-1.,0.418164129143534));
#23401=CARTESIAN_POINT('Ctrl Pts',(-1.84929312929882,-1.,0.416300022038864));
#23402=CARTESIAN_POINT('Ctrl Pts',(-1.8440575707371,-1.,0.41448743825434));
#23403=CARTESIAN_POINT('Ctrl Pts',(-1.83808953475839,-1.,0.412633125322161));
#23404=CARTESIAN_POINT('Ctrl Pts',(-1.83100408895216,-1.,0.410641256301675));
#23405=CARTESIAN_POINT('Ctrl Pts',(-1.8224702267854,-1.,0.408428948108533));
#23406=CARTESIAN_POINT('Ctrl Pts',(-1.81223801813988,-1.,0.405933518411838));
#23407=CARTESIAN_POINT('Ctrl Pts',(-1.80012077176221,-1.,0.403107976170441));
#23408=CARTESIAN_POINT('Ctrl Pts',(-1.78598826347533,-1.,0.39991940378308));
#23409=CARTESIAN_POINT('Ctrl Pts',(-1.7697556004756,-1.,0.39634619612042));
#23410=CARTESIAN_POINT('Ctrl Pts',(-1.75137405313962,-1.,0.392375812294307));
#23411=CARTESIAN_POINT('Ctrl Pts',(-1.7349317097561,-1.,0.388877023509191));
#23412=CARTESIAN_POINT('Ctrl Pts',(-1.72162022246158,-1.,0.38607079032701));
#23413=CARTESIAN_POINT('Ctrl Pts',(-1.71231062891958,-1.,0.384119047315542));
#23414=CARTESIAN_POINT('Ctrl Pts',(-1.7075470150345,-1.,0.383122945602004));
#23415=CARTESIAN_POINT('',(-1.74236521665491,-1.,0.163289472382896));
#23416=CARTESIAN_POINT('Origin',(0.,-1.,0.));
#23417=CARTESIAN_POINT('',(-2.19890268624765,-1.,0.069476445021958));
#23418=CARTESIAN_POINT('Ctrl Pts',(-1.74236521665491,-1.,0.163289472382896));
#23419=CARTESIAN_POINT('Ctrl Pts',(-1.7472034950333,-1.,0.163814161002002));
#23420=CARTESIAN_POINT('Ctrl Pts',(-1.75666056638427,-1.,0.164834765707158));
#23421=CARTESIAN_POINT('Ctrl Pts',(-1.77018771684844,-1.,0.1662793551464));
#23422=CARTESIAN_POINT('Ctrl Pts',(-1.7869064998507,-1.,0.168032772805197));
#23423=CARTESIAN_POINT('Ctrl Pts',(-1.80561530629706,-1.,0.169936923904608));
#23424=CARTESIAN_POINT('Ctrl Pts',(-1.82215766811545,-1.,0.171554770204119));
#23425=CARTESIAN_POINT('Ctrl Pts',(-1.83658380527692,-1.,0.1728894428919));
#23426=CARTESIAN_POINT('Ctrl Pts',(-1.8489811319852,-1.,0.173946627587731));
#23427=CARTESIAN_POINT('Ctrl Pts',(-1.85948367088837,-1.,0.17473525927603));
#23428=CARTESIAN_POINT('Ctrl Pts',(-1.86828349694799,-1.,0.175268337590758));
#23429=CARTESIAN_POINT('Ctrl Pts',(-1.87563767773588,-1.,0.175563480746485));
#23430=CARTESIAN_POINT('Ctrl Pts',(-1.88188663145367,-1.,0.175644148889698));
#23431=CARTESIAN_POINT('Ctrl Pts',(-1.88742606273259,-1.,0.175538155840648));
#23432=CARTESIAN_POINT('Ctrl Pts',(-1.892646301985,-1.,0.175274276190844));
#23433=CARTESIAN_POINT('Ctrl Pts',(-1.89788101117132,-1.,0.174879405091263));
#23434=CARTESIAN_POINT('Ctrl Pts',(-1.90335253862834,-1.,0.174375518661085));
#23435=CARTESIAN_POINT('Ctrl Pts',(-1.90911693975267,-1.,0.173776635257817));
#23436=CARTESIAN_POINT('Ctrl Pts',(-1.91511429159527,-1.,0.173090695383496));
#23437=CARTESIAN_POINT('Ctrl Pts',(-1.9212233439798,-1.,0.172321621259514));
#23438=CARTESIAN_POINT('Ctrl Pts',(-1.92731093582036,-1.,0.171471191532988));
#23439=CARTESIAN_POINT('Ctrl Pts',(-1.93329183155539,-1.,0.170541253116201));
#23440=CARTESIAN_POINT('Ctrl Pts',(-1.93915639211581,-1.,0.169534904817491));
#23441=CARTESIAN_POINT('Ctrl Pts',(-1.94493757756931,-1.,0.168455741607556));
#23442=CARTESIAN_POINT('Ctrl Pts',(-1.95069027794294,-1.,0.167307501784475));
#23443=CARTESIAN_POINT('Ctrl Pts',(-1.9564675971873,-1.,0.166093592002812));
#23444=CARTESIAN_POINT('Ctrl Pts',(-1.96229379940136,-1.,0.164816568920269));
#23445=CARTESIAN_POINT('Ctrl Pts',(-1.96816512677967,-1.,0.163478185457734));
#23446=CARTESIAN_POINT('Ctrl Pts',(-1.97406280235188,-1.,0.162079693556288));
#23447=CARTESIAN_POINT('Ctrl Pts',(-1.97996195437559,-1.,0.160622060784611));
#23448=CARTESIAN_POINT('Ctrl Pts',(-1.98584238283292,-1.,0.159106226437299));
#23449=CARTESIAN_POINT('Ctrl Pts',(-1.99169810931908,-1.,0.157533331459227));
#23450=CARTESIAN_POINT('Ctrl Pts',(-1.99753284771497,-1.,0.155904629548783));
#23451=CARTESIAN_POINT('Ctrl Pts',(-2.00335565310543,-1.,0.154221403049722));
#23452=CARTESIAN_POINT('Ctrl Pts',(-2.00917680318424,-1.,0.15248488362145));
#23453=CARTESIAN_POINT('Ctrl Pts',(-2.01500291940238,-1.,0.150696157673078));
#23454=CARTESIAN_POINT('Ctrl Pts',(-2.02083464969894,-1.,0.148856124775337));
#23455=CARTESIAN_POINT('Ctrl Pts',(-2.02666926182017,-1.,0.146965557332583));
#23456=CARTESIAN_POINT('Ctrl Pts',(-2.03250223739942,-1.,0.145025140186057));
#23457=CARTESIAN_POINT('Ctrl Pts',(-2.03832911025912,-1.,0.143035515058209));
#23458=CARTESIAN_POINT('Ctrl Pts',(-2.04414757947916,-1.,0.140997332152546));
#23459=CARTESIAN_POINT('Ctrl Pts',(-2.04995762001328,-1.,0.138911255368966));
#23460=CARTESIAN_POINT('Ctrl Pts',(-2.05576044414264,-1.,0.136777941218043));
#23461=CARTESIAN_POINT('Ctrl Pts',(-2.06155781517842,-1.,0.134598026192106));
#23462=CARTESIAN_POINT('Ctrl Pts',(-2.06735123910326,-1.,0.13237211154771));
#23463=CARTESIAN_POINT('Ctrl Pts',(-2.07314114713063,-1.,0.130100748328403));
#23464=CARTESIAN_POINT('Ctrl Pts',(-2.07892715110987,-1.,0.12778444527612));
#23465=CARTESIAN_POINT('Ctrl Pts',(-2.08470840653643,-1.,0.125423679412061));
#23466=CARTESIAN_POINT('Ctrl Pts',(-2.09048392424825,-1.,0.123018905621083));
#23467=CARTESIAN_POINT('Ctrl Pts',(-2.0962529286773,-1.,0.120570567965122));
#23468=CARTESIAN_POINT('Ctrl Pts',(-2.102015121329,-1.,0.118079107988355));
#23469=CARTESIAN_POINT('Ctrl Pts',(-2.10777050261309,-1.,0.115544957687926));
#23470=CARTESIAN_POINT('Ctrl Pts',(-2.11351924490306,-1.,0.112968534419737));
#23471=CARTESIAN_POINT('Ctrl Pts',(-2.11926155590865,-1.,0.110350236135025));
#23472=CARTESIAN_POINT('Ctrl Pts',(-2.12499752307,-1.,0.10769043523109));
#23473=CARTESIAN_POINT('Ctrl Pts',(-2.13072704887293,-1.,0.104989479152739));
#23474=CARTESIAN_POINT('Ctrl Pts',(-2.13644992667165,-1.,0.1022477005561));
#23475=CARTESIAN_POINT('Ctrl Pts',(-2.14216588396025,-1.,0.0994654261990914));
#23476=CARTESIAN_POINT('Ctrl Pts',(-2.14787463531795,-1.,0.0966429852305457));
#23477=CARTESIAN_POINT('Ctrl Pts',(-2.1535759397817,-1.,0.0937807218867642));
#23478=CARTESIAN_POINT('Ctrl Pts',(-2.15926961544516,-1.,0.0908789888107264));
#23479=CARTESIAN_POINT('Ctrl Pts',(-2.16495552645014,-1.,0.0879381291386921));
#23480=CARTESIAN_POINT('Ctrl Pts',(-2.17063357870952,-1.,0.0849584620835371));
#23481=CARTESIAN_POINT('Ctrl Pts',(-2.176303712113,-1.,0.0819402680872764));
#23482=CARTESIAN_POINT('Ctrl Pts',(-2.18196589448887,-1.,0.0788837727685241));
#23483=CARTESIAN_POINT('Ctrl Pts',(-2.1876201139953,-1.,0.0757891465836146));
#23484=CARTESIAN_POINT('Ctrl Pts',(-2.19213712013662,-1.,0.0732830357306724));
#23485=CARTESIAN_POINT('Ctrl Pts',(-2.19552129484002,-1.,0.0713863779526153));
#23486=CARTESIAN_POINT('Ctrl Pts',(-2.19777582085423,-1.,0.0701143536325489));
#23487=CARTESIAN_POINT('Ctrl Pts',(-2.19890268624765,-1.,0.069476445021958));
#23488=CARTESIAN_POINT('',(-2.19890268624765,-1.,-0.0694764450219585));
#23489=CARTESIAN_POINT('',(-2.19890268624765,-1.,0.069476445021958));
#23490=CARTESIAN_POINT('',(-1.74236521665491,-1.,-0.163289472382896));
#23491=CARTESIAN_POINT('Ctrl Pts',(-2.19890268624765,-1.,-0.0694764450219585));
#23492=CARTESIAN_POINT('Ctrl Pts',(-2.19777582085261,-1.,-0.0701143536324927));
#23493=CARTESIAN_POINT('Ctrl Pts',(-2.19552129483562,-1.,-0.0713863779524629));
#23494=CARTESIAN_POINT('Ctrl Pts',(-2.19213712012956,-1.,-0.0732830357304277));
#23495=CARTESIAN_POINT('Ctrl Pts',(-2.1876201139874,-1.,-0.0757891465833413));
#23496=CARTESIAN_POINT('Ctrl Pts',(-2.18196589448304,-1.,-0.0788837727683229));
#23497=CARTESIAN_POINT('Ctrl Pts',(-2.1763037121106,-1.,-0.0819402680871941));
#23498=CARTESIAN_POINT('Ctrl Pts',(-2.17063357871031,-1.,-0.0849584620835644));
#23499=CARTESIAN_POINT('Ctrl Pts',(-2.16495552645275,-1.,-0.0879381291387824));
#23500=CARTESIAN_POINT('Ctrl Pts',(-2.15926961544808,-1.,-0.0908789888108267));
#23501=CARTESIAN_POINT('Ctrl Pts',(-2.15357593978377,-1.,-0.0937807218868346));
#23502=CARTESIAN_POINT('Ctrl Pts',(-2.14787463531864,-1.,-0.096642985230569));
#23503=CARTESIAN_POINT('Ctrl Pts',(-2.14216588395974,-1.,-0.0994654261990744));
#23504=CARTESIAN_POINT('Ctrl Pts',(-2.13644992667052,-1.,-0.102247700556064));
#23505=CARTESIAN_POINT('Ctrl Pts',(-2.1307270488718,-1.,-0.104989479152703));
#23506=CARTESIAN_POINT('Ctrl Pts',(-2.12499752306927,-1.,-0.107690435231068));
#23507=CARTESIAN_POINT('Ctrl Pts',(-2.11926155590849,-1.,-0.11035023613502));
#23508=CARTESIAN_POINT('Ctrl Pts',(-2.11351924490335,-1.,-0.112968534419746));
#23509=CARTESIAN_POINT('Ctrl Pts',(-2.10777050261359,-1.,-0.11554495768794));
#23510=CARTESIAN_POINT('Ctrl Pts',(-2.10201512132945,-1.,-0.118079107988368));
#23511=CARTESIAN_POINT('Ctrl Pts',(-2.09625292867756,-1.,-0.120570567965129));
#23512=CARTESIAN_POINT('Ctrl Pts',(-2.09048392424826,-1.,-0.123018905621083));
#23513=CARTESIAN_POINT('Ctrl Pts',(-2.08470840653628,-1.,-0.125423679412058));
#23514=CARTESIAN_POINT('Ctrl Pts',(-2.07892715110967,-1.,-0.127784445276116));
#23515=CARTESIAN_POINT('Ctrl Pts',(-2.07314114713047,-1.,-0.130100748328401));
#23516=CARTESIAN_POINT('Ctrl Pts',(-2.06735123910319,-1.,-0.13237211154771));
#23517=CARTESIAN_POINT('Ctrl Pts',(-2.06155781517844,-1.,-0.134598026192107));
#23518=CARTESIAN_POINT('Ctrl Pts',(-2.0557604441427,-1.,-0.136777941218044));
#23519=CARTESIAN_POINT('Ctrl Pts',(-2.04995762001333,-1.,-0.138911255368966));
#23520=CARTESIAN_POINT('Ctrl Pts',(-2.04414757947919,-1.,-0.140997332152545));
#23521=CARTESIAN_POINT('Ctrl Pts',(-2.03832911025913,-1.,-0.143035515058208));
#23522=CARTESIAN_POINT('Ctrl Pts',(-2.03250223739941,-1.,-0.145025140186058));
#23523=CARTESIAN_POINT('Ctrl Pts',(-2.02666926182017,-1.,-0.146965557332586));
#23524=CARTESIAN_POINT('Ctrl Pts',(-2.02083464969897,-1.,-0.148856124775343));
#23525=CARTESIAN_POINT('Ctrl Pts',(-2.01500291940243,-1.,-0.150696157673084));
#23526=CARTESIAN_POINT('Ctrl Pts',(-2.00917680318426,-1.,-0.152484883621452));
#23527=CARTESIAN_POINT('Ctrl Pts',(-2.00335565310539,-1.,-0.154221403049719));
#23528=CARTESIAN_POINT('Ctrl Pts',(-1.99753284771487,-1.,-0.155904629548775));
#23529=CARTESIAN_POINT('Ctrl Pts',(-1.99169810931893,-1.,-0.157533331459215));
#23530=CARTESIAN_POINT('Ctrl Pts',(-1.98584238283279,-1.,-0.159106226437289));
#23531=CARTESIAN_POINT('Ctrl Pts',(-1.97996195437557,-1.,-0.16062206078461));
#23532=CARTESIAN_POINT('Ctrl Pts',(-1.97406280235204,-1.,-0.162079693556302));
#23533=CARTESIAN_POINT('Ctrl Pts',(-1.96816512678,-1.,-0.16347818545776));
#23534=CARTESIAN_POINT('Ctrl Pts',(-1.96229379940174,-1.,-0.1648165689203));
#23535=CARTESIAN_POINT('Ctrl Pts',(-1.95646759718755,-1.,-0.166093592002833));
#23536=CARTESIAN_POINT('Ctrl Pts',(-1.95069027794286,-1.,-0.167307501784469));
#23537=CARTESIAN_POINT('Ctrl Pts',(-1.94493757756879,-1.,-0.168455741607516));
#23538=CARTESIAN_POINT('Ctrl Pts',(-1.93915639211497,-1.,-0.169534904817425));
#23539=CARTESIAN_POINT('Ctrl Pts',(-1.93329183155455,-1.,-0.170541253116136));
#23540=CARTESIAN_POINT('Ctrl Pts',(-1.92731093582,-1.,-0.17147119153296));
#23541=CARTESIAN_POINT('Ctrl Pts',(-1.92122334398034,-1.,-0.172321621259557));
#23542=CARTESIAN_POINT('Ctrl Pts',(-1.91511429159681,-1.,-0.173090695383619));
#23543=CARTESIAN_POINT('Ctrl Pts',(-1.90911693975475,-1.,-0.173776635257984));
#23544=CARTESIAN_POINT('Ctrl Pts',(-1.90335253863003,-1.,-0.174375518661222));
#23545=CARTESIAN_POINT('Ctrl Pts',(-1.89788101117148,-1.,-0.174879405091277));
#23546=CARTESIAN_POINT('Ctrl Pts',(-1.89264630198279,-1.,-0.175274276190664));
#23547=CARTESIAN_POINT('Ctrl Pts',(-1.88742606272818,-1.,-0.175538155840286));
#23548=CARTESIAN_POINT('Ctrl Pts',(-1.88188663144846,-1.,-0.175644148889271));
#23549=CARTESIAN_POINT('Ctrl Pts',(-1.87563767773249,-1.,-0.175563480746205));
#23550=CARTESIAN_POINT('Ctrl Pts',(-1.86828349694972,-1.,-0.175268337590901));
#23551=CARTESIAN_POINT('Ctrl Pts',(-1.85948367089838,-1.,-0.174735259276856));
#23552=CARTESIAN_POINT('Ctrl Pts',(-1.84898113200543,-1.,-0.173946627589401));
#23553=CARTESIAN_POINT('Ctrl Pts',(-1.83658380530747,-1.,-0.17288944289442));
#23554=CARTESIAN_POINT('Ctrl Pts',(-1.82215766815414,-1.,-0.171554770207306));
#23555=CARTESIAN_POINT('Ctrl Pts',(-1.80561530633924,-1.,-0.169936923908078));
#23556=CARTESIAN_POINT('Ctrl Pts',(-1.78690649988931,-1.,-0.16803277280837));
#23557=CARTESIAN_POINT('Ctrl Pts',(-1.77018771687692,-1.,-0.166279355148738));
#23558=CARTESIAN_POINT('Ctrl Pts',(-1.75666056640041,-1.,-0.164834765708484));
#23559=CARTESIAN_POINT('Ctrl Pts',(-1.74720349503904,-1.,-0.163814161002474));
#23560=CARTESIAN_POINT('Ctrl Pts',(-1.74236521665491,-1.,-0.163289472382896));
#23561=CARTESIAN_POINT('',(-1.7075470150345,-1.,-0.383122945602004));
#23562=CARTESIAN_POINT('Origin',(0.,-1.,0.));
#23563=CARTESIAN_POINT('',(-2.11275013067528,-1.,-0.61342227326009));
#23564=CARTESIAN_POINT('Ctrl Pts',(-1.7075470150345,-1.,-0.383122945602004));
#23565=CARTESIAN_POINT('Ctrl Pts',(-1.71231062891398,-1.,-0.384119047314215));
#23566=CARTESIAN_POINT('Ctrl Pts',(-1.72162022244582,-1.,-0.386070790323281));
#23567=CARTESIAN_POINT('Ctrl Pts',(-1.73493170972829,-1.,-0.388877023502615));
#23568=CARTESIAN_POINT('Ctrl Pts',(-1.75137405310193,-1.,-0.392375812285395));
#23569=CARTESIAN_POINT('Ctrl Pts',(-1.76975560043442,-1.,-0.396346196110688));
#23570=CARTESIAN_POINT('Ctrl Pts',(-1.78598826343754,-1.,-0.399919403774155));
#23571=CARTESIAN_POINT('Ctrl Pts',(-1.80012077173238,-1.,-0.403107976163396));
#23572=CARTESIAN_POINT('Ctrl Pts',(-1.81223801812013,-1.,-0.405933518407175));
#23573=CARTESIAN_POINT('Ctrl Pts',(-1.82247022677562,-1.,-0.408428948106227));
#23574=CARTESIAN_POINT('Ctrl Pts',(-1.83100408895047,-1.,-0.410641256301276));
#23575=CARTESIAN_POINT('Ctrl Pts',(-1.8380895347617,-1.,-0.412633125322945));
#23576=CARTESIAN_POINT('Ctrl Pts',(-1.84405757074218,-1.,-0.414487438255542));
#23577=CARTESIAN_POINT('Ctrl Pts',(-1.84929312930314,-1.,-0.416300022039885));
#23578=CARTESIAN_POINT('Ctrl Pts',(-1.8541763285645,-1.,-0.418164129144045));
#23579=CARTESIAN_POINT('Ctrl Pts',(-1.8590328109667,-1.,-0.420157287975583));
#23580=CARTESIAN_POINT('Ctrl Pts',(-1.86408083333863,-1.,-0.422327307417884));
#23581=CARTESIAN_POINT('Ctrl Pts',(-1.8693780394412,-1.,-0.424678177290876));
#23582=CARTESIAN_POINT('Ctrl Pts',(-1.87486989291333,-1.,-0.427183828518743));
#23583=CARTESIAN_POINT('Ctrl Pts',(-1.88044229001778,-1.,-0.429803062482217));
#23584=CARTESIAN_POINT('Ctrl Pts',(-1.88596913666828,-1.,-0.432493038548833));
#23585=CARTESIAN_POINT('Ctrl Pts',(-1.89136993975585,-1.,-0.43522566096358));
#23586=CARTESIAN_POINT('Ctrl Pts',(-1.89663648956549,-1.,-0.437995003948443));
#23587=CARTESIAN_POINT('Ctrl Pts',(-1.90180124389137,-1.,-0.44080783370416));
#23588=CARTESIAN_POINT('Ctrl Pts',(-1.90691756144906,-1.,-0.44367755684917));
#23589=CARTESIAN_POINT('Ctrl Pts',(-1.91203699981095,-1.,-0.446617343485651));
#23590=CARTESIAN_POINT('Ctrl Pts',(-1.91718342555717,-1.,-0.449632260106572));
#23591=CARTESIAN_POINT('Ctrl Pts',(-1.9223538064847,-1.,-0.452719478359356));
#23592=CARTESIAN_POINT('Ctrl Pts',(-1.92753067150461,-1.,-0.455872005174335));
#23593=CARTESIAN_POINT('Ctrl Pts',(-1.93269066517936,-1.,-0.459081234547931));
#23594=CARTESIAN_POINT('Ctrl Pts',(-1.93781486640834,-1.,-0.462340031009087));
#23595=CARTESIAN_POINT('Ctrl Pts',(-1.94289794196205,-1.,-0.465645462026064));
#23596=CARTESIAN_POINT('Ctrl Pts',(-1.94794381136524,-1.,-0.468997482913158));
#23597=CARTESIAN_POINT('Ctrl Pts',(-1.95296148278136,-1.,-0.472397672264079));
#23598=CARTESIAN_POINT('Ctrl Pts',(-1.95796111148175,-1.,-0.475848034683171));
#23599=CARTESIAN_POINT('Ctrl Pts',(-1.96294933055938,-1.,-0.479349583074846));
#23600=CARTESIAN_POINT('Ctrl Pts',(-1.96792703422358,-1.,-0.482901662120686));
#23601=CARTESIAN_POINT('Ctrl Pts',(-1.97289186263272,-1.,-0.486502692907661));
#23602=CARTESIAN_POINT('Ctrl Pts',(-1.97783973019229,-1.,-0.490150627860955));
#23603=CARTESIAN_POINT('Ctrl Pts',(-1.9827665876182,-1.,-0.493843476541492));
#23604=CARTESIAN_POINT('Ctrl Pts',(-1.98767044752929,-1.,-0.497579909545564));
#23605=CARTESIAN_POINT('Ctrl Pts',(-1.9925514912615,-1.,-0.501359287727129));
#23606=CARTESIAN_POINT('Ctrl Pts',(-1.99741107463567,-1.,-0.505181361323011));
#23607=CARTESIAN_POINT('Ctrl Pts',(-2.00225107134733,-1.,-0.509046069886152));
#23608=CARTESIAN_POINT('Ctrl Pts',(-2.00707309946955,-1.,-0.512953306961813));
#23609=CARTESIAN_POINT('Ctrl Pts',(-2.01187773939257,-1.,-0.516902681728733));
#23610=CARTESIAN_POINT('Ctrl Pts',(-2.01666477917305,-1.,-0.520893590399428));
#23611=CARTESIAN_POINT('Ctrl Pts',(-2.02143356304712,-1.,-0.524925318333518));
#23612=CARTESIAN_POINT('Ctrl Pts',(-2.02618329083289,-1.,-0.52899712724191));
#23613=CARTESIAN_POINT('Ctrl Pts',(-2.03091336214401,-1.,-0.533108355132905));
#23614=CARTESIAN_POINT('Ctrl Pts',(-2.03562362953993,-1.,-0.537258489833134));
#23615=CARTESIAN_POINT('Ctrl Pts',(-2.0403142269048,-1.,-0.54144712061552));
#23616=CARTESIAN_POINT('Ctrl Pts',(-2.0449854471456,-1.,-0.545673903817348));
#23617=CARTESIAN_POINT('Ctrl Pts',(-2.04963761077974,-1.,-0.549938525150342));
#23618=CARTESIAN_POINT('Ctrl Pts',(-2.05427091604482,-1.,-0.554240657464109));
#23619=CARTESIAN_POINT('Ctrl Pts',(-2.05888537756571,-1.,-0.558579940185467));
#23620=CARTESIAN_POINT('Ctrl Pts',(-2.06348090160697,-1.,-0.562955993082574));
#23621=CARTESIAN_POINT('Ctrl Pts',(-2.06805732997383,-1.,-0.567368421181229));
#23622=CARTESIAN_POINT('Ctrl Pts',(-2.07261449292757,-1.,-0.571816823242411));
#23623=CARTESIAN_POINT('Ctrl Pts',(-2.07715226767361,-1.,-0.576300797416274));
#23624=CARTESIAN_POINT('Ctrl Pts',(-2.08167059018138,-1.,-0.580819952107257));
#23625=CARTESIAN_POINT('Ctrl Pts',(-2.086169437277,-1.,-0.585373918990895));
#23626=CARTESIAN_POINT('Ctrl Pts',(-2.09064881812053,-1.,-0.589962365403189));
#23627=CARTESIAN_POINT('Ctrl Pts',(-2.09510876220501,-1.,-0.594585006052823));
#23628=CARTESIAN_POINT('Ctrl Pts',(-2.09954930865331,-1.,-0.599241616422144));
#23629=CARTESIAN_POINT('Ctrl Pts',(-2.10397049887709,-1.,-0.603932030738212));
#23630=CARTESIAN_POINT('Ctrl Pts',(-2.10749199615859,-1.,-0.607711315456826));
#23631=CARTESIAN_POINT('Ctrl Pts',(-2.11012443807661,-1.,-0.610560911691113));
#23632=CARTESIAN_POINT('Ctrl Pts',(-2.11187554260142,-1.,-0.61246736556225));
#23633=CARTESIAN_POINT('Ctrl Pts',(-2.11275013067528,-1.,-0.61342227326009));
#23634=CARTESIAN_POINT('',(-2.0698113262342,-1.,-0.745574324794401));
#23635=CARTESIAN_POINT('',(-2.11275013067528,-1.,-0.61342227326009));
#23636=CARTESIAN_POINT('',(-1.60662857109684,-1.,-0.693717979106306));
#23637=CARTESIAN_POINT('Ctrl Pts',(-2.0698113262342,-1.,-0.745574324794401));
#23638=CARTESIAN_POINT('Ctrl Pts',(-2.06854248895575,-1.,-0.74583279137781));
#23639=CARTESIAN_POINT('Ctrl Pts',(-2.06600523016401,-1.,-0.746345871542695));
#23640=CARTESIAN_POINT('Ctrl Pts',(-2.06220058927162,-1.,-0.747103932785504));
#23641=CARTESIAN_POINT('Ctrl Pts',(-2.05713023030263,-1.,-0.748091554181101));
#23642=CARTESIAN_POINT('Ctrl Pts',(-2.05079645591606,-1.,-0.749287468663053));
#23643=CARTESIAN_POINT('Ctrl Pts',(-2.04446689147754,-1.,-0.750444657874758));
#23644=CARTESIAN_POINT('Ctrl Pts',(-2.03814160092173,-1.,-0.751562963361383));
#23645=CARTESIAN_POINT('Ctrl Pts',(-2.03182068456467,-1.,-0.752642180488104));
#23646=CARTESIAN_POINT('Ctrl Pts',(-2.02550428623587,-1.,-0.753682061113765));
#23647=CARTESIAN_POINT('Ctrl Pts',(-2.01919259406003,-1.,-0.75468233072352));
#23648=CARTESIAN_POINT('Ctrl Pts',(-2.01288584328149,-1.,-0.7556427049581));
#23649=CARTESIAN_POINT('Ctrl Pts',(-2.00658431587682,-1.,-0.756562904646496));
#23650=CARTESIAN_POINT('Ctrl Pts',(-2.00028834739072,-1.,-0.757442676862341));
#23651=CARTESIAN_POINT('Ctrl Pts',(-1.9939983109871,-1.,-0.758281796766377));
#23652=CARTESIAN_POINT('Ctrl Pts',(-1.98771456680806,-1.,-0.759080037802242));
#23653=CARTESIAN_POINT('Ctrl Pts',(-1.98143741418156,-1.,-0.759837147452135));
#23654=CARTESIAN_POINT('Ctrl Pts',(-1.97516705321521,-1.,-0.760552825409855));
#23655=CARTESIAN_POINT('Ctrl Pts',(-1.96890351582545,-1.,-0.761226690483986));
#23656=CARTESIAN_POINT('Ctrl Pts',(-1.96264672744229,-1.,-0.761858300014575));
#23657=CARTESIAN_POINT('Ctrl Pts',(-1.95639665309893,-1.,-0.762447203806263));
#23658=CARTESIAN_POINT('Ctrl Pts',(-1.95015342590025,-1.,-0.762992990878774));
#23659=CARTESIAN_POINT('Ctrl Pts',(-1.94391746617626,-1.,-0.76349533353858));
#23660=CARTESIAN_POINT('Ctrl Pts',(-1.93768964875867,-1.,-0.763954049121393));
#23661=CARTESIAN_POINT('Ctrl Pts',(-1.93147105496367,-1.,-0.764369010673889));
#23662=CARTESIAN_POINT('Ctrl Pts',(-1.92526263537041,-1.,-0.764740025488189));
#23663=CARTESIAN_POINT('Ctrl Pts',(-1.91906491634197,-1.,-0.765066729667095));
#23664=CARTESIAN_POINT('Ctrl Pts',(-1.91287765805174,-1.,-0.765348465884739));
#23665=CARTESIAN_POINT('Ctrl Pts',(-1.90669961402362,-1.,-0.765584196937936));
#23666=CARTESIAN_POINT('Ctrl Pts',(-1.90052930393599,-1.,-0.765772772593395));
#23667=CARTESIAN_POINT('Ctrl Pts',(-1.89436577771389,-1.,-0.765913193856979));
#23668=CARTESIAN_POINT('Ctrl Pts',(-1.88820926433409,-1.,-0.76600483706209));
#23669=CARTESIAN_POINT('Ctrl Pts',(-1.88206215302561,-1.,-0.766047794851868));
#23670=CARTESIAN_POINT('Ctrl Pts',(-1.87592888967886,-1.,-0.766042837036759));
#23671=CARTESIAN_POINT('Ctrl Pts',(-1.86981398314345,-1.,-0.765990708546111));
#23672=CARTESIAN_POINT('Ctrl Pts',(-1.86372027063314,-1.,-0.765891519092557));
#23673=CARTESIAN_POINT('Ctrl Pts',(-1.85764741390391,-1.,-0.765744212909305));
#23674=CARTESIAN_POINT('Ctrl Pts',(-1.85158945130054,-1.,-0.765545710619023));
#23675=CARTESIAN_POINT('Ctrl Pts',(-1.8455369887591,-1.,-0.765291664861971));
#23676=CARTESIAN_POINT('Ctrl Pts',(-1.83948181064823,-1.,-0.764978057881687));
#23677=CARTESIAN_POINT('Ctrl Pts',(-1.8334207722714,-1.,-0.764602549687845));
#23678=CARTESIAN_POINT('Ctrl Pts',(-1.8273599120008,-1.,-0.764165902606055));
#23679=CARTESIAN_POINT('Ctrl Pts',(-1.82131873145297,-1.,-0.763673465462854));
#23680=CARTESIAN_POINT('Ctrl Pts',(-1.81532118405566,-1.,-0.763132003836783));
#23681=CARTESIAN_POINT('Ctrl Pts',(-1.80938551463989,-1.,-0.762546129464036));
#23682=CARTESIAN_POINT('Ctrl Pts',(-1.80351583877334,-1.,-0.761915336443515));
#23683=CARTESIAN_POINT('Ctrl Pts',(-1.79768986997735,-1.,-0.761229695230359));
#23684=CARTESIAN_POINT('Ctrl Pts',(-1.79185815610802,-1.,-0.760469555880425));
#23685=CARTESIAN_POINT('Ctrl Pts',(-1.78596964884526,-1.,-0.759614401109868));
#23686=CARTESIAN_POINT('Ctrl Pts',(-1.77999411220912,-1.,-0.75865062667738));
#23687=CARTESIAN_POINT('Ctrl Pts',(-1.77394167108342,-1.,-0.757578264077238));
#23688=CARTESIAN_POINT('Ctrl Pts',(-1.76789396003141,-1.,-0.756421896028403));
#23689=CARTESIAN_POINT('Ctrl Pts',(-1.7619781724032,-1.,-0.755220979975262));
#23690=CARTESIAN_POINT('Ctrl Pts',(-1.75631083600175,-1.,-0.75400925402848));
#23691=CARTESIAN_POINT('Ctrl Pts',(-1.75095139468809,-1.,-0.752797683531377));
#23692=CARTESIAN_POINT('Ctrl Pts',(-1.74585086852298,-1.,-0.751555614163629));
#23693=CARTESIAN_POINT('Ctrl Pts',(-1.74080458266705,-1.,-0.75019343597954));
#23694=CARTESIAN_POINT('Ctrl Pts',(-1.73550351679848,-1.,-0.748582462954854));
#23695=CARTESIAN_POINT('Ctrl Pts',(-1.72958533647399,-1.,-0.746574710096436));
#23696=CARTESIAN_POINT('Ctrl Pts',(-1.7226822991693,-1.,-0.744021445433764));
#23697=CARTESIAN_POINT('Ctrl Pts',(-1.71447789751927,-1.,-0.740795162032087));
#23698=CARTESIAN_POINT('Ctrl Pts',(-1.70473309006121,-1.,-0.736799665724771));
#23699=CARTESIAN_POINT('Ctrl Pts',(-1.69326921975743,-1.,-0.731963238697195));
#23700=CARTESIAN_POINT('Ctrl Pts',(-1.67996158455503,-1.,-0.726235967997433));
#23701=CARTESIAN_POINT('Ctrl Pts',(-1.6647288055568,-1.,-0.719585433804282));
#23702=CARTESIAN_POINT('Ctrl Pts',(-1.64752408832016,-1.,-0.711993139355394));
#23703=CARTESIAN_POINT('Ctrl Pts',(-1.63216541664676,-1.,-0.705159151988319));
#23704=CARTESIAN_POINT('Ctrl Pts',(-1.61974673472612,-1.,-0.699605146405088));
#23705=CARTESIAN_POINT('Ctrl Pts',(-1.61106790958151,-1.,-0.695712097881194));
#23706=CARTESIAN_POINT('Ctrl Pts',(-1.60662857109684,-1.,-0.693717979106306));
#23707=CARTESIAN_POINT('',(-1.5055822144029,-1.,-0.892032620296855));
#23708=CARTESIAN_POINT('Origin',(0.,-1.,0.));
#23709=CARTESIAN_POINT('',(-1.81978687191668,-1.,-1.23627494547115));
#23710=CARTESIAN_POINT('Ctrl Pts',(-1.5055822144029,-1.,-0.892032620296855));
#23711=CARTESIAN_POINT('Ctrl Pts',(-1.50980486806688,-1.,-0.894452006964543));
#23712=CARTESIAN_POINT('Ctrl Pts',(-1.51805569590094,-1.,-0.899185047483511));
#23713=CARTESIAN_POINT('Ctrl Pts',(-1.52984849887993,-1.,-0.905967409625651));
#23714=CARTESIAN_POINT('Ctrl Pts',(-1.54440491149498,-1.,-0.914375919026456));
#23715=CARTESIAN_POINT('Ctrl Pts',(-1.56065988578893,-1.,-0.923832188944341));
#23716=CARTESIAN_POINT('Ctrl Pts',(-1.57499388382243,-1.,-0.932246680108685));
#23717=CARTESIAN_POINT('Ctrl Pts',(-1.58744937487176,-1.,-0.939646377893399));
#23718=CARTESIAN_POINT('Ctrl Pts',(-1.59810042043673,-1.,-0.946078063315257));
#23719=CARTESIAN_POINT('Ctrl Pts',(-1.60706069896936,-1.,-0.951613284356035));
#23720=CARTESIAN_POINT('Ctrl Pts',(-1.61449324337085,-1.,-0.956354422920671));
#23721=CARTESIAN_POINT('Ctrl Pts',(-1.62061638140221,-1.,-0.960438326101729));
#23722=CARTESIAN_POINT('Ctrl Pts',(-1.62571930670187,-1.,-0.964046107040536));
#23723=CARTESIAN_POINT('Ctrl Pts',(-1.63013849959461,-1.,-0.967387853230345));
#23724=CARTESIAN_POINT('Ctrl Pts',(-1.63420665729798,-1.,-0.970669715997509));
#23725=CARTESIAN_POINT('Ctrl Pts',(-1.63820952658144,-1.,-0.974066058287418));
#23726=CARTESIAN_POINT('Ctrl Pts',(-1.64233990826687,-1.,-0.977689794119416));
#23727=CARTESIAN_POINT('Ctrl Pts',(-1.64665139190656,-1.,-0.981562530939489));
#23728=CARTESIAN_POINT('Ctrl Pts',(-1.65110016612638,-1.,-0.985642622920821));
#23729=CARTESIAN_POINT('Ctrl Pts',(-1.65559044289699,-1.,-0.989855627854165));
#23730=CARTESIAN_POINT('Ctrl Pts',(-1.66001553809947,-1.,-0.994121836661306));
#23731=CARTESIAN_POINT('Ctrl Pts',(-1.66430758030376,-1.,-0.998389654952758));
#23732=CARTESIAN_POINT('Ctrl Pts',(-1.66846059277303,-1.,-1.00265091003727));
#23733=CARTESIAN_POINT('Ctrl Pts',(-1.67250335383293,-1.,-1.00692206696414));
#23734=CARTESIAN_POINT('Ctrl Pts',(-1.67648246776464,-1.,-1.01123236493511));
#23735=CARTESIAN_POINT('Ctrl Pts',(-1.68044289894798,-1.,-1.01561026162773));
#23736=CARTESIAN_POINT('Ctrl Pts',(-1.68440578021706,-1.,-1.02006795074201));
#23737=CARTESIAN_POINT('Ctrl Pts',(-1.68836910178447,-1.,-1.02460180535255));
#23738=CARTESIAN_POINT('Ctrl Pts',(-1.69231840863458,-1.,-1.02919977579147));
#23739=CARTESIAN_POINT('Ctrl Pts',(-1.69623414782771,-1.,-1.03384646003588));
#23740=CARTESIAN_POINT('Ctrl Pts',(-1.70010052930962,-1.,-1.03852922490789));
#23741=CARTESIAN_POINT('Ctrl Pts',(-1.70391338707982,-1.,-1.04324363334554));
#23742=CARTESIAN_POINT('Ctrl Pts',(-1.70767646263649,-1.,-1.04799085404995));
#23743=CARTESIAN_POINT('Ctrl Pts',(-1.71139783543989,-1.,-1.05277517202855));
#23744=CARTESIAN_POINT('Ctrl Pts',(-1.7150865442702,-1.,-1.05760163192479));
#23745=CARTESIAN_POINT('Ctrl Pts',(-1.71874858456904,-1.,-1.06247324680647));
#23746=CARTESIAN_POINT('Ctrl Pts',(-1.72238500928453,-1.,-1.06738966975462));
#23747=CARTESIAN_POINT('Ctrl Pts',(-1.72599406198488,-1.,-1.07234866990252));
#23748=CARTESIAN_POINT('Ctrl Pts',(-1.72957248977424,-1.,-1.0773470373727));
#23749=CARTESIAN_POINT('Ctrl Pts',(-1.73311705663407,-1.,-1.08238162784749));
#23750=CARTESIAN_POINT('Ctrl Pts',(-1.73662628326091,-1.,-1.08745056285427));
#23751=CARTESIAN_POINT('Ctrl Pts',(-1.74010053962247,-1.,-1.09255329056493));
#23752=CARTESIAN_POINT('Ctrl Pts',(-1.74354119236208,-1.,-1.09768999241225));
#23753=CARTESIAN_POINT('Ctrl Pts',(-1.74695004214923,-1.,-1.10286118991143));
#23754=CARTESIAN_POINT('Ctrl Pts',(-1.7503286607592,-1.,-1.10806728183007));
#23755=CARTESIAN_POINT('Ctrl Pts',(-1.7536777209463,-1.,-1.11330807582551));
#23756=CARTESIAN_POINT('Ctrl Pts',(-1.75699720772105,-1.,-1.11858293216763));
#23757=CARTESIAN_POINT('Ctrl Pts',(-1.76028671825096,-1.,-1.12389096855086));
#23758=CARTESIAN_POINT('Ctrl Pts',(-1.7635457196617,-1.,-1.12923123555075));
#23759=CARTESIAN_POINT('Ctrl Pts',(-1.76677384551862,-1.,-1.1346029180462));
#23760=CARTESIAN_POINT('Ctrl Pts',(-1.76997111386769,-1.,-1.14000548336975));
#23761=CARTESIAN_POINT('Ctrl Pts',(-1.77313777896194,-1.,-1.1454385822692));
#23762=CARTESIAN_POINT('Ctrl Pts',(-1.7762742255701,-1.,-1.15090197841515));
#23763=CARTESIAN_POINT('Ctrl Pts',(-1.77938085564275,-1.,-1.15639547194698));
#23764=CARTESIAN_POINT('Ctrl Pts',(-1.78245795881009,-1.,-1.16191881298499));
#23765=CARTESIAN_POINT('Ctrl Pts',(-1.78550566040443,-1.,-1.16747166312303));
#23766=CARTESIAN_POINT('Ctrl Pts',(-1.78852398877616,-1.,-1.17305363177328));
#23767=CARTESIAN_POINT('Ctrl Pts',(-1.79151291552689,-1.,-1.17866429440809));
#23768=CARTESIAN_POINT('Ctrl Pts',(-1.79447240321515,-1.,-1.18430321697432));
#23769=CARTESIAN_POINT('Ctrl Pts',(-1.79740245923478,-1.,-1.18996997934445));
#23770=CARTESIAN_POINT('Ctrl Pts',(-1.80030314369879,-1.,-1.19566418930242));
#23771=CARTESIAN_POINT('Ctrl Pts',(-1.80317454838603,-1.,-1.20138548938974));
#23772=CARTESIAN_POINT('Ctrl Pts',(-1.80601678480707,-1.,-1.20713356605475));
#23773=CARTESIAN_POINT('Ctrl Pts',(-1.80882996917129,-1.,-1.21290815708314));
#23774=CARTESIAN_POINT('Ctrl Pts',(-1.81161420806656,-1.,-1.21870906103557));
#23775=CARTESIAN_POINT('Ctrl Pts',(-1.81436959210434,-1.,-1.2245361330495));
#23776=CARTESIAN_POINT('Ctrl Pts',(-1.8165508718364,-1.,-1.2292186489137));
#23777=CARTESIAN_POINT('Ctrl Pts',(-1.81817389921279,-1.,-1.2327422452705));
#23778=CARTESIAN_POINT('Ctrl Pts',(-1.81925017193666,-1.,-1.23509651170476));
#23779=CARTESIAN_POINT('Ctrl Pts',(-1.81978687191668,-1.,-1.23627494547115));
#23780=CARTESIAN_POINT('',(-1.73811241238545,-1.,-1.34869019493419));
#23781=CARTESIAN_POINT('',(-1.81978687191668,-1.,-1.23627494547115));
#23782=CARTESIAN_POINT('',(-1.31362392696032,-1.,-1.15624053661742));
#23783=CARTESIAN_POINT('Ctrl Pts',(-1.73811241238545,-1.,-1.34869019493419));
#23784=CARTESIAN_POINT('Ctrl Pts',(-1.73682580585691,-1.,-1.34854391898045));
#23785=CARTESIAN_POINT('Ctrl Pts',(-1.73425417885907,-1.,-1.34824783112887));
#23786=CARTESIAN_POINT('Ctrl Pts',(-1.7304014965394,-1.,-1.34779309152035));
#23787=CARTESIAN_POINT('Ctrl Pts',(-1.72527410680674,-1.,-1.34716554819527));
#23788=CARTESIAN_POINT('Ctrl Pts',(-1.7188807715049,-1.,-1.34634568653227));
#23789=CARTESIAN_POINT('Ctrl Pts',(-1.71250340686822,-1.,-1.34549029589416));
#23790=CARTESIAN_POINT('Ctrl Pts',(-1.70614212266738,-1.,-1.34459924533831));
#23791=CARTESIAN_POINT('Ctrl Pts',(-1.69979707754427,-1.,-1.34367237124483));
#23792=CARTESIAN_POINT('Ctrl Pts',(-1.6934684849687,-1.,-1.34270948206319));
#23793=CARTESIAN_POINT('Ctrl Pts',(-1.68715660868764,-1.,-1.341710374848));
#23794=CARTESIAN_POINT('Ctrl Pts',(-1.68086176030362,-1.,-1.34067485185203));
#23795=CARTESIAN_POINT('Ctrl Pts',(-1.67458429426086,-1.,-1.3396027347034));
#23796=CARTESIAN_POINT('Ctrl Pts',(-1.66832460783989,-1.,-1.33849388654388));
#23797=CARTESIAN_POINT('Ctrl Pts',(-1.66208312541983,-1.,-1.33734820885262));
#23798=CARTESIAN_POINT('Ctrl Pts',(-1.65586025952593,-1.,-1.33616559745172));
#23799=CARTESIAN_POINT('Ctrl Pts',(-1.6496563728683,-1.,-1.33494590467993));
#23800=CARTESIAN_POINT('Ctrl Pts',(-1.6434717485603,-1.,-1.33368890676572));
#23801=CARTESIAN_POINT('Ctrl Pts',(-1.63730653475089,-1.,-1.33239425103724));
#23802=CARTESIAN_POINT('Ctrl Pts',(-1.63116079730923,-1.,-1.33106149345645));
#23803=CARTESIAN_POINT('Ctrl Pts',(-1.62503464209797,-1.,-1.3296901950568));
#23804=CARTESIAN_POINT('Ctrl Pts',(-1.61892832270724,-1.,-1.32828000610449));
#23805=CARTESIAN_POINT('Ctrl Pts',(-1.6128423401575,-1.,-1.32683074483356));
#23806=CARTESIAN_POINT('Ctrl Pts',(-1.60677758290954,-1.,-1.32534250785782));
#23807=CARTESIAN_POINT('Ctrl Pts',(-1.60073511858687,-1.,-1.32381550858256));
#23808=CARTESIAN_POINT('Ctrl Pts',(-1.59471591079403,-1.,-1.32224985747682));
#23809=CARTESIAN_POINT('Ctrl Pts',(-1.58872057258245,-1.,-1.32064537110892));
#23810=CARTESIAN_POINT('Ctrl Pts',(-1.58274907898834,-1.,-1.31900135021432));
#23811=CARTESIAN_POINT('Ctrl Pts',(-1.5768005650559,-1.,-1.31731642317187));
#23812=CARTESIAN_POINT('Ctrl Pts',(-1.57087397835723,-1.,-1.31558903860016));
#23813=CARTESIAN_POINT('Ctrl Pts',(-1.56496872402353,-1.,-1.31381795281002));
#23814=CARTESIAN_POINT('Ctrl Pts',(-1.55908521254821,-1.,-1.31200264341696));
#23815=CARTESIAN_POINT('Ctrl Pts',(-1.55322568759481,-1.,-1.31014393684222));
#23816=CARTESIAN_POINT('Ctrl Pts',(-1.54739413957185,-1.,-1.30824393907473));
#23817=CARTESIAN_POINT('Ctrl Pts',(-1.54159462645432,-1.,-1.30630475189556));
#23818=CARTESIAN_POINT('Ctrl Pts',(-1.53582981268977,-1.,-1.30432735639489));
#23819=CARTESIAN_POINT('Ctrl Pts',(-1.53009970283891,-1.,-1.30231064395568));
#23820=CARTESIAN_POINT('Ctrl Pts',(-1.52439957861062,-1.,-1.30024984366328));
#23821=CARTESIAN_POINT('Ctrl Pts',(-1.51872184912724,-1.,-1.29813791800747));
#23822=CARTESIAN_POINT('Ctrl Pts',(-1.51305994241402,-1.,-1.29596850710509));
#23823=CARTESIAN_POINT('Ctrl Pts',(-1.50741159078365,-1.,-1.29373841372842));
#23824=CARTESIAN_POINT('Ctrl Pts',(-1.50178230149776,-1.,-1.29145022885181));
#23825=CARTESIAN_POINT('Ctrl Pts',(-1.49618896881754,-1.,-1.28911506584254));
#23826=CARTESIAN_POINT('Ctrl Pts',(-1.4906522831278,-1.,-1.2867467611644));
#23827=CARTESIAN_POINT('Ctrl Pts',(-1.4851881711891,-1.,-1.28435533880201));
#23828=CARTESIAN_POINT('Ctrl Pts',(-1.47980070347095,-1.,-1.28194158939517));
#23829=CARTESIAN_POINT('Ctrl Pts',(-1.4744717526707,-1.,-1.2794891824849));
#23830=CARTESIAN_POINT('Ctrl Pts',(-1.46916035917133,-1.,-1.27696414831089));
#23831=CARTESIAN_POINT('Ctrl Pts',(-1.46382431332476,-1.,-1.27433119897822));
#23832=CARTESIAN_POINT('Ctrl Pts',(-1.45843906294697,-1.,-1.27156805265289));
#23833=CARTESIAN_POINT('Ctrl Pts',(-1.45301422764247,-1.,-1.2686778680489));
#23834=CARTESIAN_POINT('Ctrl Pts',(-1.44761985001662,-1.,-1.26570925118868));
#23835=CARTESIAN_POINT('Ctrl Pts',(-1.44236470511303,-1.,-1.26273903323859));
#23836=CARTESIAN_POINT('Ctrl Pts',(-1.43734919180848,-1.,-1.25983531012005));
#23837=CARTESIAN_POINT('Ctrl Pts',(-1.43262645609691,-1.,-1.25702687965755));
#23838=CARTESIAN_POINT('Ctrl Pts',(-1.42815938799387,-1.,-1.25426945222639));
#23839=CARTESIAN_POINT('Ctrl Pts',(-1.42378102115575,-1.,-1.2514145557001));
#23840=CARTESIAN_POINT('Ctrl Pts',(-1.41923722596025,-1.,-1.24824430986571));
#23841=CARTESIAN_POINT('Ctrl Pts',(-1.41422913175179,-1.,-1.24450600513056));
#23842=CARTESIAN_POINT('Ctrl Pts',(-1.40845295531283,-1.,-1.23994455029534));
#23843=CARTESIAN_POINT('Ctrl Pts',(-1.40164708206106,-1.,-1.23434087290423));
#23844=CARTESIAN_POINT('Ctrl Pts',(-1.39361389568796,-1.,-1.22752961899387));
#23845=CARTESIAN_POINT('Ctrl Pts',(-1.38420564527715,-1.,-1.21938737280852));
#23846=CARTESIAN_POINT('Ctrl Pts',(-1.37331915607905,-1.,-1.20982812925645));
#23847=CARTESIAN_POINT('Ctrl Pts',(-1.36088705043885,-1.,-1.1987959077932));
#23848=CARTESIAN_POINT('Ctrl Pts',(-1.34687054001093,-1.,-1.18625865667441));
#23849=CARTESIAN_POINT('Ctrl Pts',(-1.33437539347008,-1.,-1.17501305789857));
#23850=CARTESIAN_POINT('Ctrl Pts',(-1.32428080721772,-1.,-1.16589330093588));
#23851=CARTESIAN_POINT('Ctrl Pts',(-1.31722977216397,-1.,-1.15950888730809));
#23852=CARTESIAN_POINT('Ctrl Pts',(-1.31362392696032,-1.,-1.15624053661742));
#23853=CARTESIAN_POINT('',(-1.15624053661742,-1.,-1.31362392696033));
#23854=CARTESIAN_POINT('Origin',(0.,-1.,0.));
#23855=CARTESIAN_POINT('',(-1.34869019493419,-1.,-1.73811241238545));
#23856=CARTESIAN_POINT('Ctrl Pts',(-1.15624053661742,-1.,-1.31362392696033));
#23857=CARTESIAN_POINT('Ctrl Pts',(-1.15950888730433,-1.,-1.3172297721596));
#23858=CARTESIAN_POINT('Ctrl Pts',(-1.16589330092532,-1.,-1.32428080720544));
#23859=CARTESIAN_POINT('Ctrl Pts',(-1.17501305787994,-1.,-1.33437539344842));
#23860=CARTESIAN_POINT('Ctrl Pts',(-1.18625865664915,-1.,-1.34687053998157));
#23861=CARTESIAN_POINT('Ctrl Pts',(-1.1987959077656,-1.,-1.36088705040677));
#23862=CARTESIAN_POINT('Ctrl Pts',(-1.20982812923113,-1.,-1.37331915604962));
#23863=CARTESIAN_POINT('Ctrl Pts',(-1.21938737278853,-1.,-1.38420564525391));
#23864=CARTESIAN_POINT('Ctrl Pts',(-1.22752961898063,-1.,-1.39361389567257));
#23865=CARTESIAN_POINT('Ctrl Pts',(-1.23434087289768,-1.,-1.40164708205345));
#23866=CARTESIAN_POINT('Ctrl Pts',(-1.23994455029421,-1.,-1.40845295531151));
#23867=CARTESIAN_POINT('Ctrl Pts',(-1.24450600513278,-1.,-1.41422913175437));
#23868=CARTESIAN_POINT('Ctrl Pts',(-1.24824430986911,-1.,-1.41923722596421));
#23869=CARTESIAN_POINT('Ctrl Pts',(-1.25141455570299,-1.,-1.42378102115911));
#23870=CARTESIAN_POINT('Ctrl Pts',(-1.25426945222783,-1.,-1.42815938799555));
#23871=CARTESIAN_POINT('Ctrl Pts',(-1.25702687965744,-1.,-1.43262645609679));
#23872=CARTESIAN_POINT('Ctrl Pts',(-1.25983531011894,-1.,-1.43734919180719));
#23873=CARTESIAN_POINT('Ctrl Pts',(-1.26273903323723,-1.,-1.44236470511145));
#23874=CARTESIAN_POINT('Ctrl Pts',(-1.26570925118767,-1.,-1.44761985001544));
#23875=CARTESIAN_POINT('Ctrl Pts',(-1.26867786804854,-1.,-1.45301422764205));
#23876=CARTESIAN_POINT('Ctrl Pts',(-1.27156805265312,-1.,-1.45843906294725));
#23877=CARTESIAN_POINT('Ctrl Pts',(-1.27433119897877,-1.,-1.4638243133254));
#23878=CARTESIAN_POINT('Ctrl Pts',(-1.27696414831144,-1.,-1.46916035917197));
#23879=CARTESIAN_POINT('Ctrl Pts',(-1.27948918248524,-1.,-1.4744717526711));
#23880=CARTESIAN_POINT('Ctrl Pts',(-1.28194158939522,-1.,-1.47980070347102));
#23881=CARTESIAN_POINT('Ctrl Pts',(-1.28435533880184,-1.,-1.48518817118891));
#23882=CARTESIAN_POINT('Ctrl Pts',(-1.28674676116415,-1.,-1.4906522831275));
#23883=CARTESIAN_POINT('Ctrl Pts',(-1.28911506584232,-1.,-1.49618896881729));
#23884=CARTESIAN_POINT('Ctrl Pts',(-1.29145022885171,-1.,-1.50178230149764));
#23885=CARTESIAN_POINT('Ctrl Pts',(-1.29373841372843,-1.,-1.50741159078367));
#23886=CARTESIAN_POINT('Ctrl Pts',(-1.29596850710518,-1.,-1.51305994241412));
#23887=CARTESIAN_POINT('Ctrl Pts',(-1.29813791800757,-1.,-1.51872184912735));
#23888=CARTESIAN_POINT('Ctrl Pts',(-1.30024984366334,-1.,-1.5243995786107));
#23889=CARTESIAN_POINT('Ctrl Pts',(-1.3023106439557,-1.,-1.53009970283893));
#23890=CARTESIAN_POINT('Ctrl Pts',(-1.30432735639487,-1.,-1.53582981268976));
#23891=CARTESIAN_POINT('Ctrl Pts',(-1.30630475189553,-1.,-1.54159462645428));
#23892=CARTESIAN_POINT('Ctrl Pts',(-1.30824393907471,-1.,-1.54739413957183));
#23893=CARTESIAN_POINT('Ctrl Pts',(-1.31014393684221,-1.,-1.55322568759481));
#23894=CARTESIAN_POINT('Ctrl Pts',(-1.31200264341696,-1.,-1.55908521254822));
#23895=CARTESIAN_POINT('Ctrl Pts',(-1.31381795281002,-1.,-1.56496872402352));
#23896=CARTESIAN_POINT('Ctrl Pts',(-1.31558903860015,-1.,-1.57087397835721));
#23897=CARTESIAN_POINT('Ctrl Pts',(-1.31731642317183,-1.,-1.57680056505585));
#23898=CARTESIAN_POINT('Ctrl Pts',(-1.31900135021428,-1.,-1.58274907898829));
#23899=CARTESIAN_POINT('Ctrl Pts',(-1.32064537110891,-1.,-1.58872057258244));
#23900=CARTESIAN_POINT('Ctrl Pts',(-1.32224985747686,-1.,-1.59471591079408));
#23901=CARTESIAN_POINT('Ctrl Pts',(-1.32381550858266,-1.,-1.600735118587));
#23902=CARTESIAN_POINT('Ctrl Pts',(-1.32534250785794,-1.,-1.6067775829097));
#23903=CARTESIAN_POINT('Ctrl Pts',(-1.32683074483365,-1.,-1.61284234015762));
#23904=CARTESIAN_POINT('Ctrl Pts',(-1.32828000610448,-1.,-1.61892832270723));
#23905=CARTESIAN_POINT('Ctrl Pts',(-1.32969019505665,-1.,-1.62503464209777));
#23906=CARTESIAN_POINT('Ctrl Pts',(-1.33106149345618,-1.,-1.63116079730887));
#23907=CARTESIAN_POINT('Ctrl Pts',(-1.33239425103694,-1.,-1.6373065347505));
#23908=CARTESIAN_POINT('Ctrl Pts',(-1.33368890676554,-1.,-1.64347174856007));
#23909=CARTESIAN_POINT('Ctrl Pts',(-1.33494590468003,-1.,-1.64965637286843));
#23910=CARTESIAN_POINT('Ctrl Pts',(-1.33616559745217,-1.,-1.65586025952651));
#23911=CARTESIAN_POINT('Ctrl Pts',(-1.33734820885331,-1.,-1.66208312542073));
#23912=CARTESIAN_POINT('Ctrl Pts',(-1.33849388654458,-1.,-1.66832460784078));
#23913=CARTESIAN_POINT('Ctrl Pts',(-1.33960273470372,-1.,-1.67458429426126));
#23914=CARTESIAN_POINT('Ctrl Pts',(-1.3406748518516,-1.,-1.68086176030308));
#23915=CARTESIAN_POINT('Ctrl Pts',(-1.34171037484673,-1.,-1.68715660868602));
#23916=CARTESIAN_POINT('Ctrl Pts',(-1.34270948206139,-1.,-1.6934684849664));
#23917=CARTESIAN_POINT('Ctrl Pts',(-1.34367237124322,-1.,-1.69979707754221));
#23918=CARTESIAN_POINT('Ctrl Pts',(-1.34459924533783,-1.,-1.70614212266676));
#23919=CARTESIAN_POINT('Ctrl Pts',(-1.34549029589563,-1.,-1.71250340687011));
#23920=CARTESIAN_POINT('Ctrl Pts',(-1.34634568653586,-1.,-1.7188807715095));
#23921=CARTESIAN_POINT('Ctrl Pts',(-1.34716554820013,-1.,-1.72527410681298));
#23922=CARTESIAN_POINT('Ctrl Pts',(-1.3477930915247,-1.,-1.73040149654497));
#23923=CARTESIAN_POINT('Ctrl Pts',(-1.34824783113158,-1.,-1.73425417886255));
#23924=CARTESIAN_POINT('Ctrl Pts',(-1.34854391898145,-1.,-1.73682580585819));
#23925=CARTESIAN_POINT('Ctrl Pts',(-1.34869019493419,-1.,-1.73811241238545));
#23926=CARTESIAN_POINT('',(-1.23627494547115,-1.,-1.81978687191668));
#23927=CARTESIAN_POINT('',(-1.34869019493419,-1.,-1.73811241238545));
#23928=CARTESIAN_POINT('',(-0.892032620296855,-1.,-1.5055822144029));
#23929=CARTESIAN_POINT('Ctrl Pts',(-1.23627494547115,-1.,-1.81978687191668));
#23930=CARTESIAN_POINT('Ctrl Pts',(-1.23509651170384,-1.,-1.81925017193531));
#23931=CARTESIAN_POINT('Ctrl Pts',(-1.23274224526804,-1.,-1.81817389920914));
#23932=CARTESIAN_POINT('Ctrl Pts',(-1.22921864890975,-1.,-1.81655087183054));
#23933=CARTESIAN_POINT('Ctrl Pts',(-1.22453613304507,-1.,-1.81436959209778));
#23934=CARTESIAN_POINT('Ctrl Pts',(-1.2187090610323,-1.,-1.81161420806172));
#23935=CARTESIAN_POINT('Ctrl Pts',(-1.2129081570818,-1.,-1.80882996916931));
#23936=CARTESIAN_POINT('Ctrl Pts',(-1.20713356605519,-1.,-1.80601678480772));
#23937=CARTESIAN_POINT('Ctrl Pts',(-1.2013854893912,-1.,-1.8031745483882));
#23938=CARTESIAN_POINT('Ctrl Pts',(-1.19566418930405,-1.,-1.80030314370121));
#23939=CARTESIAN_POINT('Ctrl Pts',(-1.1899699793456,-1.,-1.79740245923649));
#23940=CARTESIAN_POINT('Ctrl Pts',(-1.18430321697471,-1.,-1.79447240321572));
#23941=CARTESIAN_POINT('Ctrl Pts',(-1.17866429440781,-1.,-1.79151291552646));
#23942=CARTESIAN_POINT('Ctrl Pts',(-1.17305363177265,-1.,-1.78852398877523));
#23943=CARTESIAN_POINT('Ctrl Pts',(-1.16747166312239,-1.,-1.78550566040349));
#23944=CARTESIAN_POINT('Ctrl Pts',(-1.16191881298458,-1.,-1.78245795880949));
#23945=CARTESIAN_POINT('Ctrl Pts',(-1.15639547194689,-1.,-1.77938085564261));
#23946=CARTESIAN_POINT('Ctrl Pts',(-1.15090197841531,-1.,-1.77627422557034));
#23947=CARTESIAN_POINT('Ctrl Pts',(-1.14543858226948,-1.,-1.77313777896234));
#23948=CARTESIAN_POINT('Ctrl Pts',(-1.14000548337,-1.,-1.76997111386806));
#23949=CARTESIAN_POINT('Ctrl Pts',(-1.13460291804635,-1.,-1.76677384551883));
#23950=CARTESIAN_POINT('Ctrl Pts',(-1.12923123555076,-1.,-1.76354571966171));
#23951=CARTESIAN_POINT('Ctrl Pts',(-1.12389096855078,-1.,-1.76028671825084));
#23952=CARTESIAN_POINT('Ctrl Pts',(-1.11858293216752,-1.,-1.75699720772089));
#23953=CARTESIAN_POINT('Ctrl Pts',(-1.11330807582542,-1.,-1.75367772094617));
#23954=CARTESIAN_POINT('Ctrl Pts',(-1.10806728183003,-1.,-1.75032866075914));
#23955=CARTESIAN_POINT('Ctrl Pts',(-1.10286118991144,-1.,-1.74695004214924));
#23956=CARTESIAN_POINT('Ctrl Pts',(-1.09768999241229,-1.,-1.74354119236212));
#23957=CARTESIAN_POINT('Ctrl Pts',(-1.09255329056496,-1.,-1.74010053962252));
#23958=CARTESIAN_POINT('Ctrl Pts',(-1.08745056285429,-1.,-1.73662628326093));
#23959=CARTESIAN_POINT('Ctrl Pts',(-1.08238162784749,-1.,-1.73311705663407));
#23960=CARTESIAN_POINT('Ctrl Pts',(-1.0773470373727,-1.,-1.72957248977424));
#23961=CARTESIAN_POINT('Ctrl Pts',(-1.07234866990252,-1.,-1.72599406198489));
#23962=CARTESIAN_POINT('Ctrl Pts',(-1.06738966975463,-1.,-1.72238500928456));
#23963=CARTESIAN_POINT('Ctrl Pts',(-1.0624732468065,-1.,-1.71874858456908));
#23964=CARTESIAN_POINT('Ctrl Pts',(-1.05760163192481,-1.,-1.71508654427022));
#23965=CARTESIAN_POINT('Ctrl Pts',(-1.05277517202854,-1.,-1.71139783543986));
#23966=CARTESIAN_POINT('Ctrl Pts',(-1.0479908540499,-1.,-1.70767646263641));
#23967=CARTESIAN_POINT('Ctrl Pts',(-1.04324363334546,-1.,-1.70391338707969));
#23968=CARTESIAN_POINT('Ctrl Pts',(-1.03852922490782,-1.,-1.70010052930951));
#23969=CARTESIAN_POINT('Ctrl Pts',(-1.03384646003587,-1.,-1.69623414782769));
#23970=CARTESIAN_POINT('Ctrl Pts',(-1.02919977579155,-1.,-1.69231840863471));
#23971=CARTESIAN_POINT('Ctrl Pts',(-1.02460180535272,-1.,-1.68836910178475));
#23972=CARTESIAN_POINT('Ctrl Pts',(-1.02006795074222,-1.,-1.68440578021739));
#23973=CARTESIAN_POINT('Ctrl Pts',(-1.01561026162787,-1.,-1.6804428989482));
#23974=CARTESIAN_POINT('Ctrl Pts',(-1.01123236493507,-1.,-1.67648246776457));
#23975=CARTESIAN_POINT('Ctrl Pts',(-1.00692206696387,-1.,-1.67250335383248));
#23976=CARTESIAN_POINT('Ctrl Pts',(-1.00265091003682,-1.,-1.66846059277231));
#23977=CARTESIAN_POINT('Ctrl Pts',(-0.998389654952317,-1.,-1.66430758030304));
#23978=CARTESIAN_POINT('Ctrl Pts',(-0.994121836661116,-1.,-1.66001553809916));
#23979=CARTESIAN_POINT('Ctrl Pts',(-0.98985562785445,-1.,-1.65559044289746));
#23980=CARTESIAN_POINT('Ctrl Pts',(-0.985642622921626,-1.,-1.6511001661277));
#23981=CARTESIAN_POINT('Ctrl Pts',(-0.981562530940574,-1.,-1.64665139190834));
#23982=CARTESIAN_POINT('Ctrl Pts',(-0.977689794120297,-1.,-1.64233990826831));
#23983=CARTESIAN_POINT('Ctrl Pts',(-0.974066058287501,-1.,-1.63820952658157));
#23984=CARTESIAN_POINT('Ctrl Pts',(-0.970669715996356,-1.,-1.63420665729609));
#23985=CARTESIAN_POINT('Ctrl Pts',(-0.967387853228041,-1.,-1.63013849959083));
#23986=CARTESIAN_POINT('Ctrl Pts',(-0.964046107037821,-1.,-1.6257193066974));
#23987=CARTESIAN_POINT('Ctrl Pts',(-0.960438326099958,-1.,-1.62061638139929));
#23988=CARTESIAN_POINT('Ctrl Pts',(-0.956354422921573,-1.,-1.61449324337233));
#23989=CARTESIAN_POINT('Ctrl Pts',(-0.951613284361248,-1.,-1.60706069897794));
#23990=CARTESIAN_POINT('Ctrl Pts',(-0.946078063325796,-1.,-1.59810042045408));
#23991=CARTESIAN_POINT('Ctrl Pts',(-0.939646377909319,-1.,-1.58744937489796));
#23992=CARTESIAN_POINT('Ctrl Pts',(-0.932246680128849,-1.,-1.57499388385561));
#23993=CARTESIAN_POINT('Ctrl Pts',(-0.923832188966322,-1.,-1.56065988582509));
#23994=CARTESIAN_POINT('Ctrl Pts',(-0.91437591904658,-1.,-1.54440491152808));
#23995=CARTESIAN_POINT('Ctrl Pts',(-0.905967409640499,-1.,-1.52984849890434));
#23996=CARTESIAN_POINT('Ctrl Pts',(-0.89918504749193,-1.,-1.51805569591479));
#23997=CARTESIAN_POINT('Ctrl Pts',(-0.894452006967538,-1.,-1.50980486807181));
#23998=CARTESIAN_POINT('Ctrl Pts',(-0.892032620296855,-1.,-1.5055822144029));
#23999=CARTESIAN_POINT('',(-0.693717979106305,-1.,-1.60662857109684));
#24000=CARTESIAN_POINT('Origin',(0.,-1.,0.));
#24001=CARTESIAN_POINT('',(-0.745574324794401,-1.,-2.0698113262342));
#24002=CARTESIAN_POINT('Ctrl Pts',(-0.693717979106305,-1.,-1.60662857109684));
#24003=CARTESIAN_POINT('Ctrl Pts',(-0.69571209787897,-1.,-1.61106790957619));
#24004=CARTESIAN_POINT('Ctrl Pts',(-0.699605146398837,-1.,-1.61974673471117));
#24005=CARTESIAN_POINT('Ctrl Pts',(-0.705159151977294,-1.,-1.6321654166204));
#24006=CARTESIAN_POINT('Ctrl Pts',(-0.711993139340447,-1.,-1.64752408828442));
#24007=CARTESIAN_POINT('Ctrl Pts',(-0.71958543378795,-1.,-1.66472880551777));
#24008=CARTESIAN_POINT('Ctrl Pts',(-0.726235967982445,-1.,-1.67996158451922));
#24009=CARTESIAN_POINT('Ctrl Pts',(-0.731963238685357,-1.,-1.69326921972915));
#24010=CARTESIAN_POINT('Ctrl Pts',(-0.736799665716932,-1.,-1.70473309004249));
#24011=CARTESIAN_POINT('Ctrl Pts',(-0.74079516202821,-1.,-1.71447789751001));
#24012=CARTESIAN_POINT('Ctrl Pts',(-0.744021445433093,-1.,-1.72268229916769));
#24013=CARTESIAN_POINT('Ctrl Pts',(-0.746574710097752,-1.,-1.72958533647714));
#24014=CARTESIAN_POINT('Ctrl Pts',(-0.74858246295687,-1.,-1.7355035168033));
#24015=CARTESIAN_POINT('Ctrl Pts',(-0.750193435981249,-1.,-1.74080458267114));
#24016=CARTESIAN_POINT('Ctrl Pts',(-0.751555614164482,-1.,-1.74585086852502));
#24017=CARTESIAN_POINT('Ctrl Pts',(-0.752797683531314,-1.,-1.75095139468794));
#24018=CARTESIAN_POINT('Ctrl Pts',(-0.754009254027829,-1.,-1.75631083600019));
#24019=CARTESIAN_POINT('Ctrl Pts',(-0.755220979974461,-1.,-1.76197817240128));
#24020=CARTESIAN_POINT('Ctrl Pts',(-0.75642189602781,-1.,-1.76789396002998));
#24021=CARTESIAN_POINT('Ctrl Pts',(-0.757578264077029,-1.,-1.77394167108292));
#24022=CARTESIAN_POINT('Ctrl Pts',(-0.758650626677518,-1.,-1.77999411220945));
#24023=CARTESIAN_POINT('Ctrl Pts',(-0.759614401110189,-1.,-1.78596964884604));
#24024=CARTESIAN_POINT('Ctrl Pts',(-0.760469555880749,-1.,-1.7918581561088));
#24025=CARTESIAN_POINT('Ctrl Pts',(-0.761229695230558,-1.,-1.79768986997783));
#24026=CARTESIAN_POINT('Ctrl Pts',(-0.761915336443547,-1.,-1.80351583877342));
#24027=CARTESIAN_POINT('Ctrl Pts',(-0.762546129463938,-1.,-1.80938551463965));
#24028=CARTESIAN_POINT('Ctrl Pts',(-0.763132003836634,-1.,-1.8153211840553));
#24029=CARTESIAN_POINT('Ctrl Pts',(-0.763673465462726,-1.,-1.82131873145266));
#24030=CARTESIAN_POINT('Ctrl Pts',(-0.764165902605995,-1.,-1.82735991200065));
#24031=CARTESIAN_POINT('Ctrl Pts',(-0.764602549687853,-1.,-1.83342077227142));
#24032=CARTESIAN_POINT('Ctrl Pts',(-0.764978057881737,-1.,-1.83948181064835));
#24033=CARTESIAN_POINT('Ctrl Pts',(-0.765291664862029,-1.,-1.84553698875924));
#24034=CARTESIAN_POINT('Ctrl Pts',(-0.765545710619062,-1.,-1.85158945130063));
#24035=CARTESIAN_POINT('Ctrl Pts',(-0.765744212909318,-1.,-1.85764741390394));
#24036=CARTESIAN_POINT('Ctrl Pts',(-0.765891519092547,-1.,-1.86372027063312));
#24037=CARTESIAN_POINT('Ctrl Pts',(-0.765990708546091,-1.,-1.86981398314341));
#24038=CARTESIAN_POINT('Ctrl Pts',(-0.766042837036744,-1.,-1.87592888967883));
#24039=CARTESIAN_POINT('Ctrl Pts',(-0.766047794851865,-1.,-1.88206215302561));
#24040=CARTESIAN_POINT('Ctrl Pts',(-0.766004837062091,-1.,-1.88820926433409));
#24041=CARTESIAN_POINT('Ctrl Pts',(-0.765913193856978,-1.,-1.89436577771388));
#24042=CARTESIAN_POINT('Ctrl Pts',(-0.765772772593386,-1.,-1.90052930393596));
#24043=CARTESIAN_POINT('Ctrl Pts',(-0.765584196937919,-1.,-1.90669961402356));
#24044=CARTESIAN_POINT('Ctrl Pts',(-0.765348465884722,-1.,-1.91287765805169));
#24045=CARTESIAN_POINT('Ctrl Pts',(-0.765066729667088,-1.,-1.91906491634196));
#24046=CARTESIAN_POINT('Ctrl Pts',(-0.764740025488211,-1.,-1.92526263537048));
#24047=CARTESIAN_POINT('Ctrl Pts',(-0.764369010673941,-1.,-1.93147105496382));
#24048=CARTESIAN_POINT('Ctrl Pts',(-0.763954049121458,-1.,-1.93768964875886));
#24049=CARTESIAN_POINT('Ctrl Pts',(-0.763495333538629,-1.,-1.9439174661764));
#24050=CARTESIAN_POINT('Ctrl Pts',(-0.762992990878769,-1.,-1.95015342590024));
#24051=CARTESIAN_POINT('Ctrl Pts',(-0.762447203806179,-1.,-1.95639665309869));
#24052=CARTESIAN_POINT('Ctrl Pts',(-0.761858300014423,-1.,-1.96264672744186));
#24053=CARTESIAN_POINT('Ctrl Pts',(-0.76122669048382,-1.,-1.96890351582499));
#24054=CARTESIAN_POINT('Ctrl Pts',(-0.760552825409757,-1.,-1.97516705321494));
#24055=CARTESIAN_POINT('Ctrl Pts',(-0.75983714745219,-1.,-1.98143741418172));
#24056=CARTESIAN_POINT('Ctrl Pts',(-0.759080037802488,-1.,-1.98771456680874));
#24057=CARTESIAN_POINT('Ctrl Pts',(-0.758281796766761,-1.,-1.99399831098817));
#24058=CARTESIAN_POINT('Ctrl Pts',(-0.757442676862724,-1.,-2.00028834739178));
#24059=CARTESIAN_POINT('Ctrl Pts',(-0.75656290464667,-1.,-2.0065843158773));
#24060=CARTESIAN_POINT('Ctrl Pts',(-0.755642704957865,-1.,-2.01288584328084));
#24061=CARTESIAN_POINT('Ctrl Pts',(-0.754682330722816,-1.,-2.01919259405809));
#24062=CARTESIAN_POINT('Ctrl Pts',(-0.753682061112768,-1.,-2.02550428623313));
#24063=CARTESIAN_POINT('Ctrl Pts',(-0.752642180487211,-1.,-2.03182068456221));
#24064=CARTESIAN_POINT('Ctrl Pts',(-0.751562963361115,-1.,-2.03814160092099));
#24065=CARTESIAN_POINT('Ctrl Pts',(-0.750444657875576,-1.,-2.04446689147979));
#24066=CARTESIAN_POINT('Ctrl Pts',(-0.749287468665046,-1.,-2.05079645592154));
#24067=CARTESIAN_POINT('Ctrl Pts',(-0.748091554183802,-1.,-2.05713023031006));
#24068=CARTESIAN_POINT('Ctrl Pts',(-0.747103932787919,-1.,-2.06220058927826));
#24069=CARTESIAN_POINT('Ctrl Pts',(-0.7463458715442,-1.,-2.06600523016815));
#24070=CARTESIAN_POINT('Ctrl Pts',(-0.745832791378367,-1.,-2.06854248895728));
#24071=CARTESIAN_POINT('Ctrl Pts',(-0.745574324794401,-1.,-2.0698113262342));
#24072=CARTESIAN_POINT('',(-0.61342227326009,-1.,-2.11275013067528));
#24073=CARTESIAN_POINT('',(-0.745574324794401,-1.,-2.0698113262342));
#24074=CARTESIAN_POINT('',(-0.383122945602004,-1.,-1.7075470150345));
#24075=CARTESIAN_POINT('Ctrl Pts',(-0.61342227326009,-1.,-2.11275013067528));
#24076=CARTESIAN_POINT('Ctrl Pts',(-0.6124673655618,-1.,-2.11187554259986));
#24077=CARTESIAN_POINT('Ctrl Pts',(-0.610560911689899,-1.,-2.11012443807238));
#24078=CARTESIAN_POINT('Ctrl Pts',(-0.607711315454876,-1.,-2.1074919961518));
#24079=CARTESIAN_POINT('Ctrl Pts',(-0.60393203073603,-1.,-2.10397049886949));
#24080=CARTESIAN_POINT('Ctrl Pts',(-0.599241616420533,-1.,-2.0995493086477));
#24081=CARTESIAN_POINT('Ctrl Pts',(-0.594585006052162,-1.,-2.0951087622027));
#24082=CARTESIAN_POINT('Ctrl Pts',(-0.589962365403406,-1.,-2.09064881812129));
#24083=CARTESIAN_POINT('Ctrl Pts',(-0.585373918991617,-1.,-2.08616943727951));
#24084=CARTESIAN_POINT('Ctrl Pts',(-0.580819952108063,-1.,-2.08167059018418));
#24085=CARTESIAN_POINT('Ctrl Pts',(-0.576300797416844,-1.,-2.07715226767559));
#24086=CARTESIAN_POINT('Ctrl Pts',(-0.571816823242603,-1.,-2.07261449292824));
#24087=CARTESIAN_POINT('Ctrl Pts',(-0.567368421181087,-1.,-2.06805732997334));
#24088=CARTESIAN_POINT('Ctrl Pts',(-0.562955993082261,-1.,-2.06348090160589));
#24089=CARTESIAN_POINT('Ctrl Pts',(-0.558579940185151,-1.,-2.05888537756462));
#24090=CARTESIAN_POINT('Ctrl Pts',(-0.554240657463906,-1.,-2.05427091604413));
#24091=CARTESIAN_POINT('Ctrl Pts',(-0.549938525150295,-1.,-2.04963761077958));
#24092=CARTESIAN_POINT('Ctrl Pts',(-0.54567390381743,-1.,-2.04498544714588));
#24093=CARTESIAN_POINT('Ctrl Pts',(-0.541447120615659,-1.,-2.04031422690527));
#24094=CARTESIAN_POINT('Ctrl Pts',(-0.537258489833262,-1.,-2.03562362954037));
#24095=CARTESIAN_POINT('Ctrl Pts',(-0.533108355132977,-1.,-2.03091336214426));
#24096=CARTESIAN_POINT('Ctrl Pts',(-0.528997127241914,-1.,-2.0261832908329));
#24097=CARTESIAN_POINT('Ctrl Pts',(-0.524925318333476,-1.,-2.02143356304698));
#24098=CARTESIAN_POINT('Ctrl Pts',(-0.52089359039937,-1.,-2.01666477917286));
#24099=CARTESIAN_POINT('Ctrl Pts',(-0.516902681728687,-1.,-2.01187773939242));
#24100=CARTESIAN_POINT('Ctrl Pts',(-0.512953306961792,-1.,-2.00707309946949));
#24101=CARTESIAN_POINT('Ctrl Pts',(-0.509046069886157,-1.,-2.00225107134734));
#24102=CARTESIAN_POINT('Ctrl Pts',(-0.505181361323026,-1.,-1.99741107463572));
#24103=CARTESIAN_POINT('Ctrl Pts',(-0.501359287727146,-1.,-1.99255149126155));
#24104=CARTESIAN_POINT('Ctrl Pts',(-0.497579909545574,-1.,-1.98767044752932));
#24105=CARTESIAN_POINT('Ctrl Pts',(-0.493843476541495,-1.,-1.98276658761821));
#24106=CARTESIAN_POINT('Ctrl Pts',(-0.490150627860952,-1.,-1.97783973019229));
#24107=CARTESIAN_POINT('Ctrl Pts',(-0.486502692907659,-1.,-1.97289186263272));
#24108=CARTESIAN_POINT('Ctrl Pts',(-0.482901662120691,-1.,-1.96792703422362));
#24109=CARTESIAN_POINT('Ctrl Pts',(-0.479349583074855,-1.,-1.96294933055943));
#24110=CARTESIAN_POINT('Ctrl Pts',(-0.475848034683176,-1.,-1.95796111148177));
#24111=CARTESIAN_POINT('Ctrl Pts',(-0.472397672264072,-1.,-1.95296148278133));
#24112=CARTESIAN_POINT('Ctrl Pts',(-0.468997482913135,-1.,-1.94794381136514));
#24113=CARTESIAN_POINT('Ctrl Pts',(-0.46564546202603,-1.,-1.9428979419619));
#24114=CARTESIAN_POINT('Ctrl Pts',(-0.462340031009056,-1.,-1.93781486640821));
#24115=CARTESIAN_POINT('Ctrl Pts',(-0.459081234547926,-1.,-1.93269066517934));
#24116=CARTESIAN_POINT('Ctrl Pts',(-0.455872005174371,-1.,-1.92753067150476));
#24117=CARTESIAN_POINT('Ctrl Pts',(-0.452719478359432,-1.,-1.92235380648502));
#24118=CARTESIAN_POINT('Ctrl Pts',(-0.449632260106662,-1.,-1.91718342555755));
#24119=CARTESIAN_POINT('Ctrl Pts',(-0.446617343485711,-1.,-1.9120369998112));
#24120=CARTESIAN_POINT('Ctrl Pts',(-0.443677556849151,-1.,-1.90691756144898));
#24121=CARTESIAN_POINT('Ctrl Pts',(-0.440807833704038,-1.,-1.90180124389086));
#24122=CARTESIAN_POINT('Ctrl Pts',(-0.437995003948244,-1.,-1.89663648956466));
#24123=CARTESIAN_POINT('Ctrl Pts',(-0.435225660963383,-1.,-1.89136993975504));
#24124=CARTESIAN_POINT('Ctrl Pts',(-0.432493038548748,-1.,-1.88596913666793));
#24125=CARTESIAN_POINT('Ctrl Pts',(-0.429803062482344,-1.,-1.88044229001832));
#24126=CARTESIAN_POINT('Ctrl Pts',(-0.427183828519102,-1.,-1.87486989291484));
#24127=CARTESIAN_POINT('Ctrl Pts',(-0.424678177291359,-1.,-1.86937803944323));
#24128=CARTESIAN_POINT('Ctrl Pts',(-0.422327307418275,-1.,-1.86408083334028));
#24129=CARTESIAN_POINT('Ctrl Pts',(-0.420157287975619,-1.,-1.85903281096686));
#24130=CARTESIAN_POINT('Ctrl Pts',(-0.418164129143534,-1.,-1.85417632856234));
#24131=CARTESIAN_POINT('Ctrl Pts',(-0.416300022038864,-1.,-1.84929312929882));
#24132=CARTESIAN_POINT('Ctrl Pts',(-0.41448743825434,-1.,-1.8440575707371));
#24133=CARTESIAN_POINT('Ctrl Pts',(-0.412633125322162,-1.,-1.83808953475839));
#24134=CARTESIAN_POINT('Ctrl Pts',(-0.410641256301675,-1.,-1.83100408895216));
#24135=CARTESIAN_POINT('Ctrl Pts',(-0.408428948108533,-1.,-1.8224702267854));
#24136=CARTESIAN_POINT('Ctrl Pts',(-0.405933518411838,-1.,-1.81223801813988));
#24137=CARTESIAN_POINT('Ctrl Pts',(-0.403107976170441,-1.,-1.80012077176221));
#24138=CARTESIAN_POINT('Ctrl Pts',(-0.39991940378308,-1.,-1.78598826347533));
#24139=CARTESIAN_POINT('Ctrl Pts',(-0.39634619612042,-1.,-1.7697556004756));
#24140=CARTESIAN_POINT('Ctrl Pts',(-0.392375812294307,-1.,-1.75137405313962));
#24141=CARTESIAN_POINT('Ctrl Pts',(-0.388877023509191,-1.,-1.7349317097561));
#24142=CARTESIAN_POINT('Ctrl Pts',(-0.38607079032701,-1.,-1.72162022246158));
#24143=CARTESIAN_POINT('Ctrl Pts',(-0.384119047315542,-1.,-1.71231062891958));
#24144=CARTESIAN_POINT('Ctrl Pts',(-0.383122945602004,-1.,-1.7075470150345));
#24145=CARTESIAN_POINT('',(-0.163289472382896,-1.,-1.74236521665491));
#24146=CARTESIAN_POINT('Origin',(0.,-1.,0.));
#24147=CARTESIAN_POINT('',(-0.0694764450219581,-1.,-2.19890268624765));
#24148=CARTESIAN_POINT('Ctrl Pts',(-0.163289472382896,-1.,-1.74236521665491));
#24149=CARTESIAN_POINT('Ctrl Pts',(-0.163814161002002,-1.,-1.7472034950333));
#24150=CARTESIAN_POINT('Ctrl Pts',(-0.164834765707158,-1.,-1.75666056638427));
#24151=CARTESIAN_POINT('Ctrl Pts',(-0.1662793551464,-1.,-1.77018771684844));
#24152=CARTESIAN_POINT('Ctrl Pts',(-0.168032772805197,-1.,-1.7869064998507));
#24153=CARTESIAN_POINT('Ctrl Pts',(-0.169936923904608,-1.,-1.80561530629706));
#24154=CARTESIAN_POINT('Ctrl Pts',(-0.171554770204119,-1.,-1.82215766811545));
#24155=CARTESIAN_POINT('Ctrl Pts',(-0.1728894428919,-1.,-1.83658380527692));
#24156=CARTESIAN_POINT('Ctrl Pts',(-0.173946627587731,-1.,-1.8489811319852));
#24157=CARTESIAN_POINT('Ctrl Pts',(-0.17473525927603,-1.,-1.85948367088837));
#24158=CARTESIAN_POINT('Ctrl Pts',(-0.175268337590758,-1.,-1.86828349694799));
#24159=CARTESIAN_POINT('Ctrl Pts',(-0.175563480746485,-1.,-1.87563767773588));
#24160=CARTESIAN_POINT('Ctrl Pts',(-0.175644148889699,-1.,-1.88188663145367));
#24161=CARTESIAN_POINT('Ctrl Pts',(-0.175538155840648,-1.,-1.88742606273259));
#24162=CARTESIAN_POINT('Ctrl Pts',(-0.175274276190844,-1.,-1.892646301985));
#24163=CARTESIAN_POINT('Ctrl Pts',(-0.174879405091263,-1.,-1.89788101117132));
#24164=CARTESIAN_POINT('Ctrl Pts',(-0.174375518661085,-1.,-1.90335253862834));
#24165=CARTESIAN_POINT('Ctrl Pts',(-0.173776635257817,-1.,-1.90911693975267));
#24166=CARTESIAN_POINT('Ctrl Pts',(-0.173090695383496,-1.,-1.91511429159527));
#24167=CARTESIAN_POINT('Ctrl Pts',(-0.172321621259514,-1.,-1.9212233439798));
#24168=CARTESIAN_POINT('Ctrl Pts',(-0.171471191532988,-1.,-1.92731093582036));
#24169=CARTESIAN_POINT('Ctrl Pts',(-0.170541253116202,-1.,-1.93329183155539));
#24170=CARTESIAN_POINT('Ctrl Pts',(-0.169534904817491,-1.,-1.93915639211581));
#24171=CARTESIAN_POINT('Ctrl Pts',(-0.168455741607556,-1.,-1.94493757756931));
#24172=CARTESIAN_POINT('Ctrl Pts',(-0.167307501784475,-1.,-1.95069027794294));
#24173=CARTESIAN_POINT('Ctrl Pts',(-0.166093592002812,-1.,-1.9564675971873));
#24174=CARTESIAN_POINT('Ctrl Pts',(-0.164816568920269,-1.,-1.96229379940136));
#24175=CARTESIAN_POINT('Ctrl Pts',(-0.163478185457734,-1.,-1.96816512677967));
#24176=CARTESIAN_POINT('Ctrl Pts',(-0.162079693556289,-1.,-1.97406280235188));
#24177=CARTESIAN_POINT('Ctrl Pts',(-0.160622060784611,-1.,-1.97996195437559));
#24178=CARTESIAN_POINT('Ctrl Pts',(-0.159106226437299,-1.,-1.98584238283292));
#24179=CARTESIAN_POINT('Ctrl Pts',(-0.157533331459227,-1.,-1.99169810931908));
#24180=CARTESIAN_POINT('Ctrl Pts',(-0.155904629548783,-1.,-1.99753284771497));
#24181=CARTESIAN_POINT('Ctrl Pts',(-0.154221403049722,-1.,-2.00335565310543));
#24182=CARTESIAN_POINT('Ctrl Pts',(-0.15248488362145,-1.,-2.00917680318424));
#24183=CARTESIAN_POINT('Ctrl Pts',(-0.150696157673078,-1.,-2.01500291940238));
#24184=CARTESIAN_POINT('Ctrl Pts',(-0.148856124775337,-1.,-2.02083464969894));
#24185=CARTESIAN_POINT('Ctrl Pts',(-0.146965557332583,-1.,-2.02666926182017));
#24186=CARTESIAN_POINT('Ctrl Pts',(-0.145025140186057,-1.,-2.03250223739942));
#24187=CARTESIAN_POINT('Ctrl Pts',(-0.143035515058209,-1.,-2.03832911025912));
#24188=CARTESIAN_POINT('Ctrl Pts',(-0.140997332152546,-1.,-2.04414757947916));
#24189=CARTESIAN_POINT('Ctrl Pts',(-0.138911255368966,-1.,-2.04995762001328));
#24190=CARTESIAN_POINT('Ctrl Pts',(-0.136777941218044,-1.,-2.05576044414264));
#24191=CARTESIAN_POINT('Ctrl Pts',(-0.134598026192106,-1.,-2.06155781517842));
#24192=CARTESIAN_POINT('Ctrl Pts',(-0.13237211154771,-1.,-2.06735123910326));
#24193=CARTESIAN_POINT('Ctrl Pts',(-0.130100748328403,-1.,-2.07314114713063));
#24194=CARTESIAN_POINT('Ctrl Pts',(-0.12778444527612,-1.,-2.07892715110987));
#24195=CARTESIAN_POINT('Ctrl Pts',(-0.125423679412061,-1.,-2.08470840653643));
#24196=CARTESIAN_POINT('Ctrl Pts',(-0.123018905621083,-1.,-2.09048392424825));
#24197=CARTESIAN_POINT('Ctrl Pts',(-0.120570567965122,-1.,-2.0962529286773));
#24198=CARTESIAN_POINT('Ctrl Pts',(-0.118079107988355,-1.,-2.102015121329));
#24199=CARTESIAN_POINT('Ctrl Pts',(-0.115544957687926,-1.,-2.10777050261309));
#24200=CARTESIAN_POINT('Ctrl Pts',(-0.112968534419737,-1.,-2.11351924490306));
#24201=CARTESIAN_POINT('Ctrl Pts',(-0.110350236135025,-1.,-2.11926155590865));
#24202=CARTESIAN_POINT('Ctrl Pts',(-0.10769043523109,-1.,-2.12499752307));
#24203=CARTESIAN_POINT('Ctrl Pts',(-0.104989479152739,-1.,-2.13072704887293));
#24204=CARTESIAN_POINT('Ctrl Pts',(-0.1022477005561,-1.,-2.13644992667165));
#24205=CARTESIAN_POINT('Ctrl Pts',(-0.0994654261990915,-1.,-2.14216588396025));
#24206=CARTESIAN_POINT('Ctrl Pts',(-0.0966429852305459,-1.,-2.14787463531795));
#24207=CARTESIAN_POINT('Ctrl Pts',(-0.0937807218867643,-1.,-2.1535759397817));
#24208=CARTESIAN_POINT('Ctrl Pts',(-0.0908789888107265,-1.,-2.15926961544516));
#24209=CARTESIAN_POINT('Ctrl Pts',(-0.0879381291386923,-1.,-2.16495552645014));
#24210=CARTESIAN_POINT('Ctrl Pts',(-0.0849584620835372,-1.,-2.17063357870952));
#24211=CARTESIAN_POINT('Ctrl Pts',(-0.0819402680872765,-1.,-2.176303712113));
#24212=CARTESIAN_POINT('Ctrl Pts',(-0.0788837727685243,-1.,-2.18196589448887));
#24213=CARTESIAN_POINT('Ctrl Pts',(-0.0757891465836148,-1.,-2.1876201139953));
#24214=CARTESIAN_POINT('Ctrl Pts',(-0.0732830357306725,-1.,-2.19213712013662));
#24215=CARTESIAN_POINT('Ctrl Pts',(-0.0713863779526154,-1.,-2.19552129484002));
#24216=CARTESIAN_POINT('Ctrl Pts',(-0.070114353632549,-1.,-2.19777582085423));
#24217=CARTESIAN_POINT('Ctrl Pts',(-0.0694764450219581,-1.,-2.19890268624765));
#24218=CARTESIAN_POINT('',(0.0694764450219584,-1.,-2.19890268624765));
#24219=CARTESIAN_POINT('',(-0.0694764450219581,-1.,-2.19890268624765));
#24220=CARTESIAN_POINT('',(0.163289472382896,-1.,-1.74236521665491));
#24221=CARTESIAN_POINT('Ctrl Pts',(0.0694764450219584,-1.,-2.19890268624765));
#24222=CARTESIAN_POINT('Ctrl Pts',(0.0701143536324926,-1.,-2.19777582085261));
#24223=CARTESIAN_POINT('Ctrl Pts',(0.0713863779524627,-1.,-2.19552129483562));
#24224=CARTESIAN_POINT('Ctrl Pts',(0.0732830357304276,-1.,-2.19213712012956));
#24225=CARTESIAN_POINT('Ctrl Pts',(0.0757891465833411,-1.,-2.1876201139874));
#24226=CARTESIAN_POINT('Ctrl Pts',(0.0788837727683228,-1.,-2.18196589448304));
#24227=CARTESIAN_POINT('Ctrl Pts',(0.0819402680871939,-1.,-2.1763037121106));
#24228=CARTESIAN_POINT('Ctrl Pts',(0.0849584620835643,-1.,-2.17063357871031));
#24229=CARTESIAN_POINT('Ctrl Pts',(0.0879381291387823,-1.,-2.16495552645275));
#24230=CARTESIAN_POINT('Ctrl Pts',(0.0908789888108266,-1.,-2.15926961544808));
#24231=CARTESIAN_POINT('Ctrl Pts',(0.0937807218868345,-1.,-2.15357593978377));
#24232=CARTESIAN_POINT('Ctrl Pts',(0.0966429852305689,-1.,-2.14787463531864));
#24233=CARTESIAN_POINT('Ctrl Pts',(0.0994654261990743,-1.,-2.14216588395974));
#24234=CARTESIAN_POINT('Ctrl Pts',(0.102247700556064,-1.,-2.13644992667052));
#24235=CARTESIAN_POINT('Ctrl Pts',(0.104989479152703,-1.,-2.1307270488718));
#24236=CARTESIAN_POINT('Ctrl Pts',(0.107690435231068,-1.,-2.12499752306927));
#24237=CARTESIAN_POINT('Ctrl Pts',(0.11035023613502,-1.,-2.11926155590849));
#24238=CARTESIAN_POINT('Ctrl Pts',(0.112968534419746,-1.,-2.11351924490335));
#24239=CARTESIAN_POINT('Ctrl Pts',(0.11554495768794,-1.,-2.10777050261359));
#24240=CARTESIAN_POINT('Ctrl Pts',(0.118079107988368,-1.,-2.10201512132945));
#24241=CARTESIAN_POINT('Ctrl Pts',(0.120570567965129,-1.,-2.09625292867756));
#24242=CARTESIAN_POINT('Ctrl Pts',(0.123018905621083,-1.,-2.09048392424826));
#24243=CARTESIAN_POINT('Ctrl Pts',(0.125423679412058,-1.,-2.08470840653628));
#24244=CARTESIAN_POINT('Ctrl Pts',(0.127784445276116,-1.,-2.07892715110967));
#24245=CARTESIAN_POINT('Ctrl Pts',(0.1301007483284,-1.,-2.07314114713047));
#24246=CARTESIAN_POINT('Ctrl Pts',(0.13237211154771,-1.,-2.06735123910319));
#24247=CARTESIAN_POINT('Ctrl Pts',(0.134598026192107,-1.,-2.06155781517844));
#24248=CARTESIAN_POINT('Ctrl Pts',(0.136777941218044,-1.,-2.0557604441427));
#24249=CARTESIAN_POINT('Ctrl Pts',(0.138911255368966,-1.,-2.04995762001333));
#24250=CARTESIAN_POINT('Ctrl Pts',(0.140997332152545,-1.,-2.04414757947919));
#24251=CARTESIAN_POINT('Ctrl Pts',(0.143035515058208,-1.,-2.03832911025913));
#24252=CARTESIAN_POINT('Ctrl Pts',(0.145025140186058,-1.,-2.03250223739941));
#24253=CARTESIAN_POINT('Ctrl Pts',(0.146965557332586,-1.,-2.02666926182017));
#24254=CARTESIAN_POINT('Ctrl Pts',(0.148856124775343,-1.,-2.02083464969897));
#24255=CARTESIAN_POINT('Ctrl Pts',(0.150696157673084,-1.,-2.01500291940243));
#24256=CARTESIAN_POINT('Ctrl Pts',(0.152484883621452,-1.,-2.00917680318426));
#24257=CARTESIAN_POINT('Ctrl Pts',(0.154221403049719,-1.,-2.00335565310539));
#24258=CARTESIAN_POINT('Ctrl Pts',(0.155904629548774,-1.,-1.99753284771487));
#24259=CARTESIAN_POINT('Ctrl Pts',(0.157533331459215,-1.,-1.99169810931893));
#24260=CARTESIAN_POINT('Ctrl Pts',(0.159106226437288,-1.,-1.98584238283279));
#24261=CARTESIAN_POINT('Ctrl Pts',(0.16062206078461,-1.,-1.97996195437557));
#24262=CARTESIAN_POINT('Ctrl Pts',(0.162079693556302,-1.,-1.97406280235204));
#24263=CARTESIAN_POINT('Ctrl Pts',(0.16347818545776,-1.,-1.96816512678));
#24264=CARTESIAN_POINT('Ctrl Pts',(0.1648165689203,-1.,-1.96229379940174));
#24265=CARTESIAN_POINT('Ctrl Pts',(0.166093592002833,-1.,-1.95646759718755));
#24266=CARTESIAN_POINT('Ctrl Pts',(0.167307501784469,-1.,-1.95069027794286));
#24267=CARTESIAN_POINT('Ctrl Pts',(0.168455741607516,-1.,-1.94493757756879));
#24268=CARTESIAN_POINT('Ctrl Pts',(0.169534904817425,-1.,-1.93915639211497));
#24269=CARTESIAN_POINT('Ctrl Pts',(0.170541253116136,-1.,-1.93329183155455));
#24270=CARTESIAN_POINT('Ctrl Pts',(0.17147119153296,-1.,-1.92731093582));
#24271=CARTESIAN_POINT('Ctrl Pts',(0.172321621259557,-1.,-1.92122334398034));
#24272=CARTESIAN_POINT('Ctrl Pts',(0.173090695383619,-1.,-1.91511429159681));
#24273=CARTESIAN_POINT('Ctrl Pts',(0.173776635257984,-1.,-1.90911693975475));
#24274=CARTESIAN_POINT('Ctrl Pts',(0.174375518661222,-1.,-1.90335253863003));
#24275=CARTESIAN_POINT('Ctrl Pts',(0.174879405091277,-1.,-1.89788101117148));
#24276=CARTESIAN_POINT('Ctrl Pts',(0.175274276190664,-1.,-1.89264630198279));
#24277=CARTESIAN_POINT('Ctrl Pts',(0.175538155840286,-1.,-1.88742606272818));
#24278=CARTESIAN_POINT('Ctrl Pts',(0.175644148889271,-1.,-1.88188663144846));
#24279=CARTESIAN_POINT('Ctrl Pts',(0.175563480746205,-1.,-1.87563767773249));
#24280=CARTESIAN_POINT('Ctrl Pts',(0.175268337590901,-1.,-1.86828349694972));
#24281=CARTESIAN_POINT('Ctrl Pts',(0.174735259276856,-1.,-1.85948367089838));
#24282=CARTESIAN_POINT('Ctrl Pts',(0.173946627589401,-1.,-1.84898113200543));
#24283=CARTESIAN_POINT('Ctrl Pts',(0.17288944289442,-1.,-1.83658380530747));
#24284=CARTESIAN_POINT('Ctrl Pts',(0.171554770207306,-1.,-1.82215766815414));
#24285=CARTESIAN_POINT('Ctrl Pts',(0.169936923908078,-1.,-1.80561530633924));
#24286=CARTESIAN_POINT('Ctrl Pts',(0.16803277280837,-1.,-1.78690649988931));
#24287=CARTESIAN_POINT('Ctrl Pts',(0.166279355148738,-1.,-1.77018771687692));
#24288=CARTESIAN_POINT('Ctrl Pts',(0.164834765708484,-1.,-1.75666056640041));
#24289=CARTESIAN_POINT('Ctrl Pts',(0.163814161002474,-1.,-1.74720349503904));
#24290=CARTESIAN_POINT('Ctrl Pts',(0.163289472382896,-1.,-1.74236521665491));
#24291=CARTESIAN_POINT('',(0.383122945602004,-1.,-1.7075470150345));
#24292=CARTESIAN_POINT('Origin',(0.,-1.,0.));
#24293=CARTESIAN_POINT('',(0.61342227326009,-1.,-2.11275013067528));
#24294=CARTESIAN_POINT('Ctrl Pts',(0.383122945602004,-1.,-1.7075470150345));
#24295=CARTESIAN_POINT('Ctrl Pts',(0.384119047314215,-1.,-1.71231062891398));
#24296=CARTESIAN_POINT('Ctrl Pts',(0.386070790323281,-1.,-1.72162022244582));
#24297=CARTESIAN_POINT('Ctrl Pts',(0.388877023502615,-1.,-1.73493170972829));
#24298=CARTESIAN_POINT('Ctrl Pts',(0.392375812285395,-1.,-1.75137405310193));
#24299=CARTESIAN_POINT('Ctrl Pts',(0.396346196110688,-1.,-1.76975560043442));
#24300=CARTESIAN_POINT('Ctrl Pts',(0.399919403774155,-1.,-1.78598826343754));
#24301=CARTESIAN_POINT('Ctrl Pts',(0.403107976163396,-1.,-1.80012077173238));
#24302=CARTESIAN_POINT('Ctrl Pts',(0.405933518407175,-1.,-1.81223801812013));
#24303=CARTESIAN_POINT('Ctrl Pts',(0.408428948106227,-1.,-1.82247022677562));
#24304=CARTESIAN_POINT('Ctrl Pts',(0.410641256301276,-1.,-1.83100408895047));
#24305=CARTESIAN_POINT('Ctrl Pts',(0.412633125322945,-1.,-1.8380895347617));
#24306=CARTESIAN_POINT('Ctrl Pts',(0.414487438255542,-1.,-1.84405757074218));
#24307=CARTESIAN_POINT('Ctrl Pts',(0.416300022039885,-1.,-1.84929312930314));
#24308=CARTESIAN_POINT('Ctrl Pts',(0.418164129144045,-1.,-1.8541763285645));
#24309=CARTESIAN_POINT('Ctrl Pts',(0.420157287975583,-1.,-1.8590328109667));
#24310=CARTESIAN_POINT('Ctrl Pts',(0.422327307417884,-1.,-1.86408083333863));
#24311=CARTESIAN_POINT('Ctrl Pts',(0.424678177290876,-1.,-1.8693780394412));
#24312=CARTESIAN_POINT('Ctrl Pts',(0.427183828518743,-1.,-1.87486989291334));
#24313=CARTESIAN_POINT('Ctrl Pts',(0.429803062482217,-1.,-1.88044229001779));
#24314=CARTESIAN_POINT('Ctrl Pts',(0.432493038548833,-1.,-1.88596913666828));
#24315=CARTESIAN_POINT('Ctrl Pts',(0.43522566096358,-1.,-1.89136993975585));
#24316=CARTESIAN_POINT('Ctrl Pts',(0.437995003948443,-1.,-1.89663648956549));
#24317=CARTESIAN_POINT('Ctrl Pts',(0.44080783370416,-1.,-1.90180124389137));
#24318=CARTESIAN_POINT('Ctrl Pts',(0.44367755684917,-1.,-1.90691756144906));
#24319=CARTESIAN_POINT('Ctrl Pts',(0.446617343485651,-1.,-1.91203699981095));
#24320=CARTESIAN_POINT('Ctrl Pts',(0.449632260106572,-1.,-1.91718342555717));
#24321=CARTESIAN_POINT('Ctrl Pts',(0.452719478359356,-1.,-1.9223538064847));
#24322=CARTESIAN_POINT('Ctrl Pts',(0.455872005174335,-1.,-1.92753067150461));
#24323=CARTESIAN_POINT('Ctrl Pts',(0.459081234547931,-1.,-1.93269066517936));
#24324=CARTESIAN_POINT('Ctrl Pts',(0.462340031009087,-1.,-1.93781486640834));
#24325=CARTESIAN_POINT('Ctrl Pts',(0.465645462026064,-1.,-1.94289794196205));
#24326=CARTESIAN_POINT('Ctrl Pts',(0.468997482913158,-1.,-1.94794381136524));
#24327=CARTESIAN_POINT('Ctrl Pts',(0.472397672264079,-1.,-1.95296148278136));
#24328=CARTESIAN_POINT('Ctrl Pts',(0.475848034683171,-1.,-1.95796111148175));
#24329=CARTESIAN_POINT('Ctrl Pts',(0.479349583074846,-1.,-1.96294933055938));
#24330=CARTESIAN_POINT('Ctrl Pts',(0.482901662120686,-1.,-1.96792703422358));
#24331=CARTESIAN_POINT('Ctrl Pts',(0.486502692907661,-1.,-1.97289186263272));
#24332=CARTESIAN_POINT('Ctrl Pts',(0.490150627860955,-1.,-1.97783973019229));
#24333=CARTESIAN_POINT('Ctrl Pts',(0.493843476541492,-1.,-1.9827665876182));
#24334=CARTESIAN_POINT('Ctrl Pts',(0.497579909545564,-1.,-1.98767044752929));
#24335=CARTESIAN_POINT('Ctrl Pts',(0.501359287727129,-1.,-1.9925514912615));
#24336=CARTESIAN_POINT('Ctrl Pts',(0.505181361323011,-1.,-1.99741107463567));
#24337=CARTESIAN_POINT('Ctrl Pts',(0.509046069886152,-1.,-2.00225107134733));
#24338=CARTESIAN_POINT('Ctrl Pts',(0.512953306961813,-1.,-2.00707309946955));
#24339=CARTESIAN_POINT('Ctrl Pts',(0.516902681728733,-1.,-2.01187773939257));
#24340=CARTESIAN_POINT('Ctrl Pts',(0.520893590399428,-1.,-2.01666477917306));
#24341=CARTESIAN_POINT('Ctrl Pts',(0.524925318333518,-1.,-2.02143356304712));
#24342=CARTESIAN_POINT('Ctrl Pts',(0.52899712724191,-1.,-2.02618329083289));
#24343=CARTESIAN_POINT('Ctrl Pts',(0.533108355132905,-1.,-2.03091336214401));
#24344=CARTESIAN_POINT('Ctrl Pts',(0.537258489833134,-1.,-2.03562362953993));
#24345=CARTESIAN_POINT('Ctrl Pts',(0.54144712061552,-1.,-2.0403142269048));
#24346=CARTESIAN_POINT('Ctrl Pts',(0.545673903817348,-1.,-2.0449854471456));
#24347=CARTESIAN_POINT('Ctrl Pts',(0.549938525150342,-1.,-2.04963761077974));
#24348=CARTESIAN_POINT('Ctrl Pts',(0.554240657464109,-1.,-2.05427091604482));
#24349=CARTESIAN_POINT('Ctrl Pts',(0.558579940185467,-1.,-2.05888537756571));
#24350=CARTESIAN_POINT('Ctrl Pts',(0.562955993082574,-1.,-2.06348090160697));
#24351=CARTESIAN_POINT('Ctrl Pts',(0.567368421181229,-1.,-2.06805732997383));
#24352=CARTESIAN_POINT('Ctrl Pts',(0.571816823242411,-1.,-2.07261449292758));
#24353=CARTESIAN_POINT('Ctrl Pts',(0.576300797416274,-1.,-2.07715226767361));
#24354=CARTESIAN_POINT('Ctrl Pts',(0.580819952107256,-1.,-2.08167059018138));
#24355=CARTESIAN_POINT('Ctrl Pts',(0.585373918990895,-1.,-2.086169437277));
#24356=CARTESIAN_POINT('Ctrl Pts',(0.589962365403189,-1.,-2.09064881812053));
#24357=CARTESIAN_POINT('Ctrl Pts',(0.594585006052823,-1.,-2.09510876220501));
#24358=CARTESIAN_POINT('Ctrl Pts',(0.599241616422144,-1.,-2.09954930865331));
#24359=CARTESIAN_POINT('Ctrl Pts',(0.603932030738212,-1.,-2.10397049887709));
#24360=CARTESIAN_POINT('Ctrl Pts',(0.607711315456826,-1.,-2.10749199615859));
#24361=CARTESIAN_POINT('Ctrl Pts',(0.610560911691113,-1.,-2.11012443807661));
#24362=CARTESIAN_POINT('Ctrl Pts',(0.61246736556225,-1.,-2.11187554260142));
#24363=CARTESIAN_POINT('Ctrl Pts',(0.61342227326009,-1.,-2.11275013067528));
#24364=CARTESIAN_POINT('',(0.745574324794401,-1.,-2.0698113262342));
#24365=CARTESIAN_POINT('',(0.61342227326009,-1.,-2.11275013067528));
#24366=CARTESIAN_POINT('',(0.693717979106306,-1.,-1.60662857109684));
#24367=CARTESIAN_POINT('Ctrl Pts',(0.745574324794401,-1.,-2.0698113262342));
#24368=CARTESIAN_POINT('Ctrl Pts',(0.74583279137781,-1.,-2.06854248895575));
#24369=CARTESIAN_POINT('Ctrl Pts',(0.746345871542695,-1.,-2.06600523016401));
#24370=CARTESIAN_POINT('Ctrl Pts',(0.747103932785504,-1.,-2.06220058927162));
#24371=CARTESIAN_POINT('Ctrl Pts',(0.748091554181101,-1.,-2.05713023030263));
#24372=CARTESIAN_POINT('Ctrl Pts',(0.749287468663053,-1.,-2.05079645591606));
#24373=CARTESIAN_POINT('Ctrl Pts',(0.750444657874758,-1.,-2.04446689147754));
#24374=CARTESIAN_POINT('Ctrl Pts',(0.751562963361383,-1.,-2.03814160092173));
#24375=CARTESIAN_POINT('Ctrl Pts',(0.752642180488104,-1.,-2.03182068456467));
#24376=CARTESIAN_POINT('Ctrl Pts',(0.753682061113765,-1.,-2.02550428623587));
#24377=CARTESIAN_POINT('Ctrl Pts',(0.75468233072352,-1.,-2.01919259406003));
#24378=CARTESIAN_POINT('Ctrl Pts',(0.7556427049581,-1.,-2.01288584328149));
#24379=CARTESIAN_POINT('Ctrl Pts',(0.756562904646496,-1.,-2.00658431587682));
#24380=CARTESIAN_POINT('Ctrl Pts',(0.757442676862341,-1.,-2.00028834739072));
#24381=CARTESIAN_POINT('Ctrl Pts',(0.758281796766377,-1.,-1.9939983109871));
#24382=CARTESIAN_POINT('Ctrl Pts',(0.759080037802242,-1.,-1.98771456680806));
#24383=CARTESIAN_POINT('Ctrl Pts',(0.759837147452135,-1.,-1.98143741418156));
#24384=CARTESIAN_POINT('Ctrl Pts',(0.760552825409855,-1.,-1.97516705321521));
#24385=CARTESIAN_POINT('Ctrl Pts',(0.761226690483986,-1.,-1.96890351582545));
#24386=CARTESIAN_POINT('Ctrl Pts',(0.761858300014575,-1.,-1.96264672744229));
#24387=CARTESIAN_POINT('Ctrl Pts',(0.762447203806263,-1.,-1.95639665309893));
#24388=CARTESIAN_POINT('Ctrl Pts',(0.762992990878774,-1.,-1.95015342590025));
#24389=CARTESIAN_POINT('Ctrl Pts',(0.76349533353858,-1.,-1.94391746617626));
#24390=CARTESIAN_POINT('Ctrl Pts',(0.763954049121393,-1.,-1.93768964875867));
#24391=CARTESIAN_POINT('Ctrl Pts',(0.764369010673889,-1.,-1.93147105496367));
#24392=CARTESIAN_POINT('Ctrl Pts',(0.764740025488189,-1.,-1.92526263537041));
#24393=CARTESIAN_POINT('Ctrl Pts',(0.765066729667095,-1.,-1.91906491634197));
#24394=CARTESIAN_POINT('Ctrl Pts',(0.765348465884739,-1.,-1.91287765805174));
#24395=CARTESIAN_POINT('Ctrl Pts',(0.765584196937936,-1.,-1.90669961402362));
#24396=CARTESIAN_POINT('Ctrl Pts',(0.765772772593395,-1.,-1.90052930393599));
#24397=CARTESIAN_POINT('Ctrl Pts',(0.765913193856979,-1.,-1.89436577771389));
#24398=CARTESIAN_POINT('Ctrl Pts',(0.76600483706209,-1.,-1.88820926433409));
#24399=CARTESIAN_POINT('Ctrl Pts',(0.766047794851868,-1.,-1.88206215302561));
#24400=CARTESIAN_POINT('Ctrl Pts',(0.766042837036759,-1.,-1.87592888967886));
#24401=CARTESIAN_POINT('Ctrl Pts',(0.765990708546111,-1.,-1.86981398314345));
#24402=CARTESIAN_POINT('Ctrl Pts',(0.765891519092557,-1.,-1.86372027063315));
#24403=CARTESIAN_POINT('Ctrl Pts',(0.765744212909305,-1.,-1.85764741390391));
#24404=CARTESIAN_POINT('Ctrl Pts',(0.765545710619023,-1.,-1.85158945130054));
#24405=CARTESIAN_POINT('Ctrl Pts',(0.765291664861971,-1.,-1.84553698875911));
#24406=CARTESIAN_POINT('Ctrl Pts',(0.764978057881687,-1.,-1.83948181064823));
#24407=CARTESIAN_POINT('Ctrl Pts',(0.764602549687845,-1.,-1.8334207722714));
#24408=CARTESIAN_POINT('Ctrl Pts',(0.764165902606055,-1.,-1.8273599120008));
#24409=CARTESIAN_POINT('Ctrl Pts',(0.763673465462854,-1.,-1.82131873145297));
#24410=CARTESIAN_POINT('Ctrl Pts',(0.763132003836783,-1.,-1.81532118405566));
#24411=CARTESIAN_POINT('Ctrl Pts',(0.762546129464036,-1.,-1.80938551463989));
#24412=CARTESIAN_POINT('Ctrl Pts',(0.761915336443515,-1.,-1.80351583877334));
#24413=CARTESIAN_POINT('Ctrl Pts',(0.761229695230359,-1.,-1.79768986997735));
#24414=CARTESIAN_POINT('Ctrl Pts',(0.760469555880425,-1.,-1.79185815610802));
#24415=CARTESIAN_POINT('Ctrl Pts',(0.759614401109868,-1.,-1.78596964884527));
#24416=CARTESIAN_POINT('Ctrl Pts',(0.75865062667738,-1.,-1.77999411220912));
#24417=CARTESIAN_POINT('Ctrl Pts',(0.757578264077238,-1.,-1.77394167108342));
#24418=CARTESIAN_POINT('Ctrl Pts',(0.756421896028403,-1.,-1.76789396003141));
#24419=CARTESIAN_POINT('Ctrl Pts',(0.755220979975262,-1.,-1.7619781724032));
#24420=CARTESIAN_POINT('Ctrl Pts',(0.75400925402848,-1.,-1.75631083600175));
#24421=CARTESIAN_POINT('Ctrl Pts',(0.752797683531377,-1.,-1.75095139468809));
#24422=CARTESIAN_POINT('Ctrl Pts',(0.751555614163629,-1.,-1.74585086852298));
#24423=CARTESIAN_POINT('Ctrl Pts',(0.75019343597954,-1.,-1.74080458266705));
#24424=CARTESIAN_POINT('Ctrl Pts',(0.748582462954854,-1.,-1.73550351679848));
#24425=CARTESIAN_POINT('Ctrl Pts',(0.746574710096436,-1.,-1.72958533647399));
#24426=CARTESIAN_POINT('Ctrl Pts',(0.744021445433764,-1.,-1.7226822991693));
#24427=CARTESIAN_POINT('Ctrl Pts',(0.740795162032087,-1.,-1.71447789751927));
#24428=CARTESIAN_POINT('Ctrl Pts',(0.736799665724771,-1.,-1.70473309006121));
#24429=CARTESIAN_POINT('Ctrl Pts',(0.731963238697195,-1.,-1.69326921975743));
#24430=CARTESIAN_POINT('Ctrl Pts',(0.726235967997433,-1.,-1.67996158455503));
#24431=CARTESIAN_POINT('Ctrl Pts',(0.719585433804282,-1.,-1.6647288055568));
#24432=CARTESIAN_POINT('Ctrl Pts',(0.711993139355394,-1.,-1.64752408832016));
#24433=CARTESIAN_POINT('Ctrl Pts',(0.705159151988319,-1.,-1.63216541664676));
#24434=CARTESIAN_POINT('Ctrl Pts',(0.699605146405088,-1.,-1.61974673472612));
#24435=CARTESIAN_POINT('Ctrl Pts',(0.695712097881194,-1.,-1.61106790958151));
#24436=CARTESIAN_POINT('Ctrl Pts',(0.693717979106306,-1.,-1.60662857109684));
#24437=CARTESIAN_POINT('',(0.892032620296855,-1.,-1.5055822144029));
#24438=CARTESIAN_POINT('Origin',(0.,-1.,0.));
#24439=CARTESIAN_POINT('',(1.23627494547115,-1.,-1.81978687191668));
#24440=CARTESIAN_POINT('Ctrl Pts',(0.892032620296855,-1.,-1.5055822144029));
#24441=CARTESIAN_POINT('Ctrl Pts',(0.894452006964543,-1.,-1.50980486806688));
#24442=CARTESIAN_POINT('Ctrl Pts',(0.89918504748351,-1.,-1.51805569590094));
#24443=CARTESIAN_POINT('Ctrl Pts',(0.905967409625651,-1.,-1.52984849887993));
#24444=CARTESIAN_POINT('Ctrl Pts',(0.914375919026456,-1.,-1.54440491149498));
#24445=CARTESIAN_POINT('Ctrl Pts',(0.923832188944341,-1.,-1.56065988578893));
#24446=CARTESIAN_POINT('Ctrl Pts',(0.932246680108685,-1.,-1.57499388382243));
#24447=CARTESIAN_POINT('Ctrl Pts',(0.939646377893399,-1.,-1.58744937487176));
#24448=CARTESIAN_POINT('Ctrl Pts',(0.946078063315257,-1.,-1.59810042043673));
#24449=CARTESIAN_POINT('Ctrl Pts',(0.951613284356035,-1.,-1.60706069896936));
#24450=CARTESIAN_POINT('Ctrl Pts',(0.95635442292067,-1.,-1.61449324337085));
#24451=CARTESIAN_POINT('Ctrl Pts',(0.960438326101728,-1.,-1.62061638140221));
#24452=CARTESIAN_POINT('Ctrl Pts',(0.964046107040535,-1.,-1.62571930670187));
#24453=CARTESIAN_POINT('Ctrl Pts',(0.967387853230345,-1.,-1.63013849959462));
#24454=CARTESIAN_POINT('Ctrl Pts',(0.970669715997509,-1.,-1.63420665729798));
#24455=CARTESIAN_POINT('Ctrl Pts',(0.974066058287418,-1.,-1.63820952658144));
#24456=CARTESIAN_POINT('Ctrl Pts',(0.977689794119416,-1.,-1.64233990826687));
#24457=CARTESIAN_POINT('Ctrl Pts',(0.981562530939489,-1.,-1.64665139190656));
#24458=CARTESIAN_POINT('Ctrl Pts',(0.98564262292082,-1.,-1.65110016612638));
#24459=CARTESIAN_POINT('Ctrl Pts',(0.989855627854164,-1.,-1.65559044289699));
#24460=CARTESIAN_POINT('Ctrl Pts',(0.994121836661305,-1.,-1.66001553809947));
#24461=CARTESIAN_POINT('Ctrl Pts',(0.998389654952757,-1.,-1.66430758030376));
#24462=CARTESIAN_POINT('Ctrl Pts',(1.00265091003727,-1.,-1.66846059277303));
#24463=CARTESIAN_POINT('Ctrl Pts',(1.00692206696414,-1.,-1.67250335383293));
#24464=CARTESIAN_POINT('Ctrl Pts',(1.01123236493511,-1.,-1.67648246776464));
#24465=CARTESIAN_POINT('Ctrl Pts',(1.01561026162773,-1.,-1.68044289894798));
#24466=CARTESIAN_POINT('Ctrl Pts',(1.02006795074201,-1.,-1.68440578021706));
#24467=CARTESIAN_POINT('Ctrl Pts',(1.02460180535255,-1.,-1.68836910178447));
#24468=CARTESIAN_POINT('Ctrl Pts',(1.02919977579147,-1.,-1.69231840863458));
#24469=CARTESIAN_POINT('Ctrl Pts',(1.03384646003588,-1.,-1.69623414782771));
#24470=CARTESIAN_POINT('Ctrl Pts',(1.03852922490789,-1.,-1.70010052930962));
#24471=CARTESIAN_POINT('Ctrl Pts',(1.04324363334554,-1.,-1.70391338707982));
#24472=CARTESIAN_POINT('Ctrl Pts',(1.04799085404995,-1.,-1.70767646263649));
#24473=CARTESIAN_POINT('Ctrl Pts',(1.05277517202855,-1.,-1.71139783543989));
#24474=CARTESIAN_POINT('Ctrl Pts',(1.05760163192479,-1.,-1.7150865442702));
#24475=CARTESIAN_POINT('Ctrl Pts',(1.06247324680647,-1.,-1.71874858456904));
#24476=CARTESIAN_POINT('Ctrl Pts',(1.06738966975462,-1.,-1.72238500928453));
#24477=CARTESIAN_POINT('Ctrl Pts',(1.07234866990252,-1.,-1.72599406198488));
#24478=CARTESIAN_POINT('Ctrl Pts',(1.0773470373727,-1.,-1.72957248977424));
#24479=CARTESIAN_POINT('Ctrl Pts',(1.08238162784749,-1.,-1.73311705663407));
#24480=CARTESIAN_POINT('Ctrl Pts',(1.08745056285427,-1.,-1.73662628326091));
#24481=CARTESIAN_POINT('Ctrl Pts',(1.09255329056493,-1.,-1.74010053962247));
#24482=CARTESIAN_POINT('Ctrl Pts',(1.09768999241225,-1.,-1.74354119236208));
#24483=CARTESIAN_POINT('Ctrl Pts',(1.10286118991143,-1.,-1.74695004214923));
#24484=CARTESIAN_POINT('Ctrl Pts',(1.10806728183007,-1.,-1.7503286607592));
#24485=CARTESIAN_POINT('Ctrl Pts',(1.11330807582551,-1.,-1.7536777209463));
#24486=CARTESIAN_POINT('Ctrl Pts',(1.11858293216763,-1.,-1.75699720772105));
#24487=CARTESIAN_POINT('Ctrl Pts',(1.12389096855086,-1.,-1.76028671825096));
#24488=CARTESIAN_POINT('Ctrl Pts',(1.12923123555075,-1.,-1.7635457196617));
#24489=CARTESIAN_POINT('Ctrl Pts',(1.1346029180462,-1.,-1.76677384551862));
#24490=CARTESIAN_POINT('Ctrl Pts',(1.14000548336975,-1.,-1.76997111386769));
#24491=CARTESIAN_POINT('Ctrl Pts',(1.1454385822692,-1.,-1.77313777896194));
#24492=CARTESIAN_POINT('Ctrl Pts',(1.15090197841514,-1.,-1.7762742255701));
#24493=CARTESIAN_POINT('Ctrl Pts',(1.15639547194698,-1.,-1.77938085564275));
#24494=CARTESIAN_POINT('Ctrl Pts',(1.16191881298499,-1.,-1.78245795881009));
#24495=CARTESIAN_POINT('Ctrl Pts',(1.16747166312303,-1.,-1.78550566040443));
#24496=CARTESIAN_POINT('Ctrl Pts',(1.17305363177328,-1.,-1.78852398877617));
#24497=CARTESIAN_POINT('Ctrl Pts',(1.17866429440809,-1.,-1.79151291552689));
#24498=CARTESIAN_POINT('Ctrl Pts',(1.18430321697432,-1.,-1.79447240321515));
#24499=CARTESIAN_POINT('Ctrl Pts',(1.18996997934445,-1.,-1.79740245923478));
#24500=CARTESIAN_POINT('Ctrl Pts',(1.19566418930242,-1.,-1.80030314369879));
#24501=CARTESIAN_POINT('Ctrl Pts',(1.20138548938974,-1.,-1.80317454838603));
#24502=CARTESIAN_POINT('Ctrl Pts',(1.20713356605475,-1.,-1.80601678480707));
#24503=CARTESIAN_POINT('Ctrl Pts',(1.21290815708314,-1.,-1.80882996917129));
#24504=CARTESIAN_POINT('Ctrl Pts',(1.21870906103557,-1.,-1.81161420806656));
#24505=CARTESIAN_POINT('Ctrl Pts',(1.2245361330495,-1.,-1.81436959210434));
#24506=CARTESIAN_POINT('Ctrl Pts',(1.2292186489137,-1.,-1.8165508718364));
#24507=CARTESIAN_POINT('Ctrl Pts',(1.2327422452705,-1.,-1.81817389921279));
#24508=CARTESIAN_POINT('Ctrl Pts',(1.23509651170476,-1.,-1.81925017193666));
#24509=CARTESIAN_POINT('Ctrl Pts',(1.23627494547115,-1.,-1.81978687191668));
#24510=CARTESIAN_POINT('',(1.34869019493419,-1.,-1.73811241238545));
#24511=CARTESIAN_POINT('',(1.23627494547115,-1.,-1.81978687191668));
#24512=CARTESIAN_POINT('',(1.15624053661742,-1.,-1.31362392696032));
#24513=CARTESIAN_POINT('Ctrl Pts',(1.34869019493419,-1.,-1.73811241238545));
#24514=CARTESIAN_POINT('Ctrl Pts',(1.34854391898045,-1.,-1.73682580585691));
#24515=CARTESIAN_POINT('Ctrl Pts',(1.34824783112887,-1.,-1.73425417885907));
#24516=CARTESIAN_POINT('Ctrl Pts',(1.34779309152035,-1.,-1.7304014965394));
#24517=CARTESIAN_POINT('Ctrl Pts',(1.34716554819527,-1.,-1.72527410680674));
#24518=CARTESIAN_POINT('Ctrl Pts',(1.34634568653227,-1.,-1.7188807715049));
#24519=CARTESIAN_POINT('Ctrl Pts',(1.34549029589416,-1.,-1.71250340686822));
#24520=CARTESIAN_POINT('Ctrl Pts',(1.34459924533831,-1.,-1.70614212266738));
#24521=CARTESIAN_POINT('Ctrl Pts',(1.34367237124483,-1.,-1.69979707754427));
#24522=CARTESIAN_POINT('Ctrl Pts',(1.34270948206319,-1.,-1.6934684849687));
#24523=CARTESIAN_POINT('Ctrl Pts',(1.341710374848,-1.,-1.68715660868764));
#24524=CARTESIAN_POINT('Ctrl Pts',(1.34067485185203,-1.,-1.68086176030362));
#24525=CARTESIAN_POINT('Ctrl Pts',(1.3396027347034,-1.,-1.67458429426086));
#24526=CARTESIAN_POINT('Ctrl Pts',(1.33849388654388,-1.,-1.66832460783989));
#24527=CARTESIAN_POINT('Ctrl Pts',(1.33734820885262,-1.,-1.66208312541983));
#24528=CARTESIAN_POINT('Ctrl Pts',(1.33616559745172,-1.,-1.65586025952593));
#24529=CARTESIAN_POINT('Ctrl Pts',(1.33494590467993,-1.,-1.6496563728683));
#24530=CARTESIAN_POINT('Ctrl Pts',(1.33368890676572,-1.,-1.6434717485603));
#24531=CARTESIAN_POINT('Ctrl Pts',(1.33239425103724,-1.,-1.63730653475089));
#24532=CARTESIAN_POINT('Ctrl Pts',(1.33106149345645,-1.,-1.63116079730923));
#24533=CARTESIAN_POINT('Ctrl Pts',(1.3296901950568,-1.,-1.62503464209797));
#24534=CARTESIAN_POINT('Ctrl Pts',(1.32828000610449,-1.,-1.61892832270724));
#24535=CARTESIAN_POINT('Ctrl Pts',(1.32683074483356,-1.,-1.6128423401575));
#24536=CARTESIAN_POINT('Ctrl Pts',(1.32534250785782,-1.,-1.60677758290954));
#24537=CARTESIAN_POINT('Ctrl Pts',(1.32381550858256,-1.,-1.60073511858687));
#24538=CARTESIAN_POINT('Ctrl Pts',(1.32224985747682,-1.,-1.59471591079403));
#24539=CARTESIAN_POINT('Ctrl Pts',(1.32064537110892,-1.,-1.58872057258245));
#24540=CARTESIAN_POINT('Ctrl Pts',(1.31900135021432,-1.,-1.58274907898834));
#24541=CARTESIAN_POINT('Ctrl Pts',(1.31731642317187,-1.,-1.5768005650559));
#24542=CARTESIAN_POINT('Ctrl Pts',(1.31558903860016,-1.,-1.57087397835723));
#24543=CARTESIAN_POINT('Ctrl Pts',(1.31381795281002,-1.,-1.56496872402353));
#24544=CARTESIAN_POINT('Ctrl Pts',(1.31200264341696,-1.,-1.55908521254821));
#24545=CARTESIAN_POINT('Ctrl Pts',(1.31014393684222,-1.,-1.55322568759481));
#24546=CARTESIAN_POINT('Ctrl Pts',(1.30824393907473,-1.,-1.54739413957185));
#24547=CARTESIAN_POINT('Ctrl Pts',(1.30630475189556,-1.,-1.54159462645432));
#24548=CARTESIAN_POINT('Ctrl Pts',(1.30432735639489,-1.,-1.53582981268977));
#24549=CARTESIAN_POINT('Ctrl Pts',(1.30231064395568,-1.,-1.53009970283891));
#24550=CARTESIAN_POINT('Ctrl Pts',(1.30024984366328,-1.,-1.52439957861062));
#24551=CARTESIAN_POINT('Ctrl Pts',(1.29813791800747,-1.,-1.51872184912724));
#24552=CARTESIAN_POINT('Ctrl Pts',(1.29596850710509,-1.,-1.51305994241402));
#24553=CARTESIAN_POINT('Ctrl Pts',(1.29373841372842,-1.,-1.50741159078365));
#24554=CARTESIAN_POINT('Ctrl Pts',(1.29145022885181,-1.,-1.50178230149776));
#24555=CARTESIAN_POINT('Ctrl Pts',(1.28911506584254,-1.,-1.49618896881754));
#24556=CARTESIAN_POINT('Ctrl Pts',(1.2867467611644,-1.,-1.4906522831278));
#24557=CARTESIAN_POINT('Ctrl Pts',(1.28435533880201,-1.,-1.4851881711891));
#24558=CARTESIAN_POINT('Ctrl Pts',(1.28194158939517,-1.,-1.47980070347096));
#24559=CARTESIAN_POINT('Ctrl Pts',(1.2794891824849,-1.,-1.4744717526707));
#24560=CARTESIAN_POINT('Ctrl Pts',(1.27696414831089,-1.,-1.46916035917133));
#24561=CARTESIAN_POINT('Ctrl Pts',(1.27433119897822,-1.,-1.46382431332476));
#24562=CARTESIAN_POINT('Ctrl Pts',(1.27156805265289,-1.,-1.45843906294697));
#24563=CARTESIAN_POINT('Ctrl Pts',(1.2686778680489,-1.,-1.45301422764247));
#24564=CARTESIAN_POINT('Ctrl Pts',(1.26570925118868,-1.,-1.44761985001662));
#24565=CARTESIAN_POINT('Ctrl Pts',(1.26273903323858,-1.,-1.44236470511303));
#24566=CARTESIAN_POINT('Ctrl Pts',(1.25983531012005,-1.,-1.43734919180848));
#24567=CARTESIAN_POINT('Ctrl Pts',(1.25702687965755,-1.,-1.43262645609691));
#24568=CARTESIAN_POINT('Ctrl Pts',(1.25426945222639,-1.,-1.42815938799387));
#24569=CARTESIAN_POINT('Ctrl Pts',(1.2514145557001,-1.,-1.42378102115575));
#24570=CARTESIAN_POINT('Ctrl Pts',(1.24824430986571,-1.,-1.41923722596025));
#24571=CARTESIAN_POINT('Ctrl Pts',(1.24450600513056,-1.,-1.41422913175179));
#24572=CARTESIAN_POINT('Ctrl Pts',(1.23994455029534,-1.,-1.40845295531283));
#24573=CARTESIAN_POINT('Ctrl Pts',(1.23434087290423,-1.,-1.40164708206106));
#24574=CARTESIAN_POINT('Ctrl Pts',(1.22752961899387,-1.,-1.39361389568796));
#24575=CARTESIAN_POINT('Ctrl Pts',(1.21938737280852,-1.,-1.38420564527715));
#24576=CARTESIAN_POINT('Ctrl Pts',(1.20982812925645,-1.,-1.37331915607905));
#24577=CARTESIAN_POINT('Ctrl Pts',(1.1987959077932,-1.,-1.36088705043885));
#24578=CARTESIAN_POINT('Ctrl Pts',(1.18625865667441,-1.,-1.34687054001093));
#24579=CARTESIAN_POINT('Ctrl Pts',(1.17501305789857,-1.,-1.33437539347008));
#24580=CARTESIAN_POINT('Ctrl Pts',(1.16589330093588,-1.,-1.32428080721772));
#24581=CARTESIAN_POINT('Ctrl Pts',(1.15950888730809,-1.,-1.31722977216397));
#24582=CARTESIAN_POINT('Ctrl Pts',(1.15624053661742,-1.,-1.31362392696032));
#24583=CARTESIAN_POINT('',(1.31362392696032,-1.,-1.15624053661742));
#24584=CARTESIAN_POINT('Origin',(0.,-1.,0.));
#24585=CARTESIAN_POINT('',(1.73811241238545,-1.,-1.34869019493419));
#24586=CARTESIAN_POINT('Ctrl Pts',(1.31362392696032,-1.,-1.15624053661742));
#24587=CARTESIAN_POINT('Ctrl Pts',(1.3172297721596,-1.,-1.15950888730433));
#24588=CARTESIAN_POINT('Ctrl Pts',(1.32428080720544,-1.,-1.16589330092532));
#24589=CARTESIAN_POINT('Ctrl Pts',(1.33437539344842,-1.,-1.17501305787994));
#24590=CARTESIAN_POINT('Ctrl Pts',(1.34687053998157,-1.,-1.18625865664915));
#24591=CARTESIAN_POINT('Ctrl Pts',(1.36088705040677,-1.,-1.1987959077656));
#24592=CARTESIAN_POINT('Ctrl Pts',(1.37331915604962,-1.,-1.20982812923113));
#24593=CARTESIAN_POINT('Ctrl Pts',(1.38420564525391,-1.,-1.21938737278853));
#24594=CARTESIAN_POINT('Ctrl Pts',(1.39361389567257,-1.,-1.22752961898063));
#24595=CARTESIAN_POINT('Ctrl Pts',(1.40164708205345,-1.,-1.23434087289768));
#24596=CARTESIAN_POINT('Ctrl Pts',(1.40845295531151,-1.,-1.23994455029421));
#24597=CARTESIAN_POINT('Ctrl Pts',(1.41422913175437,-1.,-1.24450600513278));
#24598=CARTESIAN_POINT('Ctrl Pts',(1.41923722596421,-1.,-1.24824430986911));
#24599=CARTESIAN_POINT('Ctrl Pts',(1.42378102115911,-1.,-1.25141455570299));
#24600=CARTESIAN_POINT('Ctrl Pts',(1.42815938799555,-1.,-1.25426945222783));
#24601=CARTESIAN_POINT('Ctrl Pts',(1.43262645609679,-1.,-1.25702687965744));
#24602=CARTESIAN_POINT('Ctrl Pts',(1.43734919180719,-1.,-1.25983531011894));
#24603=CARTESIAN_POINT('Ctrl Pts',(1.44236470511145,-1.,-1.26273903323723));
#24604=CARTESIAN_POINT('Ctrl Pts',(1.44761985001544,-1.,-1.26570925118767));
#24605=CARTESIAN_POINT('Ctrl Pts',(1.45301422764205,-1.,-1.26867786804854));
#24606=CARTESIAN_POINT('Ctrl Pts',(1.45843906294725,-1.,-1.27156805265312));
#24607=CARTESIAN_POINT('Ctrl Pts',(1.4638243133254,-1.,-1.27433119897877));
#24608=CARTESIAN_POINT('Ctrl Pts',(1.46916035917197,-1.,-1.27696414831144));
#24609=CARTESIAN_POINT('Ctrl Pts',(1.4744717526711,-1.,-1.27948918248524));
#24610=CARTESIAN_POINT('Ctrl Pts',(1.47980070347102,-1.,-1.28194158939522));
#24611=CARTESIAN_POINT('Ctrl Pts',(1.48518817118891,-1.,-1.28435533880184));
#24612=CARTESIAN_POINT('Ctrl Pts',(1.4906522831275,-1.,-1.28674676116415));
#24613=CARTESIAN_POINT('Ctrl Pts',(1.49618896881729,-1.,-1.28911506584232));
#24614=CARTESIAN_POINT('Ctrl Pts',(1.50178230149764,-1.,-1.29145022885171));
#24615=CARTESIAN_POINT('Ctrl Pts',(1.50741159078367,-1.,-1.29373841372843));
#24616=CARTESIAN_POINT('Ctrl Pts',(1.51305994241412,-1.,-1.29596850710518));
#24617=CARTESIAN_POINT('Ctrl Pts',(1.51872184912735,-1.,-1.29813791800757));
#24618=CARTESIAN_POINT('Ctrl Pts',(1.5243995786107,-1.,-1.30024984366334));
#24619=CARTESIAN_POINT('Ctrl Pts',(1.53009970283893,-1.,-1.3023106439557));
#24620=CARTESIAN_POINT('Ctrl Pts',(1.53582981268976,-1.,-1.30432735639487));
#24621=CARTESIAN_POINT('Ctrl Pts',(1.54159462645428,-1.,-1.30630475189553));
#24622=CARTESIAN_POINT('Ctrl Pts',(1.54739413957183,-1.,-1.30824393907471));
#24623=CARTESIAN_POINT('Ctrl Pts',(1.55322568759481,-1.,-1.31014393684221));
#24624=CARTESIAN_POINT('Ctrl Pts',(1.55908521254822,-1.,-1.31200264341696));
#24625=CARTESIAN_POINT('Ctrl Pts',(1.56496872402352,-1.,-1.31381795281002));
#24626=CARTESIAN_POINT('Ctrl Pts',(1.57087397835721,-1.,-1.31558903860015));
#24627=CARTESIAN_POINT('Ctrl Pts',(1.57680056505585,-1.,-1.31731642317183));
#24628=CARTESIAN_POINT('Ctrl Pts',(1.58274907898829,-1.,-1.31900135021428));
#24629=CARTESIAN_POINT('Ctrl Pts',(1.58872057258244,-1.,-1.32064537110891));
#24630=CARTESIAN_POINT('Ctrl Pts',(1.59471591079408,-1.,-1.32224985747686));
#24631=CARTESIAN_POINT('Ctrl Pts',(1.600735118587,-1.,-1.32381550858266));
#24632=CARTESIAN_POINT('Ctrl Pts',(1.6067775829097,-1.,-1.32534250785794));
#24633=CARTESIAN_POINT('Ctrl Pts',(1.61284234015762,-1.,-1.32683074483365));
#24634=CARTESIAN_POINT('Ctrl Pts',(1.61892832270723,-1.,-1.32828000610448));
#24635=CARTESIAN_POINT('Ctrl Pts',(1.62503464209777,-1.,-1.32969019505665));
#24636=CARTESIAN_POINT('Ctrl Pts',(1.63116079730887,-1.,-1.33106149345618));
#24637=CARTESIAN_POINT('Ctrl Pts',(1.63730653475049,-1.,-1.33239425103694));
#24638=CARTESIAN_POINT('Ctrl Pts',(1.64347174856007,-1.,-1.33368890676554));
#24639=CARTESIAN_POINT('Ctrl Pts',(1.64965637286843,-1.,-1.33494590468003));
#24640=CARTESIAN_POINT('Ctrl Pts',(1.65586025952651,-1.,-1.33616559745217));
#24641=CARTESIAN_POINT('Ctrl Pts',(1.66208312542073,-1.,-1.33734820885331));
#24642=CARTESIAN_POINT('Ctrl Pts',(1.66832460784078,-1.,-1.33849388654458));
#24643=CARTESIAN_POINT('Ctrl Pts',(1.67458429426126,-1.,-1.33960273470372));
#24644=CARTESIAN_POINT('Ctrl Pts',(1.68086176030308,-1.,-1.3406748518516));
#24645=CARTESIAN_POINT('Ctrl Pts',(1.68715660868602,-1.,-1.34171037484673));
#24646=CARTESIAN_POINT('Ctrl Pts',(1.6934684849664,-1.,-1.34270948206139));
#24647=CARTESIAN_POINT('Ctrl Pts',(1.69979707754221,-1.,-1.34367237124322));
#24648=CARTESIAN_POINT('Ctrl Pts',(1.70614212266676,-1.,-1.34459924533783));
#24649=CARTESIAN_POINT('Ctrl Pts',(1.71250340687011,-1.,-1.34549029589563));
#24650=CARTESIAN_POINT('Ctrl Pts',(1.7188807715095,-1.,-1.34634568653586));
#24651=CARTESIAN_POINT('Ctrl Pts',(1.72527410681298,-1.,-1.34716554820013));
#24652=CARTESIAN_POINT('Ctrl Pts',(1.73040149654497,-1.,-1.3477930915247));
#24653=CARTESIAN_POINT('Ctrl Pts',(1.73425417886254,-1.,-1.34824783113158));
#24654=CARTESIAN_POINT('Ctrl Pts',(1.73682580585819,-1.,-1.34854391898145));
#24655=CARTESIAN_POINT('Ctrl Pts',(1.73811241238545,-1.,-1.34869019493419));
#24656=CARTESIAN_POINT('',(1.81978687191668,-1.,-1.23627494547115));
#24657=CARTESIAN_POINT('',(1.73811241238545,-1.,-1.34869019493419));
#24658=CARTESIAN_POINT('',(1.5055822144029,-1.,-0.892032620296855));
#24659=CARTESIAN_POINT('Ctrl Pts',(1.81978687191668,-1.,-1.23627494547115));
#24660=CARTESIAN_POINT('Ctrl Pts',(1.81925017193531,-1.,-1.23509651170384));
#24661=CARTESIAN_POINT('Ctrl Pts',(1.81817389920914,-1.,-1.23274224526804));
#24662=CARTESIAN_POINT('Ctrl Pts',(1.81655087183054,-1.,-1.22921864890975));
#24663=CARTESIAN_POINT('Ctrl Pts',(1.81436959209778,-1.,-1.22453613304507));
#24664=CARTESIAN_POINT('Ctrl Pts',(1.81161420806172,-1.,-1.2187090610323));
#24665=CARTESIAN_POINT('Ctrl Pts',(1.80882996916931,-1.,-1.2129081570818));
#24666=CARTESIAN_POINT('Ctrl Pts',(1.80601678480772,-1.,-1.20713356605519));
#24667=CARTESIAN_POINT('Ctrl Pts',(1.8031745483882,-1.,-1.2013854893912));
#24668=CARTESIAN_POINT('Ctrl Pts',(1.80030314370121,-1.,-1.19566418930405));
#24669=CARTESIAN_POINT('Ctrl Pts',(1.79740245923649,-1.,-1.1899699793456));
#24670=CARTESIAN_POINT('Ctrl Pts',(1.79447240321572,-1.,-1.18430321697471));
#24671=CARTESIAN_POINT('Ctrl Pts',(1.79151291552646,-1.,-1.17866429440781));
#24672=CARTESIAN_POINT('Ctrl Pts',(1.78852398877523,-1.,-1.17305363177265));
#24673=CARTESIAN_POINT('Ctrl Pts',(1.78550566040349,-1.,-1.16747166312239));
#24674=CARTESIAN_POINT('Ctrl Pts',(1.78245795880949,-1.,-1.16191881298458));
#24675=CARTESIAN_POINT('Ctrl Pts',(1.77938085564261,-1.,-1.15639547194689));
#24676=CARTESIAN_POINT('Ctrl Pts',(1.77627422557034,-1.,-1.15090197841531));
#24677=CARTESIAN_POINT('Ctrl Pts',(1.77313777896234,-1.,-1.14543858226948));
#24678=CARTESIAN_POINT('Ctrl Pts',(1.76997111386806,-1.,-1.14000548337));
#24679=CARTESIAN_POINT('Ctrl Pts',(1.76677384551883,-1.,-1.13460291804635));
#24680=CARTESIAN_POINT('Ctrl Pts',(1.76354571966171,-1.,-1.12923123555076));
#24681=CARTESIAN_POINT('Ctrl Pts',(1.76028671825084,-1.,-1.12389096855078));
#24682=CARTESIAN_POINT('Ctrl Pts',(1.75699720772089,-1.,-1.11858293216752));
#24683=CARTESIAN_POINT('Ctrl Pts',(1.75367772094617,-1.,-1.11330807582542));
#24684=CARTESIAN_POINT('Ctrl Pts',(1.75032866075914,-1.,-1.10806728183003));
#24685=CARTESIAN_POINT('Ctrl Pts',(1.74695004214924,-1.,-1.10286118991144));
#24686=CARTESIAN_POINT('Ctrl Pts',(1.74354119236212,-1.,-1.09768999241229));
#24687=CARTESIAN_POINT('Ctrl Pts',(1.74010053962252,-1.,-1.09255329056496));
#24688=CARTESIAN_POINT('Ctrl Pts',(1.73662628326093,-1.,-1.08745056285429));
#24689=CARTESIAN_POINT('Ctrl Pts',(1.73311705663407,-1.,-1.08238162784749));
#24690=CARTESIAN_POINT('Ctrl Pts',(1.72957248977424,-1.,-1.0773470373727));
#24691=CARTESIAN_POINT('Ctrl Pts',(1.72599406198489,-1.,-1.07234866990252));
#24692=CARTESIAN_POINT('Ctrl Pts',(1.72238500928456,-1.,-1.06738966975463));
#24693=CARTESIAN_POINT('Ctrl Pts',(1.71874858456908,-1.,-1.0624732468065));
#24694=CARTESIAN_POINT('Ctrl Pts',(1.71508654427022,-1.,-1.05760163192481));
#24695=CARTESIAN_POINT('Ctrl Pts',(1.71139783543986,-1.,-1.05277517202854));
#24696=CARTESIAN_POINT('Ctrl Pts',(1.70767646263641,-1.,-1.0479908540499));
#24697=CARTESIAN_POINT('Ctrl Pts',(1.70391338707969,-1.,-1.04324363334546));
#24698=CARTESIAN_POINT('Ctrl Pts',(1.70010052930951,-1.,-1.03852922490782));
#24699=CARTESIAN_POINT('Ctrl Pts',(1.69623414782769,-1.,-1.03384646003587));
#24700=CARTESIAN_POINT('Ctrl Pts',(1.69231840863471,-1.,-1.02919977579155));
#24701=CARTESIAN_POINT('Ctrl Pts',(1.68836910178475,-1.,-1.02460180535272));
#24702=CARTESIAN_POINT('Ctrl Pts',(1.68440578021739,-1.,-1.02006795074222));
#24703=CARTESIAN_POINT('Ctrl Pts',(1.6804428989482,-1.,-1.01561026162787));
#24704=CARTESIAN_POINT('Ctrl Pts',(1.67648246776457,-1.,-1.01123236493507));
#24705=CARTESIAN_POINT('Ctrl Pts',(1.67250335383248,-1.,-1.00692206696387));
#24706=CARTESIAN_POINT('Ctrl Pts',(1.66846059277231,-1.,-1.00265091003682));
#24707=CARTESIAN_POINT('Ctrl Pts',(1.66430758030304,-1.,-0.998389654952317));
#24708=CARTESIAN_POINT('Ctrl Pts',(1.66001553809916,-1.,-0.994121836661116));
#24709=CARTESIAN_POINT('Ctrl Pts',(1.65559044289746,-1.,-0.98985562785445));
#24710=CARTESIAN_POINT('Ctrl Pts',(1.6511001661277,-1.,-0.985642622921626));
#24711=CARTESIAN_POINT('Ctrl Pts',(1.64665139190834,-1.,-0.981562530940574));
#24712=CARTESIAN_POINT('Ctrl Pts',(1.64233990826831,-1.,-0.977689794120297));
#24713=CARTESIAN_POINT('Ctrl Pts',(1.63820952658157,-1.,-0.974066058287501));
#24714=CARTESIAN_POINT('Ctrl Pts',(1.63420665729609,-1.,-0.970669715996356));
#24715=CARTESIAN_POINT('Ctrl Pts',(1.63013849959083,-1.,-0.967387853228041));
#24716=CARTESIAN_POINT('Ctrl Pts',(1.6257193066974,-1.,-0.964046107037821));
#24717=CARTESIAN_POINT('Ctrl Pts',(1.62061638139929,-1.,-0.960438326099958));
#24718=CARTESIAN_POINT('Ctrl Pts',(1.61449324337233,-1.,-0.956354422921573));
#24719=CARTESIAN_POINT('Ctrl Pts',(1.60706069897794,-1.,-0.951613284361248));
#24720=CARTESIAN_POINT('Ctrl Pts',(1.59810042045408,-1.,-0.946078063325796));
#24721=CARTESIAN_POINT('Ctrl Pts',(1.58744937489796,-1.,-0.939646377909319));
#24722=CARTESIAN_POINT('Ctrl Pts',(1.57499388385561,-1.,-0.932246680128849));
#24723=CARTESIAN_POINT('Ctrl Pts',(1.56065988582509,-1.,-0.923832188966322));
#24724=CARTESIAN_POINT('Ctrl Pts',(1.54440491152807,-1.,-0.91437591904658));
#24725=CARTESIAN_POINT('Ctrl Pts',(1.52984849890434,-1.,-0.905967409640499));
#24726=CARTESIAN_POINT('Ctrl Pts',(1.51805569591479,-1.,-0.89918504749193));
#24727=CARTESIAN_POINT('Ctrl Pts',(1.50980486807181,-1.,-0.894452006967538));
#24728=CARTESIAN_POINT('Ctrl Pts',(1.5055822144029,-1.,-0.892032620296855));
#24729=CARTESIAN_POINT('',(1.60662857109684,-1.,-0.693717979106306));
#24730=CARTESIAN_POINT('Origin',(0.,-1.,0.));
#24731=CARTESIAN_POINT('',(2.0698113262342,-1.,-0.745574324794401));
#24732=CARTESIAN_POINT('Ctrl Pts',(1.60662857109684,-1.,-0.693717979106306));
#24733=CARTESIAN_POINT('Ctrl Pts',(1.61106790957619,-1.,-0.69571209787897));
#24734=CARTESIAN_POINT('Ctrl Pts',(1.61974673471117,-1.,-0.699605146398837));
#24735=CARTESIAN_POINT('Ctrl Pts',(1.6321654166204,-1.,-0.705159151977294));
#24736=CARTESIAN_POINT('Ctrl Pts',(1.64752408828442,-1.,-0.711993139340448));
#24737=CARTESIAN_POINT('Ctrl Pts',(1.66472880551777,-1.,-0.71958543378795));
#24738=CARTESIAN_POINT('Ctrl Pts',(1.67996158451922,-1.,-0.726235967982445));
#24739=CARTESIAN_POINT('Ctrl Pts',(1.69326921972915,-1.,-0.731963238685357));
#24740=CARTESIAN_POINT('Ctrl Pts',(1.70473309004249,-1.,-0.736799665716932));
#24741=CARTESIAN_POINT('Ctrl Pts',(1.71447789751001,-1.,-0.74079516202821));
#24742=CARTESIAN_POINT('Ctrl Pts',(1.72268229916769,-1.,-0.744021445433094));
#24743=CARTESIAN_POINT('Ctrl Pts',(1.72958533647714,-1.,-0.746574710097752));
#24744=CARTESIAN_POINT('Ctrl Pts',(1.7355035168033,-1.,-0.74858246295687));
#24745=CARTESIAN_POINT('Ctrl Pts',(1.74080458267114,-1.,-0.75019343598125));
#24746=CARTESIAN_POINT('Ctrl Pts',(1.74585086852502,-1.,-0.751555614164483));
#24747=CARTESIAN_POINT('Ctrl Pts',(1.75095139468794,-1.,-0.752797683531314));
#24748=CARTESIAN_POINT('Ctrl Pts',(1.75631083600019,-1.,-0.754009254027829));
#24749=CARTESIAN_POINT('Ctrl Pts',(1.76197817240128,-1.,-0.755220979974462));
#24750=CARTESIAN_POINT('Ctrl Pts',(1.76789396002998,-1.,-0.75642189602781));
#24751=CARTESIAN_POINT('Ctrl Pts',(1.77394167108292,-1.,-0.757578264077029));
#24752=CARTESIAN_POINT('Ctrl Pts',(1.77999411220945,-1.,-0.758650626677519));
#24753=CARTESIAN_POINT('Ctrl Pts',(1.78596964884604,-1.,-0.75961440111019));
#24754=CARTESIAN_POINT('Ctrl Pts',(1.7918581561088,-1.,-0.760469555880749));
#24755=CARTESIAN_POINT('Ctrl Pts',(1.79768986997783,-1.,-0.761229695230558));
#24756=CARTESIAN_POINT('Ctrl Pts',(1.80351583877342,-1.,-0.761915336443547));
#24757=CARTESIAN_POINT('Ctrl Pts',(1.80938551463965,-1.,-0.762546129463938));
#24758=CARTESIAN_POINT('Ctrl Pts',(1.8153211840553,-1.,-0.763132003836634));
#24759=CARTESIAN_POINT('Ctrl Pts',(1.82131873145266,-1.,-0.763673465462727));
#24760=CARTESIAN_POINT('Ctrl Pts',(1.82735991200065,-1.,-0.764165902605995));
#24761=CARTESIAN_POINT('Ctrl Pts',(1.83342077227142,-1.,-0.764602549687853));
#24762=CARTESIAN_POINT('Ctrl Pts',(1.83948181064835,-1.,-0.764978057881738));
#24763=CARTESIAN_POINT('Ctrl Pts',(1.84553698875924,-1.,-0.765291664862029));
#24764=CARTESIAN_POINT('Ctrl Pts',(1.85158945130063,-1.,-0.765545710619063));
#24765=CARTESIAN_POINT('Ctrl Pts',(1.85764741390394,-1.,-0.765744212909319));
#24766=CARTESIAN_POINT('Ctrl Pts',(1.86372027063312,-1.,-0.765891519092547));
#24767=CARTESIAN_POINT('Ctrl Pts',(1.86981398314341,-1.,-0.765990708546091));
#24768=CARTESIAN_POINT('Ctrl Pts',(1.87592888967883,-1.,-0.766042837036744));
#24769=CARTESIAN_POINT('Ctrl Pts',(1.88206215302561,-1.,-0.766047794851865));
#24770=CARTESIAN_POINT('Ctrl Pts',(1.88820926433409,-1.,-0.766004837062091));
#24771=CARTESIAN_POINT('Ctrl Pts',(1.89436577771388,-1.,-0.765913193856978));
#24772=CARTESIAN_POINT('Ctrl Pts',(1.90052930393596,-1.,-0.765772772593386));
#24773=CARTESIAN_POINT('Ctrl Pts',(1.90669961402356,-1.,-0.765584196937919));
#24774=CARTESIAN_POINT('Ctrl Pts',(1.91287765805169,-1.,-0.765348465884722));
#24775=CARTESIAN_POINT('Ctrl Pts',(1.91906491634196,-1.,-0.765066729667089));
#24776=CARTESIAN_POINT('Ctrl Pts',(1.92526263537048,-1.,-0.764740025488212));
#24777=CARTESIAN_POINT('Ctrl Pts',(1.93147105496382,-1.,-0.764369010673941));
#24778=CARTESIAN_POINT('Ctrl Pts',(1.93768964875886,-1.,-0.763954049121459));
#24779=CARTESIAN_POINT('Ctrl Pts',(1.9439174661764,-1.,-0.763495333538629));
#24780=CARTESIAN_POINT('Ctrl Pts',(1.95015342590024,-1.,-0.762992990878769));
#24781=CARTESIAN_POINT('Ctrl Pts',(1.95639665309869,-1.,-0.762447203806179));
#24782=CARTESIAN_POINT('Ctrl Pts',(1.96264672744186,-1.,-0.761858300014424));
#24783=CARTESIAN_POINT('Ctrl Pts',(1.96890351582499,-1.,-0.761226690483821));
#24784=CARTESIAN_POINT('Ctrl Pts',(1.97516705321494,-1.,-0.760552825409757));
#24785=CARTESIAN_POINT('Ctrl Pts',(1.98143741418172,-1.,-0.75983714745219));
#24786=CARTESIAN_POINT('Ctrl Pts',(1.98771456680874,-1.,-0.759080037802488));
#24787=CARTESIAN_POINT('Ctrl Pts',(1.99399831098817,-1.,-0.758281796766761));
#24788=CARTESIAN_POINT('Ctrl Pts',(2.00028834739178,-1.,-0.757442676862724));
#24789=CARTESIAN_POINT('Ctrl Pts',(2.0065843158773,-1.,-0.756562904646671));
#24790=CARTESIAN_POINT('Ctrl Pts',(2.01288584328084,-1.,-0.755642704957865));
#24791=CARTESIAN_POINT('Ctrl Pts',(2.01919259405809,-1.,-0.754682330722816));
#24792=CARTESIAN_POINT('Ctrl Pts',(2.02550428623313,-1.,-0.753682061112768));
#24793=CARTESIAN_POINT('Ctrl Pts',(2.03182068456221,-1.,-0.752642180487211));
#24794=CARTESIAN_POINT('Ctrl Pts',(2.03814160092099,-1.,-0.751562963361115));
#24795=CARTESIAN_POINT('Ctrl Pts',(2.04446689147979,-1.,-0.750444657875576));
#24796=CARTESIAN_POINT('Ctrl Pts',(2.05079645592154,-1.,-0.749287468665046));
#24797=CARTESIAN_POINT('Ctrl Pts',(2.05713023031006,-1.,-0.748091554183803));
#24798=CARTESIAN_POINT('Ctrl Pts',(2.06220058927826,-1.,-0.74710393278792));
#24799=CARTESIAN_POINT('Ctrl Pts',(2.06600523016815,-1.,-0.746345871544201));
#24800=CARTESIAN_POINT('Ctrl Pts',(2.06854248895728,-1.,-0.745832791378367));
#24801=CARTESIAN_POINT('Ctrl Pts',(2.0698113262342,-1.,-0.745574324794401));
#24802=CARTESIAN_POINT('',(2.11275013067528,-1.,-0.61342227326009));
#24803=CARTESIAN_POINT('',(2.0698113262342,-1.,-0.745574324794401));
#24804=CARTESIAN_POINT('',(1.7075470150345,-1.,-0.383122945602004));
#24805=CARTESIAN_POINT('Ctrl Pts',(2.11275013067528,-1.,-0.61342227326009));
#24806=CARTESIAN_POINT('Ctrl Pts',(2.11187554259986,-1.,-0.6124673655618));
#24807=CARTESIAN_POINT('Ctrl Pts',(2.11012443807238,-1.,-0.610560911689899));
#24808=CARTESIAN_POINT('Ctrl Pts',(2.1074919961518,-1.,-0.607711315454876));
#24809=CARTESIAN_POINT('Ctrl Pts',(2.10397049886949,-1.,-0.60393203073603));
#24810=CARTESIAN_POINT('Ctrl Pts',(2.0995493086477,-1.,-0.599241616420534));
#24811=CARTESIAN_POINT('Ctrl Pts',(2.0951087622027,-1.,-0.594585006052162));
#24812=CARTESIAN_POINT('Ctrl Pts',(2.09064881812129,-1.,-0.589962365403406));
#24813=CARTESIAN_POINT('Ctrl Pts',(2.08616943727951,-1.,-0.585373918991617));
#24814=CARTESIAN_POINT('Ctrl Pts',(2.08167059018418,-1.,-0.580819952108064));
#24815=CARTESIAN_POINT('Ctrl Pts',(2.07715226767559,-1.,-0.576300797416845));
#24816=CARTESIAN_POINT('Ctrl Pts',(2.07261449292824,-1.,-0.571816823242603));
#24817=CARTESIAN_POINT('Ctrl Pts',(2.06805732997334,-1.,-0.567368421181087));
#24818=CARTESIAN_POINT('Ctrl Pts',(2.06348090160589,-1.,-0.562955993082262));
#24819=CARTESIAN_POINT('Ctrl Pts',(2.05888537756462,-1.,-0.558579940185152));
#24820=CARTESIAN_POINT('Ctrl Pts',(2.05427091604413,-1.,-0.554240657463906));
#24821=CARTESIAN_POINT('Ctrl Pts',(2.04963761077958,-1.,-0.549938525150295));
#24822=CARTESIAN_POINT('Ctrl Pts',(2.04498544714588,-1.,-0.54567390381743));
#24823=CARTESIAN_POINT('Ctrl Pts',(2.04031422690527,-1.,-0.541447120615659));
#24824=CARTESIAN_POINT('Ctrl Pts',(2.03562362954037,-1.,-0.537258489833262));
#24825=CARTESIAN_POINT('Ctrl Pts',(2.03091336214426,-1.,-0.533108355132977));
#24826=CARTESIAN_POINT('Ctrl Pts',(2.0261832908329,-1.,-0.528997127241914));
#24827=CARTESIAN_POINT('Ctrl Pts',(2.02143356304698,-1.,-0.524925318333476));
#24828=CARTESIAN_POINT('Ctrl Pts',(2.01666477917286,-1.,-0.520893590399371));
#24829=CARTESIAN_POINT('Ctrl Pts',(2.01187773939242,-1.,-0.516902681728687));
#24830=CARTESIAN_POINT('Ctrl Pts',(2.00707309946949,-1.,-0.512953306961793));
#24831=CARTESIAN_POINT('Ctrl Pts',(2.00225107134734,-1.,-0.509046069886157));
#24832=CARTESIAN_POINT('Ctrl Pts',(1.99741107463572,-1.,-0.505181361323026));
#24833=CARTESIAN_POINT('Ctrl Pts',(1.99255149126155,-1.,-0.501359287727146));
#24834=CARTESIAN_POINT('Ctrl Pts',(1.98767044752932,-1.,-0.497579909545574));
#24835=CARTESIAN_POINT('Ctrl Pts',(1.98276658761821,-1.,-0.493843476541495));
#24836=CARTESIAN_POINT('Ctrl Pts',(1.97783973019229,-1.,-0.490150627860953));
#24837=CARTESIAN_POINT('Ctrl Pts',(1.97289186263272,-1.,-0.486502692907659));
#24838=CARTESIAN_POINT('Ctrl Pts',(1.96792703422362,-1.,-0.482901662120691));
#24839=CARTESIAN_POINT('Ctrl Pts',(1.96294933055943,-1.,-0.479349583074855));
#24840=CARTESIAN_POINT('Ctrl Pts',(1.95796111148177,-1.,-0.475848034683176));
#24841=CARTESIAN_POINT('Ctrl Pts',(1.95296148278133,-1.,-0.472397672264072));
#24842=CARTESIAN_POINT('Ctrl Pts',(1.94794381136514,-1.,-0.468997482913135));
#24843=CARTESIAN_POINT('Ctrl Pts',(1.9428979419619,-1.,-0.46564546202603));
#24844=CARTESIAN_POINT('Ctrl Pts',(1.93781486640821,-1.,-0.462340031009057));
#24845=CARTESIAN_POINT('Ctrl Pts',(1.93269066517934,-1.,-0.459081234547926));
#24846=CARTESIAN_POINT('Ctrl Pts',(1.92753067150476,-1.,-0.455872005174371));
#24847=CARTESIAN_POINT('Ctrl Pts',(1.92235380648502,-1.,-0.452719478359433));
#24848=CARTESIAN_POINT('Ctrl Pts',(1.91718342555755,-1.,-0.449632260106662));
#24849=CARTESIAN_POINT('Ctrl Pts',(1.9120369998112,-1.,-0.446617343485711));
#24850=CARTESIAN_POINT('Ctrl Pts',(1.90691756144898,-1.,-0.443677556849151));
#24851=CARTESIAN_POINT('Ctrl Pts',(1.90180124389086,-1.,-0.440807833704038));
#24852=CARTESIAN_POINT('Ctrl Pts',(1.89663648956466,-1.,-0.437995003948244));
#24853=CARTESIAN_POINT('Ctrl Pts',(1.89136993975504,-1.,-0.435225660963383));
#24854=CARTESIAN_POINT('Ctrl Pts',(1.88596913666793,-1.,-0.432493038548748));
#24855=CARTESIAN_POINT('Ctrl Pts',(1.88044229001832,-1.,-0.429803062482345));
#24856=CARTESIAN_POINT('Ctrl Pts',(1.87486989291484,-1.,-0.427183828519102));
#24857=CARTESIAN_POINT('Ctrl Pts',(1.86937803944323,-1.,-0.424678177291359));
#24858=CARTESIAN_POINT('Ctrl Pts',(1.86408083334028,-1.,-0.422327307418275));
#24859=CARTESIAN_POINT('Ctrl Pts',(1.85903281096686,-1.,-0.42015728797562));
#24860=CARTESIAN_POINT('Ctrl Pts',(1.85417632856234,-1.,-0.418164129143534));
#24861=CARTESIAN_POINT('Ctrl Pts',(1.84929312929882,-1.,-0.416300022038864));
#24862=CARTESIAN_POINT('Ctrl Pts',(1.8440575707371,-1.,-0.41448743825434));
#24863=CARTESIAN_POINT('Ctrl Pts',(1.83808953475839,-1.,-0.412633125322162));
#24864=CARTESIAN_POINT('Ctrl Pts',(1.83100408895216,-1.,-0.410641256301675));
#24865=CARTESIAN_POINT('Ctrl Pts',(1.8224702267854,-1.,-0.408428948108534));
#24866=CARTESIAN_POINT('Ctrl Pts',(1.81223801813988,-1.,-0.405933518411838));
#24867=CARTESIAN_POINT('Ctrl Pts',(1.80012077176221,-1.,-0.403107976170441));
#24868=CARTESIAN_POINT('Ctrl Pts',(1.78598826347533,-1.,-0.399919403783081));
#24869=CARTESIAN_POINT('Ctrl Pts',(1.7697556004756,-1.,-0.39634619612042));
#24870=CARTESIAN_POINT('Ctrl Pts',(1.75137405313962,-1.,-0.392375812294307));
#24871=CARTESIAN_POINT('Ctrl Pts',(1.7349317097561,-1.,-0.388877023509192));
#24872=CARTESIAN_POINT('Ctrl Pts',(1.72162022246158,-1.,-0.38607079032701));
#24873=CARTESIAN_POINT('Ctrl Pts',(1.71231062891958,-1.,-0.384119047315542));
#24874=CARTESIAN_POINT('Ctrl Pts',(1.7075470150345,-1.,-0.383122945602004));
#24875=CARTESIAN_POINT('',(1.74236521665491,-1.,-0.163289472382896));
#24876=CARTESIAN_POINT('Origin',(0.,-1.,0.));
#24877=CARTESIAN_POINT('',(2.19890268624765,-1.,-0.0694764450219582));
#24878=CARTESIAN_POINT('Ctrl Pts',(1.74236521665491,-1.,-0.163289472382896));
#24879=CARTESIAN_POINT('Ctrl Pts',(1.7472034950333,-1.,-0.163814161002002));
#24880=CARTESIAN_POINT('Ctrl Pts',(1.75666056638427,-1.,-0.164834765707159));
#24881=CARTESIAN_POINT('Ctrl Pts',(1.77018771684844,-1.,-0.1662793551464));
#24882=CARTESIAN_POINT('Ctrl Pts',(1.7869064998507,-1.,-0.168032772805197));
#24883=CARTESIAN_POINT('Ctrl Pts',(1.80561530629706,-1.,-0.169936923904608));
#24884=CARTESIAN_POINT('Ctrl Pts',(1.82215766811545,-1.,-0.171554770204119));
#24885=CARTESIAN_POINT('Ctrl Pts',(1.83658380527692,-1.,-0.1728894428919));
#24886=CARTESIAN_POINT('Ctrl Pts',(1.8489811319852,-1.,-0.173946627587732));
#24887=CARTESIAN_POINT('Ctrl Pts',(1.85948367088837,-1.,-0.17473525927603));
#24888=CARTESIAN_POINT('Ctrl Pts',(1.86828349694799,-1.,-0.175268337590758));
#24889=CARTESIAN_POINT('Ctrl Pts',(1.87563767773588,-1.,-0.175563480746485));
#24890=CARTESIAN_POINT('Ctrl Pts',(1.88188663145367,-1.,-0.175644148889699));
#24891=CARTESIAN_POINT('Ctrl Pts',(1.88742606273259,-1.,-0.175538155840648));
#24892=CARTESIAN_POINT('Ctrl Pts',(1.892646301985,-1.,-0.175274276190844));
#24893=CARTESIAN_POINT('Ctrl Pts',(1.89788101117132,-1.,-0.174879405091263));
#24894=CARTESIAN_POINT('Ctrl Pts',(1.90335253862834,-1.,-0.174375518661085));
#24895=CARTESIAN_POINT('Ctrl Pts',(1.90911693975267,-1.,-0.173776635257817));
#24896=CARTESIAN_POINT('Ctrl Pts',(1.91511429159527,-1.,-0.173090695383496));
#24897=CARTESIAN_POINT('Ctrl Pts',(1.9212233439798,-1.,-0.172321621259514));
#24898=CARTESIAN_POINT('Ctrl Pts',(1.92731093582036,-1.,-0.171471191532988));
#24899=CARTESIAN_POINT('Ctrl Pts',(1.93329183155539,-1.,-0.170541253116202));
#24900=CARTESIAN_POINT('Ctrl Pts',(1.93915639211581,-1.,-0.169534904817491));
#24901=CARTESIAN_POINT('Ctrl Pts',(1.94493757756931,-1.,-0.168455741607556));
#24902=CARTESIAN_POINT('Ctrl Pts',(1.95069027794294,-1.,-0.167307501784476));
#24903=CARTESIAN_POINT('Ctrl Pts',(1.9564675971873,-1.,-0.166093592002813));
#24904=CARTESIAN_POINT('Ctrl Pts',(1.96229379940136,-1.,-0.164816568920269));
#24905=CARTESIAN_POINT('Ctrl Pts',(1.96816512677967,-1.,-0.163478185457734));
#24906=CARTESIAN_POINT('Ctrl Pts',(1.97406280235188,-1.,-0.162079693556289));
#24907=CARTESIAN_POINT('Ctrl Pts',(1.97996195437559,-1.,-0.160622060784611));
#24908=CARTESIAN_POINT('Ctrl Pts',(1.98584238283292,-1.,-0.159106226437299));
#24909=CARTESIAN_POINT('Ctrl Pts',(1.99169810931908,-1.,-0.157533331459227));
#24910=CARTESIAN_POINT('Ctrl Pts',(1.99753284771497,-1.,-0.155904629548784));
#24911=CARTESIAN_POINT('Ctrl Pts',(2.00335565310543,-1.,-0.154221403049722));
#24912=CARTESIAN_POINT('Ctrl Pts',(2.00917680318424,-1.,-0.15248488362145));
#24913=CARTESIAN_POINT('Ctrl Pts',(2.01500291940238,-1.,-0.150696157673078));
#24914=CARTESIAN_POINT('Ctrl Pts',(2.02083464969894,-1.,-0.148856124775337));
#24915=CARTESIAN_POINT('Ctrl Pts',(2.02666926182017,-1.,-0.146965557332583));
#24916=CARTESIAN_POINT('Ctrl Pts',(2.03250223739942,-1.,-0.145025140186058));
#24917=CARTESIAN_POINT('Ctrl Pts',(2.03832911025912,-1.,-0.143035515058209));
#24918=CARTESIAN_POINT('Ctrl Pts',(2.04414757947916,-1.,-0.140997332152546));
#24919=CARTESIAN_POINT('Ctrl Pts',(2.04995762001328,-1.,-0.138911255368966));
#24920=CARTESIAN_POINT('Ctrl Pts',(2.05576044414264,-1.,-0.136777941218044));
#24921=CARTESIAN_POINT('Ctrl Pts',(2.06155781517842,-1.,-0.134598026192106));
#24922=CARTESIAN_POINT('Ctrl Pts',(2.06735123910326,-1.,-0.132372111547711));
#24923=CARTESIAN_POINT('Ctrl Pts',(2.07314114713063,-1.,-0.130100748328404));
#24924=CARTESIAN_POINT('Ctrl Pts',(2.07892715110987,-1.,-0.12778444527612));
#24925=CARTESIAN_POINT('Ctrl Pts',(2.08470840653643,-1.,-0.125423679412062));
#24926=CARTESIAN_POINT('Ctrl Pts',(2.09048392424825,-1.,-0.123018905621083));
#24927=CARTESIAN_POINT('Ctrl Pts',(2.0962529286773,-1.,-0.120570567965122));
#24928=CARTESIAN_POINT('Ctrl Pts',(2.102015121329,-1.,-0.118079107988356));
#24929=CARTESIAN_POINT('Ctrl Pts',(2.10777050261309,-1.,-0.115544957687927));
#24930=CARTESIAN_POINT('Ctrl Pts',(2.11351924490306,-1.,-0.112968534419737));
#24931=CARTESIAN_POINT('Ctrl Pts',(2.11926155590865,-1.,-0.110350236135025));
#24932=CARTESIAN_POINT('Ctrl Pts',(2.12499752307,-1.,-0.10769043523109));
#24933=CARTESIAN_POINT('Ctrl Pts',(2.13072704887293,-1.,-0.10498947915274));
#24934=CARTESIAN_POINT('Ctrl Pts',(2.13644992667165,-1.,-0.102247700556101));
#24935=CARTESIAN_POINT('Ctrl Pts',(2.14216588396025,-1.,-0.0994654261990917));
#24936=CARTESIAN_POINT('Ctrl Pts',(2.14787463531795,-1.,-0.096642985230546));
#24937=CARTESIAN_POINT('Ctrl Pts',(2.1535759397817,-1.,-0.0937807218867645));
#24938=CARTESIAN_POINT('Ctrl Pts',(2.15926961544516,-1.,-0.0908789888107267));
#24939=CARTESIAN_POINT('Ctrl Pts',(2.16495552645014,-1.,-0.0879381291386924));
#24940=CARTESIAN_POINT('Ctrl Pts',(2.17063357870952,-1.,-0.0849584620835374));
#24941=CARTESIAN_POINT('Ctrl Pts',(2.176303712113,-1.,-0.0819402680872767));
#24942=CARTESIAN_POINT('Ctrl Pts',(2.18196589448887,-1.,-0.0788837727685244));
#24943=CARTESIAN_POINT('Ctrl Pts',(2.1876201139953,-1.,-0.0757891465836149));
#24944=CARTESIAN_POINT('Ctrl Pts',(2.19213712013662,-1.,-0.0732830357306726));
#24945=CARTESIAN_POINT('Ctrl Pts',(2.19552129484002,-1.,-0.0713863779526155));
#24946=CARTESIAN_POINT('Ctrl Pts',(2.19777582085423,-1.,-0.0701143536325491));
#24947=CARTESIAN_POINT('Ctrl Pts',(2.19890268624765,-1.,-0.0694764450219582));
#24948=CARTESIAN_POINT('',(2.19890268624765,-1.,0.0694764450219582));
#24949=CARTESIAN_POINT('',(2.19890268624765,-1.,-0.0694764450219582));
#24950=CARTESIAN_POINT('',(1.74236521665491,-1.,0.163289472382896));
#24951=CARTESIAN_POINT('Ctrl Pts',(2.19890268624765,-1.,0.0694764450219582));
#24952=CARTESIAN_POINT('Ctrl Pts',(2.19777582085261,-1.,0.0701143536324925));
#24953=CARTESIAN_POINT('Ctrl Pts',(2.19552129483562,-1.,0.0713863779524626));
#24954=CARTESIAN_POINT('Ctrl Pts',(2.19213712012956,-1.,0.0732830357304275));
#24955=CARTESIAN_POINT('Ctrl Pts',(2.1876201139874,-1.,0.075789146583341));
#24956=CARTESIAN_POINT('Ctrl Pts',(2.18196589448304,-1.,0.0788837727683226));
#24957=CARTESIAN_POINT('Ctrl Pts',(2.1763037121106,-1.,0.0819402680871938));
#24958=CARTESIAN_POINT('Ctrl Pts',(2.17063357871031,-1.,0.0849584620835642));
#24959=CARTESIAN_POINT('Ctrl Pts',(2.16495552645275,-1.,0.0879381291387821));
#24960=CARTESIAN_POINT('Ctrl Pts',(2.15926961544808,-1.,0.0908789888108265));
#24961=CARTESIAN_POINT('Ctrl Pts',(2.15357593978377,-1.,0.0937807218868344));
#24962=CARTESIAN_POINT('Ctrl Pts',(2.14787463531864,-1.,0.0966429852305688));
#24963=CARTESIAN_POINT('Ctrl Pts',(2.14216588395974,-1.,0.0994654261990741));
#24964=CARTESIAN_POINT('Ctrl Pts',(2.13644992667052,-1.,0.102247700556063));
#24965=CARTESIAN_POINT('Ctrl Pts',(2.1307270488718,-1.,0.104989479152703));
#24966=CARTESIAN_POINT('Ctrl Pts',(2.12499752306927,-1.,0.107690435231068));
#24967=CARTESIAN_POINT('Ctrl Pts',(2.11926155590849,-1.,0.11035023613502));
#24968=CARTESIAN_POINT('Ctrl Pts',(2.11351924490335,-1.,0.112968534419746));
#24969=CARTESIAN_POINT('Ctrl Pts',(2.10777050261359,-1.,0.11554495768794));
#24970=CARTESIAN_POINT('Ctrl Pts',(2.10201512132945,-1.,0.118079107988368));
#24971=CARTESIAN_POINT('Ctrl Pts',(2.09625292867756,-1.,0.120570567965129));
#24972=CARTESIAN_POINT('Ctrl Pts',(2.09048392424826,-1.,0.123018905621083));
#24973=CARTESIAN_POINT('Ctrl Pts',(2.08470840653628,-1.,0.125423679412058));
#24974=CARTESIAN_POINT('Ctrl Pts',(2.07892715110967,-1.,0.127784445276116));
#24975=CARTESIAN_POINT('Ctrl Pts',(2.07314114713047,-1.,0.1301007483284));
#24976=CARTESIAN_POINT('Ctrl Pts',(2.06735123910319,-1.,0.132372111547709));
#24977=CARTESIAN_POINT('Ctrl Pts',(2.06155781517844,-1.,0.134598026192107));
#24978=CARTESIAN_POINT('Ctrl Pts',(2.0557604441427,-1.,0.136777941218044));
#24979=CARTESIAN_POINT('Ctrl Pts',(2.04995762001333,-1.,0.138911255368966));
#24980=CARTESIAN_POINT('Ctrl Pts',(2.04414757947919,-1.,0.140997332152545));
#24981=CARTESIAN_POINT('Ctrl Pts',(2.03832911025913,-1.,0.143035515058208));
#24982=CARTESIAN_POINT('Ctrl Pts',(2.03250223739941,-1.,0.145025140186058));
#24983=CARTESIAN_POINT('Ctrl Pts',(2.02666926182017,-1.,0.146965557332586));
#24984=CARTESIAN_POINT('Ctrl Pts',(2.02083464969897,-1.,0.148856124775342));
#24985=CARTESIAN_POINT('Ctrl Pts',(2.01500291940243,-1.,0.150696157673084));
#24986=CARTESIAN_POINT('Ctrl Pts',(2.00917680318426,-1.,0.152484883621452));
#24987=CARTESIAN_POINT('Ctrl Pts',(2.00335565310539,-1.,0.154221403049719));
#24988=CARTESIAN_POINT('Ctrl Pts',(1.99753284771487,-1.,0.155904629548774));
#24989=CARTESIAN_POINT('Ctrl Pts',(1.99169810931893,-1.,0.157533331459215));
#24990=CARTESIAN_POINT('Ctrl Pts',(1.98584238283279,-1.,0.159106226437288));
#24991=CARTESIAN_POINT('Ctrl Pts',(1.97996195437557,-1.,0.16062206078461));
#24992=CARTESIAN_POINT('Ctrl Pts',(1.97406280235204,-1.,0.162079693556302));
#24993=CARTESIAN_POINT('Ctrl Pts',(1.96816512678,-1.,0.16347818545776));
#24994=CARTESIAN_POINT('Ctrl Pts',(1.96229379940174,-1.,0.1648165689203));
#24995=CARTESIAN_POINT('Ctrl Pts',(1.95646759718755,-1.,0.166093592002832));
#24996=CARTESIAN_POINT('Ctrl Pts',(1.95069027794286,-1.,0.167307501784469));
#24997=CARTESIAN_POINT('Ctrl Pts',(1.94493757756879,-1.,0.168455741607515));
#24998=CARTESIAN_POINT('Ctrl Pts',(1.93915639211497,-1.,0.169534904817425));
#24999=CARTESIAN_POINT('Ctrl Pts',(1.93329183155455,-1.,0.170541253116136));
#25000=CARTESIAN_POINT('Ctrl Pts',(1.92731093582,-1.,0.17147119153296));
#25001=CARTESIAN_POINT('Ctrl Pts',(1.92122334398034,-1.,0.172321621259556));
#25002=CARTESIAN_POINT('Ctrl Pts',(1.91511429159681,-1.,0.173090695383619));
#25003=CARTESIAN_POINT('Ctrl Pts',(1.90911693975475,-1.,0.173776635257983));
#25004=CARTESIAN_POINT('Ctrl Pts',(1.90335253863003,-1.,0.174375518661222));
#25005=CARTESIAN_POINT('Ctrl Pts',(1.89788101117148,-1.,0.174879405091277));
#25006=CARTESIAN_POINT('Ctrl Pts',(1.89264630198279,-1.,0.175274276190664));
#25007=CARTESIAN_POINT('Ctrl Pts',(1.88742606272818,-1.,0.175538155840286));
#25008=CARTESIAN_POINT('Ctrl Pts',(1.88188663144846,-1.,0.175644148889271));
#25009=CARTESIAN_POINT('Ctrl Pts',(1.87563767773249,-1.,0.175563480746205));
#25010=CARTESIAN_POINT('Ctrl Pts',(1.86828349694972,-1.,0.1752683375909));
#25011=CARTESIAN_POINT('Ctrl Pts',(1.85948367089838,-1.,0.174735259276856));
#25012=CARTESIAN_POINT('Ctrl Pts',(1.84898113200543,-1.,0.173946627589401));
#25013=CARTESIAN_POINT('Ctrl Pts',(1.83658380530747,-1.,0.17288944289442));
#25014=CARTESIAN_POINT('Ctrl Pts',(1.82215766815414,-1.,0.171554770207306));
#25015=CARTESIAN_POINT('Ctrl Pts',(1.80561530633924,-1.,0.169936923908078));
#25016=CARTESIAN_POINT('Ctrl Pts',(1.78690649988931,-1.,0.16803277280837));
#25017=CARTESIAN_POINT('Ctrl Pts',(1.77018771687692,-1.,0.166279355148738));
#25018=CARTESIAN_POINT('Ctrl Pts',(1.75666056640041,-1.,0.164834765708484));
#25019=CARTESIAN_POINT('Ctrl Pts',(1.74720349503904,-1.,0.163814161002474));
#25020=CARTESIAN_POINT('Ctrl Pts',(1.74236521665491,-1.,0.163289472382896));
#25021=CARTESIAN_POINT('',(1.7075470150345,-1.,0.383122945602004));
#25022=CARTESIAN_POINT('Origin',(0.,-1.,0.));
#25023=CARTESIAN_POINT('',(2.11275013067528,-1.,0.613422273260091));
#25024=CARTESIAN_POINT('Ctrl Pts',(1.7075470150345,-1.,0.383122945602004));
#25025=CARTESIAN_POINT('Ctrl Pts',(1.71231062891398,-1.,0.384119047314215));
#25026=CARTESIAN_POINT('Ctrl Pts',(1.72162022244582,-1.,0.386070790323281));
#25027=CARTESIAN_POINT('Ctrl Pts',(1.73493170972829,-1.,0.388877023502615));
#25028=CARTESIAN_POINT('Ctrl Pts',(1.75137405310193,-1.,0.392375812285396));
#25029=CARTESIAN_POINT('Ctrl Pts',(1.76975560043442,-1.,0.396346196110688));
#25030=CARTESIAN_POINT('Ctrl Pts',(1.78598826343754,-1.,0.399919403774156));
#25031=CARTESIAN_POINT('Ctrl Pts',(1.80012077173238,-1.,0.403107976163396));
#25032=CARTESIAN_POINT('Ctrl Pts',(1.81223801812013,-1.,0.405933518407176));
#25033=CARTESIAN_POINT('Ctrl Pts',(1.82247022677562,-1.,0.408428948106228));
#25034=CARTESIAN_POINT('Ctrl Pts',(1.83100408895047,-1.,0.410641256301276));
#25035=CARTESIAN_POINT('Ctrl Pts',(1.8380895347617,-1.,0.412633125322945));
#25036=CARTESIAN_POINT('Ctrl Pts',(1.84405757074218,-1.,0.414487438255542));
#25037=CARTESIAN_POINT('Ctrl Pts',(1.84929312930314,-1.,0.416300022039885));
#25038=CARTESIAN_POINT('Ctrl Pts',(1.8541763285645,-1.,0.418164129144046));
#25039=CARTESIAN_POINT('Ctrl Pts',(1.8590328109667,-1.,0.420157287975583));
#25040=CARTESIAN_POINT('Ctrl Pts',(1.86408083333863,-1.,0.422327307417885));
#25041=CARTESIAN_POINT('Ctrl Pts',(1.8693780394412,-1.,0.424678177290876));
#25042=CARTESIAN_POINT('Ctrl Pts',(1.87486989291333,-1.,0.427183828518743));
#25043=CARTESIAN_POINT('Ctrl Pts',(1.88044229001778,-1.,0.429803062482217));
#25044=CARTESIAN_POINT('Ctrl Pts',(1.88596913666828,-1.,0.432493038548833));
#25045=CARTESIAN_POINT('Ctrl Pts',(1.89136993975585,-1.,0.43522566096358));
#25046=CARTESIAN_POINT('Ctrl Pts',(1.89663648956549,-1.,0.437995003948443));
#25047=CARTESIAN_POINT('Ctrl Pts',(1.90180124389137,-1.,0.440807833704161));
#25048=CARTESIAN_POINT('Ctrl Pts',(1.90691756144906,-1.,0.443677556849171));
#25049=CARTESIAN_POINT('Ctrl Pts',(1.91203699981095,-1.,0.446617343485651));
#25050=CARTESIAN_POINT('Ctrl Pts',(1.91718342555717,-1.,0.449632260106572));
#25051=CARTESIAN_POINT('Ctrl Pts',(1.9223538064847,-1.,0.452719478359356));
#25052=CARTESIAN_POINT('Ctrl Pts',(1.92753067150461,-1.,0.455872005174336));
#25053=CARTESIAN_POINT('Ctrl Pts',(1.93269066517936,-1.,0.459081234547932));
#25054=CARTESIAN_POINT('Ctrl Pts',(1.93781486640834,-1.,0.462340031009087));
#25055=CARTESIAN_POINT('Ctrl Pts',(1.94289794196205,-1.,0.465645462026065));
#25056=CARTESIAN_POINT('Ctrl Pts',(1.94794381136524,-1.,0.468997482913158));
#25057=CARTESIAN_POINT('Ctrl Pts',(1.95296148278136,-1.,0.47239767226408));
#25058=CARTESIAN_POINT('Ctrl Pts',(1.95796111148175,-1.,0.475848034683172));
#25059=CARTESIAN_POINT('Ctrl Pts',(1.96294933055938,-1.,0.479349583074846));
#25060=CARTESIAN_POINT('Ctrl Pts',(1.96792703422358,-1.,0.482901662120687));
#25061=CARTESIAN_POINT('Ctrl Pts',(1.97289186263272,-1.,0.486502692907661));
#25062=CARTESIAN_POINT('Ctrl Pts',(1.97783973019229,-1.,0.490150627860955));
#25063=CARTESIAN_POINT('Ctrl Pts',(1.9827665876182,-1.,0.493843476541493));
#25064=CARTESIAN_POINT('Ctrl Pts',(1.98767044752929,-1.,0.497579909545564));
#25065=CARTESIAN_POINT('Ctrl Pts',(1.9925514912615,-1.,0.501359287727129));
#25066=CARTESIAN_POINT('Ctrl Pts',(1.99741107463567,-1.,0.505181361323011));
#25067=CARTESIAN_POINT('Ctrl Pts',(2.00225107134733,-1.,0.509046069886152));
#25068=CARTESIAN_POINT('Ctrl Pts',(2.00707309946955,-1.,0.512953306961814));
#25069=CARTESIAN_POINT('Ctrl Pts',(2.01187773939257,-1.,0.516902681728733));
#25070=CARTESIAN_POINT('Ctrl Pts',(2.01666477917305,-1.,0.520893590399429));
#25071=CARTESIAN_POINT('Ctrl Pts',(2.02143356304712,-1.,0.524925318333519));
#25072=CARTESIAN_POINT('Ctrl Pts',(2.02618329083289,-1.,0.528997127241911));
#25073=CARTESIAN_POINT('Ctrl Pts',(2.03091336214401,-1.,0.533108355132905));
#25074=CARTESIAN_POINT('Ctrl Pts',(2.03562362953993,-1.,0.537258489833135));
#25075=CARTESIAN_POINT('Ctrl Pts',(2.0403142269048,-1.,0.54144712061552));
#25076=CARTESIAN_POINT('Ctrl Pts',(2.0449854471456,-1.,0.545673903817349));
#25077=CARTESIAN_POINT('Ctrl Pts',(2.04963761077974,-1.,0.549938525150342));
#25078=CARTESIAN_POINT('Ctrl Pts',(2.05427091604482,-1.,0.55424065746411));
#25079=CARTESIAN_POINT('Ctrl Pts',(2.05888537756571,-1.,0.558579940185468));
#25080=CARTESIAN_POINT('Ctrl Pts',(2.06348090160697,-1.,0.562955993082574));
#25081=CARTESIAN_POINT('Ctrl Pts',(2.06805732997383,-1.,0.56736842118123));
#25082=CARTESIAN_POINT('Ctrl Pts',(2.07261449292757,-1.,0.571816823242411));
#25083=CARTESIAN_POINT('Ctrl Pts',(2.07715226767361,-1.,0.576300797416275));
#25084=CARTESIAN_POINT('Ctrl Pts',(2.08167059018138,-1.,0.580819952107257));
#25085=CARTESIAN_POINT('Ctrl Pts',(2.086169437277,-1.,0.585373918990895));
#25086=CARTESIAN_POINT('Ctrl Pts',(2.09064881812053,-1.,0.58996236540319));
#25087=CARTESIAN_POINT('Ctrl Pts',(2.09510876220501,-1.,0.594585006052824));
#25088=CARTESIAN_POINT('Ctrl Pts',(2.09954930865331,-1.,0.599241616422144));
#25089=CARTESIAN_POINT('Ctrl Pts',(2.10397049887709,-1.,0.603932030738212));
#25090=CARTESIAN_POINT('Ctrl Pts',(2.10749199615859,-1.,0.607711315456826));
#25091=CARTESIAN_POINT('Ctrl Pts',(2.11012443807661,-1.,0.610560911691114));
#25092=CARTESIAN_POINT('Ctrl Pts',(2.11187554260142,-1.,0.61246736556225));
#25093=CARTESIAN_POINT('Ctrl Pts',(2.11275013067528,-1.,0.613422273260091));
#25094=CARTESIAN_POINT('',(2.0698113262342,-1.,0.745574324794401));
#25095=CARTESIAN_POINT('',(2.11275013067528,-1.,0.613422273260091));
#25096=CARTESIAN_POINT('Ctrl Pts',(2.0698113262342,-1.,0.745574324794401));
#25097=CARTESIAN_POINT('Ctrl Pts',(2.06854248895575,-1.,0.74583279137781));
#25098=CARTESIAN_POINT('Ctrl Pts',(2.06600523016401,-1.,0.746345871542696));
#25099=CARTESIAN_POINT('Ctrl Pts',(2.06220058927162,-1.,0.747103932785504));
#25100=CARTESIAN_POINT('Ctrl Pts',(2.05713023030263,-1.,0.748091554181101));
#25101=CARTESIAN_POINT('Ctrl Pts',(2.05079645591606,-1.,0.749287468663053));
#25102=CARTESIAN_POINT('Ctrl Pts',(2.04446689147754,-1.,0.750444657874758));
#25103=CARTESIAN_POINT('Ctrl Pts',(2.03814160092173,-1.,0.751562963361384));
#25104=CARTESIAN_POINT('Ctrl Pts',(2.03182068456467,-1.,0.752642180488104));
#25105=CARTESIAN_POINT('Ctrl Pts',(2.02550428623587,-1.,0.753682061113766));
#25106=CARTESIAN_POINT('Ctrl Pts',(2.01919259406003,-1.,0.75468233072352));
#25107=CARTESIAN_POINT('Ctrl Pts',(2.01288584328149,-1.,0.755642704958101));
#25108=CARTESIAN_POINT('Ctrl Pts',(2.00658431587682,-1.,0.756562904646496));
#25109=CARTESIAN_POINT('Ctrl Pts',(2.00028834739072,-1.,0.757442676862342));
#25110=CARTESIAN_POINT('Ctrl Pts',(1.9939983109871,-1.,0.758281796766377));
#25111=CARTESIAN_POINT('Ctrl Pts',(1.98771456680806,-1.,0.759080037802243));
#25112=CARTESIAN_POINT('Ctrl Pts',(1.98143741418156,-1.,0.759837147452135));
#25113=CARTESIAN_POINT('Ctrl Pts',(1.97516705321521,-1.,0.760552825409856));
#25114=CARTESIAN_POINT('Ctrl Pts',(1.96890351582545,-1.,0.761226690483986));
#25115=CARTESIAN_POINT('Ctrl Pts',(1.96264672744229,-1.,0.761858300014575));
#25116=CARTESIAN_POINT('Ctrl Pts',(1.95639665309893,-1.,0.762447203806264));
#25117=CARTESIAN_POINT('Ctrl Pts',(1.95015342590025,-1.,0.762992990878774));
#25118=CARTESIAN_POINT('Ctrl Pts',(1.94391746617626,-1.,0.763495333538581));
#25119=CARTESIAN_POINT('Ctrl Pts',(1.93768964875867,-1.,0.763954049121394));
#25120=CARTESIAN_POINT('Ctrl Pts',(1.93147105496367,-1.,0.76436901067389));
#25121=CARTESIAN_POINT('Ctrl Pts',(1.92526263537041,-1.,0.764740025488189));
#25122=CARTESIAN_POINT('Ctrl Pts',(1.91906491634197,-1.,0.765066729667095));
#25123=CARTESIAN_POINT('Ctrl Pts',(1.91287765805174,-1.,0.765348465884739));
#25124=CARTESIAN_POINT('Ctrl Pts',(1.90669961402362,-1.,0.765584196937937));
#25125=CARTESIAN_POINT('Ctrl Pts',(1.90052930393599,-1.,0.765772772593395));
#25126=CARTESIAN_POINT('Ctrl Pts',(1.89436577771389,-1.,0.765913193856979));
#25127=CARTESIAN_POINT('Ctrl Pts',(1.88820926433409,-1.,0.76600483706209));
#25128=CARTESIAN_POINT('Ctrl Pts',(1.88206215302561,-1.,0.766047794851869));
#25129=CARTESIAN_POINT('Ctrl Pts',(1.87592888967886,-1.,0.766042837036759));
#25130=CARTESIAN_POINT('Ctrl Pts',(1.86981398314345,-1.,0.765990708546112));
#25131=CARTESIAN_POINT('Ctrl Pts',(1.86372027063314,-1.,0.765891519092557));
#25132=CARTESIAN_POINT('Ctrl Pts',(1.85764741390391,-1.,0.765744212909305));
#25133=CARTESIAN_POINT('Ctrl Pts',(1.85158945130054,-1.,0.765545710619023));
#25134=CARTESIAN_POINT('Ctrl Pts',(1.8455369887591,-1.,0.765291664861972));
#25135=CARTESIAN_POINT('Ctrl Pts',(1.83948181064823,-1.,0.764978057881688));
#25136=CARTESIAN_POINT('Ctrl Pts',(1.8334207722714,-1.,0.764602549687846));
#25137=CARTESIAN_POINT('Ctrl Pts',(1.8273599120008,-1.,0.764165902606056));
#25138=CARTESIAN_POINT('Ctrl Pts',(1.82131873145297,-1.,0.763673465462854));
#25139=CARTESIAN_POINT('Ctrl Pts',(1.81532118405566,-1.,0.763132003836783));
#25140=CARTESIAN_POINT('Ctrl Pts',(1.80938551463989,-1.,0.762546129464036));
#25141=CARTESIAN_POINT('Ctrl Pts',(1.80351583877334,-1.,0.761915336443516));
#25142=CARTESIAN_POINT('Ctrl Pts',(1.79768986997735,-1.,0.761229695230359));
#25143=CARTESIAN_POINT('Ctrl Pts',(1.79185815610802,-1.,0.760469555880425));
#25144=CARTESIAN_POINT('Ctrl Pts',(1.78596964884526,-1.,0.759614401109868));
#25145=CARTESIAN_POINT('Ctrl Pts',(1.77999411220912,-1.,0.75865062667738));
#25146=CARTESIAN_POINT('Ctrl Pts',(1.77394167108342,-1.,0.757578264077238));
#25147=CARTESIAN_POINT('Ctrl Pts',(1.76789396003141,-1.,0.756421896028403));
#25148=CARTESIAN_POINT('Ctrl Pts',(1.7619781724032,-1.,0.755220979975262));
#25149=CARTESIAN_POINT('Ctrl Pts',(1.75631083600175,-1.,0.75400925402848));
#25150=CARTESIAN_POINT('Ctrl Pts',(1.75095139468809,-1.,0.752797683531377));
#25151=CARTESIAN_POINT('Ctrl Pts',(1.74585086852298,-1.,0.751555614163629));
#25152=CARTESIAN_POINT('Ctrl Pts',(1.74080458266705,-1.,0.750193435979541));
#25153=CARTESIAN_POINT('Ctrl Pts',(1.73550351679848,-1.,0.748582462954855));
#25154=CARTESIAN_POINT('Ctrl Pts',(1.72958533647399,-1.,0.746574710096437));
#25155=CARTESIAN_POINT('Ctrl Pts',(1.7226822991693,-1.,0.744021445433765));
#25156=CARTESIAN_POINT('Ctrl Pts',(1.71447789751927,-1.,0.740795162032088));
#25157=CARTESIAN_POINT('Ctrl Pts',(1.70473309006121,-1.,0.736799665724771));
#25158=CARTESIAN_POINT('Ctrl Pts',(1.69326921975743,-1.,0.731963238697195));
#25159=CARTESIAN_POINT('Ctrl Pts',(1.67996158455503,-1.,0.726235967997433));
#25160=CARTESIAN_POINT('Ctrl Pts',(1.6647288055568,-1.,0.719585433804282));
#25161=CARTESIAN_POINT('Ctrl Pts',(1.64752408832016,-1.,0.711993139355394));
#25162=CARTESIAN_POINT('Ctrl Pts',(1.63216541664676,-1.,0.705159151988319));
#25163=CARTESIAN_POINT('Ctrl Pts',(1.61974673472612,-1.,0.699605146405088));
#25164=CARTESIAN_POINT('Ctrl Pts',(1.61106790958151,-1.,0.695712097881194));
#25165=CARTESIAN_POINT('Ctrl Pts',(1.60662857109684,-1.,0.693717979106306));
#25166=CARTESIAN_POINT('Origin',(0.,-1.,0.));
#25167=CARTESIAN_POINT('Origin',(0.,0.,0.));
#25168=CARTESIAN_POINT('Origin',(0.,2.2,0.));
#25169=CARTESIAN_POINT('Origin',(0.,1.,0.));
#25170=CARTESIAN_POINT('',(-1.4,2.2,1.71450551880629E-16));
#25171=CARTESIAN_POINT('Origin',(0.,2.2,0.));
#25172=CARTESIAN_POINT('',(-1.4,1.,1.71450551880629E-16));
#25173=CARTESIAN_POINT('',(-1.4,1.,1.71450551880629E-16));
#25174=CARTESIAN_POINT('Origin',(0.,1.,0.));
#25175=CARTESIAN_POINT('Origin',(0.,2.2,0.));
#25176=CARTESIAN_POINT('Ctrl Pts',(2.11275013067528,-1.,0.613422273260091));
#25177=CARTESIAN_POINT('Ctrl Pts',(2.11275013067528,1.,0.613422273260091));
#25178=CARTESIAN_POINT('Ctrl Pts',(2.11187554260142,-1.,0.61246736556225));
#25179=CARTESIAN_POINT('Ctrl Pts',(2.11187554260142,1.,0.61246736556225));
#25180=CARTESIAN_POINT('Ctrl Pts',(2.11012443807661,-1.,0.610560911691114));
#25181=CARTESIAN_POINT('Ctrl Pts',(2.11012443807661,1.,0.610560911691114));
#25182=CARTESIAN_POINT('Ctrl Pts',(2.10749199615859,-1.,0.607711315456826));
#25183=CARTESIAN_POINT('Ctrl Pts',(2.10749199615859,1.,0.607711315456826));
#25184=CARTESIAN_POINT('Ctrl Pts',(2.10397049887709,-1.,0.603932030738212));
#25185=CARTESIAN_POINT('Ctrl Pts',(2.10397049887709,1.,0.603932030738212));
#25186=CARTESIAN_POINT('Ctrl Pts',(2.09954930865331,-1.,0.599241616422144));
#25187=CARTESIAN_POINT('Ctrl Pts',(2.09954930865331,1.,0.599241616422144));
#25188=CARTESIAN_POINT('Ctrl Pts',(2.09510876220501,-1.,0.594585006052824));
#25189=CARTESIAN_POINT('Ctrl Pts',(2.09510876220501,1.,0.594585006052824));
#25190=CARTESIAN_POINT('Ctrl Pts',(2.09064881812053,-1.,0.58996236540319));
#25191=CARTESIAN_POINT('Ctrl Pts',(2.09064881812053,1.,0.58996236540319));
#25192=CARTESIAN_POINT('Ctrl Pts',(2.086169437277,-1.,0.585373918990895));
#25193=CARTESIAN_POINT('Ctrl Pts',(2.086169437277,1.,0.585373918990895));
#25194=CARTESIAN_POINT('Ctrl Pts',(2.08167059018138,-1.,0.580819952107257));
#25195=CARTESIAN_POINT('Ctrl Pts',(2.08167059018138,1.,0.580819952107257));
#25196=CARTESIAN_POINT('Ctrl Pts',(2.07715226767361,-1.,0.576300797416275));
#25197=CARTESIAN_POINT('Ctrl Pts',(2.07715226767361,1.,0.576300797416275));
#25198=CARTESIAN_POINT('Ctrl Pts',(2.07261449292757,-1.,0.571816823242411));
#25199=CARTESIAN_POINT('Ctrl Pts',(2.07261449292757,1.,0.571816823242411));
#25200=CARTESIAN_POINT('Ctrl Pts',(2.06805732997383,-1.,0.56736842118123));
#25201=CARTESIAN_POINT('Ctrl Pts',(2.06805732997383,1.,0.56736842118123));
#25202=CARTESIAN_POINT('Ctrl Pts',(2.06348090160697,-1.,0.562955993082574));
#25203=CARTESIAN_POINT('Ctrl Pts',(2.06348090160697,1.,0.562955993082574));
#25204=CARTESIAN_POINT('Ctrl Pts',(2.05888537756571,-1.,0.558579940185468));
#25205=CARTESIAN_POINT('Ctrl Pts',(2.05888537756571,1.,0.558579940185468));
#25206=CARTESIAN_POINT('Ctrl Pts',(2.05427091604482,-1.,0.55424065746411));
#25207=CARTESIAN_POINT('Ctrl Pts',(2.05427091604482,1.,0.55424065746411));
#25208=CARTESIAN_POINT('Ctrl Pts',(2.04963761077974,-1.,0.549938525150342));
#25209=CARTESIAN_POINT('Ctrl Pts',(2.04963761077974,1.,0.549938525150342));
#25210=CARTESIAN_POINT('Ctrl Pts',(2.0449854471456,-1.,0.545673903817349));
#25211=CARTESIAN_POINT('Ctrl Pts',(2.0449854471456,1.,0.545673903817349));
#25212=CARTESIAN_POINT('Ctrl Pts',(2.0403142269048,-1.,0.54144712061552));
#25213=CARTESIAN_POINT('Ctrl Pts',(2.0403142269048,1.,0.54144712061552));
#25214=CARTESIAN_POINT('Ctrl Pts',(2.03562362953993,-1.,0.537258489833135));
#25215=CARTESIAN_POINT('Ctrl Pts',(2.03562362953993,1.,0.537258489833135));
#25216=CARTESIAN_POINT('Ctrl Pts',(2.03091336214401,-1.,0.533108355132905));
#25217=CARTESIAN_POINT('Ctrl Pts',(2.03091336214401,1.,0.533108355132905));
#25218=CARTESIAN_POINT('Ctrl Pts',(2.02618329083289,-1.,0.528997127241911));
#25219=CARTESIAN_POINT('Ctrl Pts',(2.02618329083289,1.,0.528997127241911));
#25220=CARTESIAN_POINT('Ctrl Pts',(2.02143356304712,-1.,0.524925318333519));
#25221=CARTESIAN_POINT('Ctrl Pts',(2.02143356304712,1.,0.524925318333519));
#25222=CARTESIAN_POINT('Ctrl Pts',(2.01666477917305,-1.,0.520893590399429));
#25223=CARTESIAN_POINT('Ctrl Pts',(2.01666477917305,1.,0.520893590399429));
#25224=CARTESIAN_POINT('Ctrl Pts',(2.01187773939257,-1.,0.516902681728733));
#25225=CARTESIAN_POINT('Ctrl Pts',(2.01187773939257,1.,0.516902681728733));
#25226=CARTESIAN_POINT('Ctrl Pts',(2.00707309946955,-1.,0.512953306961814));
#25227=CARTESIAN_POINT('Ctrl Pts',(2.00707309946955,1.,0.512953306961814));
#25228=CARTESIAN_POINT('Ctrl Pts',(2.00225107134733,-1.,0.509046069886152));
#25229=CARTESIAN_POINT('Ctrl Pts',(2.00225107134733,1.,0.509046069886152));
#25230=CARTESIAN_POINT('Ctrl Pts',(1.99741107463567,-1.,0.505181361323011));
#25231=CARTESIAN_POINT('Ctrl Pts',(1.99741107463567,1.,0.505181361323011));
#25232=CARTESIAN_POINT('Ctrl Pts',(1.9925514912615,-1.,0.501359287727129));
#25233=CARTESIAN_POINT('Ctrl Pts',(1.9925514912615,1.,0.501359287727129));
#25234=CARTESIAN_POINT('Ctrl Pts',(1.98767044752929,-1.,0.497579909545564));
#25235=CARTESIAN_POINT('Ctrl Pts',(1.98767044752929,1.,0.497579909545564));
#25236=CARTESIAN_POINT('Ctrl Pts',(1.9827665876182,-1.,0.493843476541493));
#25237=CARTESIAN_POINT('Ctrl Pts',(1.9827665876182,1.,0.493843476541493));
#25238=CARTESIAN_POINT('Ctrl Pts',(1.97783973019229,-1.,0.490150627860955));
#25239=CARTESIAN_POINT('Ctrl Pts',(1.97783973019229,1.,0.490150627860955));
#25240=CARTESIAN_POINT('Ctrl Pts',(1.97289186263272,-1.,0.486502692907661));
#25241=CARTESIAN_POINT('Ctrl Pts',(1.97289186263272,1.,0.486502692907661));
#25242=CARTESIAN_POINT('Ctrl Pts',(1.96792703422358,-1.,0.482901662120687));
#25243=CARTESIAN_POINT('Ctrl Pts',(1.96792703422358,1.,0.482901662120687));
#25244=CARTESIAN_POINT('Ctrl Pts',(1.96294933055938,-1.,0.479349583074846));
#25245=CARTESIAN_POINT('Ctrl Pts',(1.96294933055938,1.,0.479349583074846));
#25246=CARTESIAN_POINT('Ctrl Pts',(1.95796111148175,-1.,0.475848034683172));
#25247=CARTESIAN_POINT('Ctrl Pts',(1.95796111148175,1.,0.475848034683172));
#25248=CARTESIAN_POINT('Ctrl Pts',(1.95296148278136,-1.,0.47239767226408));
#25249=CARTESIAN_POINT('Ctrl Pts',(1.95296148278136,1.,0.47239767226408));
#25250=CARTESIAN_POINT('Ctrl Pts',(1.94794381136524,-1.,0.468997482913158));
#25251=CARTESIAN_POINT('Ctrl Pts',(1.94794381136524,1.,0.468997482913158));
#25252=CARTESIAN_POINT('Ctrl Pts',(1.94289794196205,-1.,0.465645462026065));
#25253=CARTESIAN_POINT('Ctrl Pts',(1.94289794196205,1.,0.465645462026065));
#25254=CARTESIAN_POINT('Ctrl Pts',(1.93781486640834,-1.,0.462340031009087));
#25255=CARTESIAN_POINT('Ctrl Pts',(1.93781486640834,1.,0.462340031009087));
#25256=CARTESIAN_POINT('Ctrl Pts',(1.93269066517936,-1.,0.459081234547932));
#25257=CARTESIAN_POINT('Ctrl Pts',(1.93269066517936,1.,0.459081234547932));
#25258=CARTESIAN_POINT('Ctrl Pts',(1.92753067150461,-1.,0.455872005174336));
#25259=CARTESIAN_POINT('Ctrl Pts',(1.92753067150461,1.,0.455872005174336));
#25260=CARTESIAN_POINT('Ctrl Pts',(1.9223538064847,-1.,0.452719478359356));
#25261=CARTESIAN_POINT('Ctrl Pts',(1.9223538064847,1.,0.452719478359356));
#25262=CARTESIAN_POINT('Ctrl Pts',(1.91718342555717,-1.,0.449632260106572));
#25263=CARTESIAN_POINT('Ctrl Pts',(1.91718342555717,1.,0.449632260106572));
#25264=CARTESIAN_POINT('Ctrl Pts',(1.91203699981095,-1.,0.446617343485651));
#25265=CARTESIAN_POINT('Ctrl Pts',(1.91203699981095,1.,0.446617343485651));
#25266=CARTESIAN_POINT('Ctrl Pts',(1.90691756144906,-1.,0.443677556849171));
#25267=CARTESIAN_POINT('Ctrl Pts',(1.90691756144906,1.,0.443677556849171));
#25268=CARTESIAN_POINT('Ctrl Pts',(1.90180124389137,-1.,0.440807833704161));
#25269=CARTESIAN_POINT('Ctrl Pts',(1.90180124389137,1.,0.440807833704161));
#25270=CARTESIAN_POINT('Ctrl Pts',(1.89663648956549,-1.,0.437995003948443));
#25271=CARTESIAN_POINT('Ctrl Pts',(1.89663648956549,1.,0.437995003948443));
#25272=CARTESIAN_POINT('Ctrl Pts',(1.89136993975585,-1.,0.43522566096358));
#25273=CARTESIAN_POINT('Ctrl Pts',(1.89136993975585,1.,0.43522566096358));
#25274=CARTESIAN_POINT('Ctrl Pts',(1.88596913666828,-1.,0.432493038548833));
#25275=CARTESIAN_POINT('Ctrl Pts',(1.88596913666828,1.,0.432493038548833));
#25276=CARTESIAN_POINT('Ctrl Pts',(1.88044229001778,-1.,0.429803062482217));
#25277=CARTESIAN_POINT('Ctrl Pts',(1.88044229001778,1.,0.429803062482217));
#25278=CARTESIAN_POINT('Ctrl Pts',(1.87486989291333,-1.,0.427183828518743));
#25279=CARTESIAN_POINT('Ctrl Pts',(1.87486989291333,1.,0.427183828518743));
#25280=CARTESIAN_POINT('Ctrl Pts',(1.8693780394412,-1.,0.424678177290876));
#25281=CARTESIAN_POINT('Ctrl Pts',(1.8693780394412,1.,0.424678177290876));
#25282=CARTESIAN_POINT('Ctrl Pts',(1.86408083333863,-1.,0.422327307417885));
#25283=CARTESIAN_POINT('Ctrl Pts',(1.86408083333863,1.,0.422327307417885));
#25284=CARTESIAN_POINT('Ctrl Pts',(1.8590328109667,-1.,0.420157287975583));
#25285=CARTESIAN_POINT('Ctrl Pts',(1.8590328109667,1.,0.420157287975583));
#25286=CARTESIAN_POINT('Ctrl Pts',(1.8541763285645,-1.,0.418164129144046));
#25287=CARTESIAN_POINT('Ctrl Pts',(1.8541763285645,1.,0.418164129144046));
#25288=CARTESIAN_POINT('Ctrl Pts',(1.84929312930314,-1.,0.416300022039885));
#25289=CARTESIAN_POINT('Ctrl Pts',(1.84929312930314,1.,0.416300022039885));
#25290=CARTESIAN_POINT('Ctrl Pts',(1.84405757074218,-1.,0.414487438255542));
#25291=CARTESIAN_POINT('Ctrl Pts',(1.84405757074218,1.,0.414487438255542));
#25292=CARTESIAN_POINT('Ctrl Pts',(1.8380895347617,-1.,0.412633125322945));
#25293=CARTESIAN_POINT('Ctrl Pts',(1.8380895347617,1.,0.412633125322945));
#25294=CARTESIAN_POINT('Ctrl Pts',(1.83100408895047,-1.,0.410641256301276));
#25295=CARTESIAN_POINT('Ctrl Pts',(1.83100408895047,1.,0.410641256301276));
#25296=CARTESIAN_POINT('Ctrl Pts',(1.82247022677562,-1.,0.408428948106228));
#25297=CARTESIAN_POINT('Ctrl Pts',(1.82247022677562,1.,0.408428948106228));
#25298=CARTESIAN_POINT('Ctrl Pts',(1.81223801812013,-1.,0.405933518407176));
#25299=CARTESIAN_POINT('Ctrl Pts',(1.81223801812013,1.,0.405933518407176));
#25300=CARTESIAN_POINT('Ctrl Pts',(1.80012077173238,-1.,0.403107976163396));
#25301=CARTESIAN_POINT('Ctrl Pts',(1.80012077173238,1.,0.403107976163396));
#25302=CARTESIAN_POINT('Ctrl Pts',(1.78598826343754,-1.,0.399919403774156));
#25303=CARTESIAN_POINT('Ctrl Pts',(1.78598826343754,1.,0.399919403774156));
#25304=CARTESIAN_POINT('Ctrl Pts',(1.76975560043442,-1.,0.396346196110688));
#25305=CARTESIAN_POINT('Ctrl Pts',(1.76975560043442,1.,0.396346196110688));
#25306=CARTESIAN_POINT('Ctrl Pts',(1.75137405310193,-1.,0.392375812285396));
#25307=CARTESIAN_POINT('Ctrl Pts',(1.75137405310193,1.,0.392375812285396));
#25308=CARTESIAN_POINT('Ctrl Pts',(1.73493170972829,-1.,0.388877023502615));
#25309=CARTESIAN_POINT('Ctrl Pts',(1.73493170972829,1.,0.388877023502615));
#25310=CARTESIAN_POINT('Ctrl Pts',(1.72162022244582,-1.,0.386070790323281));
#25311=CARTESIAN_POINT('Ctrl Pts',(1.72162022244582,1.,0.386070790323281));
#25312=CARTESIAN_POINT('Ctrl Pts',(1.71231062891398,-1.,0.384119047314215));
#25313=CARTESIAN_POINT('Ctrl Pts',(1.71231062891398,1.,0.384119047314215));
#25314=CARTESIAN_POINT('Ctrl Pts',(1.7075470150345,-1.,0.383122945602004));
#25315=CARTESIAN_POINT('Ctrl Pts',(1.7075470150345,1.,0.383122945602004));
#25316=CARTESIAN_POINT('',(1.7075470150345,1.,0.383122945602004));
#25317=CARTESIAN_POINT('',(1.7075470150345,0.,0.383122945602005));
#25318=CARTESIAN_POINT('',(2.11275013067528,1.,0.613422273260091));
#25319=CARTESIAN_POINT('Ctrl Pts',(2.11275013067528,1.,0.613422273260091));
#25320=CARTESIAN_POINT('Ctrl Pts',(2.11187554260142,1.,0.61246736556225));
#25321=CARTESIAN_POINT('Ctrl Pts',(2.11012443807661,1.,0.610560911691114));
#25322=CARTESIAN_POINT('Ctrl Pts',(2.10749199615859,1.,0.607711315456826));
#25323=CARTESIAN_POINT('Ctrl Pts',(2.10397049887709,1.,0.603932030738212));
#25324=CARTESIAN_POINT('Ctrl Pts',(2.09954930865331,1.,0.599241616422144));
#25325=CARTESIAN_POINT('Ctrl Pts',(2.09510876220501,1.,0.594585006052824));
#25326=CARTESIAN_POINT('Ctrl Pts',(2.09064881812053,1.,0.58996236540319));
#25327=CARTESIAN_POINT('Ctrl Pts',(2.086169437277,1.,0.585373918990895));
#25328=CARTESIAN_POINT('Ctrl Pts',(2.08167059018138,1.,0.580819952107257));
#25329=CARTESIAN_POINT('Ctrl Pts',(2.07715226767361,1.,0.576300797416275));
#25330=CARTESIAN_POINT('Ctrl Pts',(2.07261449292757,1.,0.571816823242411));
#25331=CARTESIAN_POINT('Ctrl Pts',(2.06805732997383,1.,0.56736842118123));
#25332=CARTESIAN_POINT('Ctrl Pts',(2.06348090160697,1.,0.562955993082574));
#25333=CARTESIAN_POINT('Ctrl Pts',(2.05888537756571,1.,0.558579940185468));
#25334=CARTESIAN_POINT('Ctrl Pts',(2.05427091604482,1.,0.55424065746411));
#25335=CARTESIAN_POINT('Ctrl Pts',(2.04963761077974,1.,0.549938525150342));
#25336=CARTESIAN_POINT('Ctrl Pts',(2.0449854471456,1.,0.545673903817349));
#25337=CARTESIAN_POINT('Ctrl Pts',(2.0403142269048,1.,0.54144712061552));
#25338=CARTESIAN_POINT('Ctrl Pts',(2.03562362953993,1.,0.537258489833135));
#25339=CARTESIAN_POINT('Ctrl Pts',(2.03091336214401,1.,0.533108355132905));
#25340=CARTESIAN_POINT('Ctrl Pts',(2.02618329083289,1.,0.528997127241911));
#25341=CARTESIAN_POINT('Ctrl Pts',(2.02143356304712,1.,0.524925318333519));
#25342=CARTESIAN_POINT('Ctrl Pts',(2.01666477917305,1.,0.520893590399429));
#25343=CARTESIAN_POINT('Ctrl Pts',(2.01187773939257,1.,0.516902681728733));
#25344=CARTESIAN_POINT('Ctrl Pts',(2.00707309946955,1.,0.512953306961814));
#25345=CARTESIAN_POINT('Ctrl Pts',(2.00225107134733,1.,0.509046069886152));
#25346=CARTESIAN_POINT('Ctrl Pts',(1.99741107463567,1.,0.505181361323011));
#25347=CARTESIAN_POINT('Ctrl Pts',(1.9925514912615,1.,0.501359287727129));
#25348=CARTESIAN_POINT('Ctrl Pts',(1.98767044752929,1.,0.497579909545564));
#25349=CARTESIAN_POINT('Ctrl Pts',(1.9827665876182,1.,0.493843476541493));
#25350=CARTESIAN_POINT('Ctrl Pts',(1.97783973019229,1.,0.490150627860955));
#25351=CARTESIAN_POINT('Ctrl Pts',(1.97289186263272,1.,0.486502692907661));
#25352=CARTESIAN_POINT('Ctrl Pts',(1.96792703422358,1.,0.482901662120687));
#25353=CARTESIAN_POINT('Ctrl Pts',(1.96294933055938,1.,0.479349583074846));
#25354=CARTESIAN_POINT('Ctrl Pts',(1.95796111148175,1.,0.475848034683172));
#25355=CARTESIAN_POINT('Ctrl Pts',(1.95296148278136,1.,0.47239767226408));
#25356=CARTESIAN_POINT('Ctrl Pts',(1.94794381136524,1.,0.468997482913158));
#25357=CARTESIAN_POINT('Ctrl Pts',(1.94289794196205,1.,0.465645462026065));
#25358=CARTESIAN_POINT('Ctrl Pts',(1.93781486640834,1.,0.462340031009087));
#25359=CARTESIAN_POINT('Ctrl Pts',(1.93269066517936,1.,0.459081234547932));
#25360=CARTESIAN_POINT('Ctrl Pts',(1.92753067150461,1.,0.455872005174336));
#25361=CARTESIAN_POINT('Ctrl Pts',(1.9223538064847,1.,0.452719478359356));
#25362=CARTESIAN_POINT('Ctrl Pts',(1.91718342555717,1.,0.449632260106572));
#25363=CARTESIAN_POINT('Ctrl Pts',(1.91203699981095,1.,0.446617343485651));
#25364=CARTESIAN_POINT('Ctrl Pts',(1.90691756144906,1.,0.443677556849171));
#25365=CARTESIAN_POINT('Ctrl Pts',(1.90180124389137,1.,0.440807833704161));
#25366=CARTESIAN_POINT('Ctrl Pts',(1.89663648956549,1.,0.437995003948443));
#25367=CARTESIAN_POINT('Ctrl Pts',(1.89136993975585,1.,0.43522566096358));
#25368=CARTESIAN_POINT('Ctrl Pts',(1.88596913666828,1.,0.432493038548833));
#25369=CARTESIAN_POINT('Ctrl Pts',(1.88044229001778,1.,0.429803062482217));
#25370=CARTESIAN_POINT('Ctrl Pts',(1.87486989291333,1.,0.427183828518743));
#25371=CARTESIAN_POINT('Ctrl Pts',(1.8693780394412,1.,0.424678177290876));
#25372=CARTESIAN_POINT('Ctrl Pts',(1.86408083333863,1.,0.422327307417885));
#25373=CARTESIAN_POINT('Ctrl Pts',(1.8590328109667,1.,0.420157287975583));
#25374=CARTESIAN_POINT('Ctrl Pts',(1.8541763285645,1.,0.418164129144046));
#25375=CARTESIAN_POINT('Ctrl Pts',(1.84929312930314,1.,0.416300022039885));
#25376=CARTESIAN_POINT('Ctrl Pts',(1.84405757074218,1.,0.414487438255542));
#25377=CARTESIAN_POINT('Ctrl Pts',(1.8380895347617,1.,0.412633125322945));
#25378=CARTESIAN_POINT('Ctrl Pts',(1.83100408895047,1.,0.410641256301276));
#25379=CARTESIAN_POINT('Ctrl Pts',(1.82247022677562,1.,0.408428948106228));
#25380=CARTESIAN_POINT('Ctrl Pts',(1.81223801812013,1.,0.405933518407176));
#25381=CARTESIAN_POINT('Ctrl Pts',(1.80012077173238,1.,0.403107976163396));
#25382=CARTESIAN_POINT('Ctrl Pts',(1.78598826343754,1.,0.399919403774156));
#25383=CARTESIAN_POINT('Ctrl Pts',(1.76975560043442,1.,0.396346196110688));
#25384=CARTESIAN_POINT('Ctrl Pts',(1.75137405310193,1.,0.392375812285396));
#25385=CARTESIAN_POINT('Ctrl Pts',(1.73493170972829,1.,0.388877023502615));
#25386=CARTESIAN_POINT('Ctrl Pts',(1.72162022244582,1.,0.386070790323281));
#25387=CARTESIAN_POINT('Ctrl Pts',(1.71231062891398,1.,0.384119047314215));
#25388=CARTESIAN_POINT('Ctrl Pts',(1.7075470150345,1.,0.383122945602004));
#25389=CARTESIAN_POINT('',(2.11275013067528,0.,0.613422273260091));
#25390=CARTESIAN_POINT('Origin',(2.0698113262342,0.,0.745574324794401));
#25391=CARTESIAN_POINT('',(2.0698113262342,1.,0.745574324794401));
#25392=CARTESIAN_POINT('',(2.11275013067528,1.,0.613422273260091));
#25393=CARTESIAN_POINT('',(2.0698113262342,0.,0.745574324794401));
#25394=CARTESIAN_POINT('Ctrl Pts',(1.60662857109684,-1.,0.693717979106306));
#25395=CARTESIAN_POINT('Ctrl Pts',(1.60662857109684,1.,0.693717979106306));
#25396=CARTESIAN_POINT('Ctrl Pts',(1.61106790958151,-1.,0.695712097881194));
#25397=CARTESIAN_POINT('Ctrl Pts',(1.61106790958151,1.,0.695712097881194));
#25398=CARTESIAN_POINT('Ctrl Pts',(1.61974673472612,-1.,0.699605146405088));
#25399=CARTESIAN_POINT('Ctrl Pts',(1.61974673472612,1.,0.699605146405088));
#25400=CARTESIAN_POINT('Ctrl Pts',(1.63216541664676,-1.,0.705159151988319));
#25401=CARTESIAN_POINT('Ctrl Pts',(1.63216541664676,1.,0.705159151988319));
#25402=CARTESIAN_POINT('Ctrl Pts',(1.64752408832016,-1.,0.711993139355394));
#25403=CARTESIAN_POINT('Ctrl Pts',(1.64752408832016,1.,0.711993139355394));
#25404=CARTESIAN_POINT('Ctrl Pts',(1.6647288055568,-1.,0.719585433804282));
#25405=CARTESIAN_POINT('Ctrl Pts',(1.6647288055568,1.,0.719585433804282));
#25406=CARTESIAN_POINT('Ctrl Pts',(1.67996158455503,-1.,0.726235967997433));
#25407=CARTESIAN_POINT('Ctrl Pts',(1.67996158455503,1.,0.726235967997433));
#25408=CARTESIAN_POINT('Ctrl Pts',(1.69326921975743,-1.,0.731963238697195));
#25409=CARTESIAN_POINT('Ctrl Pts',(1.69326921975743,1.,0.731963238697195));
#25410=CARTESIAN_POINT('Ctrl Pts',(1.70473309006121,-1.,0.736799665724771));
#25411=CARTESIAN_POINT('Ctrl Pts',(1.70473309006121,1.,0.736799665724771));
#25412=CARTESIAN_POINT('Ctrl Pts',(1.71447789751927,-1.,0.740795162032088));
#25413=CARTESIAN_POINT('Ctrl Pts',(1.71447789751927,1.,0.740795162032088));
#25414=CARTESIAN_POINT('Ctrl Pts',(1.7226822991693,-1.,0.744021445433765));
#25415=CARTESIAN_POINT('Ctrl Pts',(1.7226822991693,1.,0.744021445433765));
#25416=CARTESIAN_POINT('Ctrl Pts',(1.72958533647399,-1.,0.746574710096437));
#25417=CARTESIAN_POINT('Ctrl Pts',(1.72958533647399,1.,0.746574710096437));
#25418=CARTESIAN_POINT('Ctrl Pts',(1.73550351679848,-1.,0.748582462954855));
#25419=CARTESIAN_POINT('Ctrl Pts',(1.73550351679848,1.,0.748582462954855));
#25420=CARTESIAN_POINT('Ctrl Pts',(1.74080458266705,-1.,0.750193435979541));
#25421=CARTESIAN_POINT('Ctrl Pts',(1.74080458266705,1.,0.750193435979541));
#25422=CARTESIAN_POINT('Ctrl Pts',(1.74585086852298,-1.,0.751555614163629));
#25423=CARTESIAN_POINT('Ctrl Pts',(1.74585086852298,1.,0.751555614163629));
#25424=CARTESIAN_POINT('Ctrl Pts',(1.75095139468809,-1.,0.752797683531377));
#25425=CARTESIAN_POINT('Ctrl Pts',(1.75095139468809,1.,0.752797683531377));
#25426=CARTESIAN_POINT('Ctrl Pts',(1.75631083600175,-1.,0.75400925402848));
#25427=CARTESIAN_POINT('Ctrl Pts',(1.75631083600175,1.,0.75400925402848));
#25428=CARTESIAN_POINT('Ctrl Pts',(1.7619781724032,-1.,0.755220979975262));
#25429=CARTESIAN_POINT('Ctrl Pts',(1.7619781724032,1.,0.755220979975262));
#25430=CARTESIAN_POINT('Ctrl Pts',(1.76789396003141,-1.,0.756421896028403));
#25431=CARTESIAN_POINT('Ctrl Pts',(1.76789396003141,1.,0.756421896028403));
#25432=CARTESIAN_POINT('Ctrl Pts',(1.77394167108342,-1.,0.757578264077238));
#25433=CARTESIAN_POINT('Ctrl Pts',(1.77394167108342,1.,0.757578264077238));
#25434=CARTESIAN_POINT('Ctrl Pts',(1.77999411220912,-1.,0.75865062667738));
#25435=CARTESIAN_POINT('Ctrl Pts',(1.77999411220912,1.,0.75865062667738));
#25436=CARTESIAN_POINT('Ctrl Pts',(1.78596964884526,-1.,0.759614401109868));
#25437=CARTESIAN_POINT('Ctrl Pts',(1.78596964884526,1.,0.759614401109868));
#25438=CARTESIAN_POINT('Ctrl Pts',(1.79185815610802,-1.,0.760469555880425));
#25439=CARTESIAN_POINT('Ctrl Pts',(1.79185815610802,1.,0.760469555880425));
#25440=CARTESIAN_POINT('Ctrl Pts',(1.79768986997735,-1.,0.761229695230359));
#25441=CARTESIAN_POINT('Ctrl Pts',(1.79768986997735,1.,0.761229695230359));
#25442=CARTESIAN_POINT('Ctrl Pts',(1.80351583877334,-1.,0.761915336443516));
#25443=CARTESIAN_POINT('Ctrl Pts',(1.80351583877334,1.,0.761915336443516));
#25444=CARTESIAN_POINT('Ctrl Pts',(1.80938551463989,-1.,0.762546129464036));
#25445=CARTESIAN_POINT('Ctrl Pts',(1.80938551463989,1.,0.762546129464036));
#25446=CARTESIAN_POINT('Ctrl Pts',(1.81532118405566,-1.,0.763132003836783));
#25447=CARTESIAN_POINT('Ctrl Pts',(1.81532118405566,1.,0.763132003836783));
#25448=CARTESIAN_POINT('Ctrl Pts',(1.82131873145297,-1.,0.763673465462854));
#25449=CARTESIAN_POINT('Ctrl Pts',(1.82131873145297,1.,0.763673465462854));
#25450=CARTESIAN_POINT('Ctrl Pts',(1.8273599120008,-1.,0.764165902606056));
#25451=CARTESIAN_POINT('Ctrl Pts',(1.8273599120008,1.,0.764165902606056));
#25452=CARTESIAN_POINT('Ctrl Pts',(1.8334207722714,-1.,0.764602549687846));
#25453=CARTESIAN_POINT('Ctrl Pts',(1.8334207722714,1.,0.764602549687846));
#25454=CARTESIAN_POINT('Ctrl Pts',(1.83948181064823,-1.,0.764978057881688));
#25455=CARTESIAN_POINT('Ctrl Pts',(1.83948181064823,1.,0.764978057881688));
#25456=CARTESIAN_POINT('Ctrl Pts',(1.8455369887591,-1.,0.765291664861972));
#25457=CARTESIAN_POINT('Ctrl Pts',(1.8455369887591,1.,0.765291664861972));
#25458=CARTESIAN_POINT('Ctrl Pts',(1.85158945130054,-1.,0.765545710619023));
#25459=CARTESIAN_POINT('Ctrl Pts',(1.85158945130054,1.,0.765545710619023));
#25460=CARTESIAN_POINT('Ctrl Pts',(1.85764741390391,-1.,0.765744212909305));
#25461=CARTESIAN_POINT('Ctrl Pts',(1.85764741390391,1.,0.765744212909305));
#25462=CARTESIAN_POINT('Ctrl Pts',(1.86372027063314,-1.,0.765891519092557));
#25463=CARTESIAN_POINT('Ctrl Pts',(1.86372027063314,1.,0.765891519092557));
#25464=CARTESIAN_POINT('Ctrl Pts',(1.86981398314345,-1.,0.765990708546112));
#25465=CARTESIAN_POINT('Ctrl Pts',(1.86981398314345,1.,0.765990708546112));
#25466=CARTESIAN_POINT('Ctrl Pts',(1.87592888967886,-1.,0.766042837036759));
#25467=CARTESIAN_POINT('Ctrl Pts',(1.87592888967886,1.,0.766042837036759));
#25468=CARTESIAN_POINT('Ctrl Pts',(1.88206215302561,-1.,0.766047794851869));
#25469=CARTESIAN_POINT('Ctrl Pts',(1.88206215302561,1.,0.766047794851869));
#25470=CARTESIAN_POINT('Ctrl Pts',(1.88820926433409,-1.,0.76600483706209));
#25471=CARTESIAN_POINT('Ctrl Pts',(1.88820926433409,1.,0.76600483706209));
#25472=CARTESIAN_POINT('Ctrl Pts',(1.89436577771389,-1.,0.765913193856979));
#25473=CARTESIAN_POINT('Ctrl Pts',(1.89436577771389,1.,0.765913193856979));
#25474=CARTESIAN_POINT('Ctrl Pts',(1.90052930393599,-1.,0.765772772593395));
#25475=CARTESIAN_POINT('Ctrl Pts',(1.90052930393599,1.,0.765772772593395));
#25476=CARTESIAN_POINT('Ctrl Pts',(1.90669961402362,-1.,0.765584196937937));
#25477=CARTESIAN_POINT('Ctrl Pts',(1.90669961402362,1.,0.765584196937937));
#25478=CARTESIAN_POINT('Ctrl Pts',(1.91287765805174,-1.,0.765348465884739));
#25479=CARTESIAN_POINT('Ctrl Pts',(1.91287765805174,1.,0.765348465884739));
#25480=CARTESIAN_POINT('Ctrl Pts',(1.91906491634197,-1.,0.765066729667095));
#25481=CARTESIAN_POINT('Ctrl Pts',(1.91906491634197,1.,0.765066729667095));
#25482=CARTESIAN_POINT('Ctrl Pts',(1.92526263537041,-1.,0.764740025488189));
#25483=CARTESIAN_POINT('Ctrl Pts',(1.92526263537041,1.,0.764740025488189));
#25484=CARTESIAN_POINT('Ctrl Pts',(1.93147105496367,-1.,0.76436901067389));
#25485=CARTESIAN_POINT('Ctrl Pts',(1.93147105496367,1.,0.76436901067389));
#25486=CARTESIAN_POINT('Ctrl Pts',(1.93768964875867,-1.,0.763954049121394));
#25487=CARTESIAN_POINT('Ctrl Pts',(1.93768964875867,1.,0.763954049121394));
#25488=CARTESIAN_POINT('Ctrl Pts',(1.94391746617626,-1.,0.763495333538581));
#25489=CARTESIAN_POINT('Ctrl Pts',(1.94391746617626,1.,0.763495333538581));
#25490=CARTESIAN_POINT('Ctrl Pts',(1.95015342590025,-1.,0.762992990878774));
#25491=CARTESIAN_POINT('Ctrl Pts',(1.95015342590025,1.,0.762992990878774));
#25492=CARTESIAN_POINT('Ctrl Pts',(1.95639665309893,-1.,0.762447203806264));
#25493=CARTESIAN_POINT('Ctrl Pts',(1.95639665309893,1.,0.762447203806264));
#25494=CARTESIAN_POINT('Ctrl Pts',(1.96264672744229,-1.,0.761858300014575));
#25495=CARTESIAN_POINT('Ctrl Pts',(1.96264672744229,1.,0.761858300014575));
#25496=CARTESIAN_POINT('Ctrl Pts',(1.96890351582545,-1.,0.761226690483986));
#25497=CARTESIAN_POINT('Ctrl Pts',(1.96890351582545,1.,0.761226690483986));
#25498=CARTESIAN_POINT('Ctrl Pts',(1.97516705321521,-1.,0.760552825409856));
#25499=CARTESIAN_POINT('Ctrl Pts',(1.97516705321521,1.,0.760552825409856));
#25500=CARTESIAN_POINT('Ctrl Pts',(1.98143741418156,-1.,0.759837147452135));
#25501=CARTESIAN_POINT('Ctrl Pts',(1.98143741418156,1.,0.759837147452135));
#25502=CARTESIAN_POINT('Ctrl Pts',(1.98771456680806,-1.,0.759080037802243));
#25503=CARTESIAN_POINT('Ctrl Pts',(1.98771456680806,1.,0.759080037802243));
#25504=CARTESIAN_POINT('Ctrl Pts',(1.9939983109871,-1.,0.758281796766377));
#25505=CARTESIAN_POINT('Ctrl Pts',(1.9939983109871,1.,0.758281796766377));
#25506=CARTESIAN_POINT('Ctrl Pts',(2.00028834739072,-1.,0.757442676862342));
#25507=CARTESIAN_POINT('Ctrl Pts',(2.00028834739072,1.,0.757442676862342));
#25508=CARTESIAN_POINT('Ctrl Pts',(2.00658431587682,-1.,0.756562904646496));
#25509=CARTESIAN_POINT('Ctrl Pts',(2.00658431587682,1.,0.756562904646496));
#25510=CARTESIAN_POINT('Ctrl Pts',(2.01288584328149,-1.,0.755642704958101));
#25511=CARTESIAN_POINT('Ctrl Pts',(2.01288584328149,1.,0.755642704958101));
#25512=CARTESIAN_POINT('Ctrl Pts',(2.01919259406003,-1.,0.75468233072352));
#25513=CARTESIAN_POINT('Ctrl Pts',(2.01919259406003,1.,0.75468233072352));
#25514=CARTESIAN_POINT('Ctrl Pts',(2.02550428623587,-1.,0.753682061113766));
#25515=CARTESIAN_POINT('Ctrl Pts',(2.02550428623587,1.,0.753682061113766));
#25516=CARTESIAN_POINT('Ctrl Pts',(2.03182068456467,-1.,0.752642180488104));
#25517=CARTESIAN_POINT('Ctrl Pts',(2.03182068456467,1.,0.752642180488104));
#25518=CARTESIAN_POINT('Ctrl Pts',(2.03814160092173,-1.,0.751562963361384));
#25519=CARTESIAN_POINT('Ctrl Pts',(2.03814160092173,1.,0.751562963361384));
#25520=CARTESIAN_POINT('Ctrl Pts',(2.04446689147754,-1.,0.750444657874758));
#25521=CARTESIAN_POINT('Ctrl Pts',(2.04446689147754,1.,0.750444657874758));
#25522=CARTESIAN_POINT('Ctrl Pts',(2.05079645591606,-1.,0.749287468663053));
#25523=CARTESIAN_POINT('Ctrl Pts',(2.05079645591606,1.,0.749287468663053));
#25524=CARTESIAN_POINT('Ctrl Pts',(2.05713023030263,-1.,0.748091554181101));
#25525=CARTESIAN_POINT('Ctrl Pts',(2.05713023030263,1.,0.748091554181101));
#25526=CARTESIAN_POINT('Ctrl Pts',(2.06220058927162,-1.,0.747103932785504));
#25527=CARTESIAN_POINT('Ctrl Pts',(2.06220058927162,1.,0.747103932785504));
#25528=CARTESIAN_POINT('Ctrl Pts',(2.06600523016401,-1.,0.746345871542696));
#25529=CARTESIAN_POINT('Ctrl Pts',(2.06600523016401,1.,0.746345871542696));
#25530=CARTESIAN_POINT('Ctrl Pts',(2.06854248895575,-1.,0.74583279137781));
#25531=CARTESIAN_POINT('Ctrl Pts',(2.06854248895575,1.,0.74583279137781));
#25532=CARTESIAN_POINT('Ctrl Pts',(2.0698113262342,-1.,0.745574324794401));
#25533=CARTESIAN_POINT('Ctrl Pts',(2.0698113262342,1.,0.745574324794401));
#25534=CARTESIAN_POINT('',(1.60662857109684,1.,0.693717979106306));
#25535=CARTESIAN_POINT('Ctrl Pts',(1.60662857109684,1.,0.693717979106306));
#25536=CARTESIAN_POINT('Ctrl Pts',(1.61106790958151,1.,0.695712097881194));
#25537=CARTESIAN_POINT('Ctrl Pts',(1.61974673472612,1.,0.699605146405088));
#25538=CARTESIAN_POINT('Ctrl Pts',(1.63216541664676,1.,0.705159151988319));
#25539=CARTESIAN_POINT('Ctrl Pts',(1.64752408832016,1.,0.711993139355394));
#25540=CARTESIAN_POINT('Ctrl Pts',(1.6647288055568,1.,0.719585433804282));
#25541=CARTESIAN_POINT('Ctrl Pts',(1.67996158455503,1.,0.726235967997433));
#25542=CARTESIAN_POINT('Ctrl Pts',(1.69326921975743,1.,0.731963238697195));
#25543=CARTESIAN_POINT('Ctrl Pts',(1.70473309006121,1.,0.736799665724771));
#25544=CARTESIAN_POINT('Ctrl Pts',(1.71447789751927,1.,0.740795162032088));
#25545=CARTESIAN_POINT('Ctrl Pts',(1.7226822991693,1.,0.744021445433765));
#25546=CARTESIAN_POINT('Ctrl Pts',(1.72958533647399,1.,0.746574710096437));
#25547=CARTESIAN_POINT('Ctrl Pts',(1.73550351679848,1.,0.748582462954855));
#25548=CARTESIAN_POINT('Ctrl Pts',(1.74080458266705,1.,0.750193435979541));
#25549=CARTESIAN_POINT('Ctrl Pts',(1.74585086852298,1.,0.751555614163629));
#25550=CARTESIAN_POINT('Ctrl Pts',(1.75095139468809,1.,0.752797683531377));
#25551=CARTESIAN_POINT('Ctrl Pts',(1.75631083600175,1.,0.75400925402848));
#25552=CARTESIAN_POINT('Ctrl Pts',(1.7619781724032,1.,0.755220979975262));
#25553=CARTESIAN_POINT('Ctrl Pts',(1.76789396003141,1.,0.756421896028403));
#25554=CARTESIAN_POINT('Ctrl Pts',(1.77394167108342,1.,0.757578264077238));
#25555=CARTESIAN_POINT('Ctrl Pts',(1.77999411220912,1.,0.75865062667738));
#25556=CARTESIAN_POINT('Ctrl Pts',(1.78596964884526,1.,0.759614401109868));
#25557=CARTESIAN_POINT('Ctrl Pts',(1.79185815610802,1.,0.760469555880425));
#25558=CARTESIAN_POINT('Ctrl Pts',(1.79768986997735,1.,0.761229695230359));
#25559=CARTESIAN_POINT('Ctrl Pts',(1.80351583877334,1.,0.761915336443516));
#25560=CARTESIAN_POINT('Ctrl Pts',(1.80938551463989,1.,0.762546129464036));
#25561=CARTESIAN_POINT('Ctrl Pts',(1.81532118405566,1.,0.763132003836783));
#25562=CARTESIAN_POINT('Ctrl Pts',(1.82131873145297,1.,0.763673465462854));
#25563=CARTESIAN_POINT('Ctrl Pts',(1.8273599120008,1.,0.764165902606056));
#25564=CARTESIAN_POINT('Ctrl Pts',(1.8334207722714,1.,0.764602549687846));
#25565=CARTESIAN_POINT('Ctrl Pts',(1.83948181064823,1.,0.764978057881688));
#25566=CARTESIAN_POINT('Ctrl Pts',(1.8455369887591,1.,0.765291664861972));
#25567=CARTESIAN_POINT('Ctrl Pts',(1.85158945130054,1.,0.765545710619023));
#25568=CARTESIAN_POINT('Ctrl Pts',(1.85764741390391,1.,0.765744212909305));
#25569=CARTESIAN_POINT('Ctrl Pts',(1.86372027063314,1.,0.765891519092557));
#25570=CARTESIAN_POINT('Ctrl Pts',(1.86981398314345,1.,0.765990708546112));
#25571=CARTESIAN_POINT('Ctrl Pts',(1.87592888967886,1.,0.766042837036759));
#25572=CARTESIAN_POINT('Ctrl Pts',(1.88206215302561,1.,0.766047794851869));
#25573=CARTESIAN_POINT('Ctrl Pts',(1.88820926433409,1.,0.76600483706209));
#25574=CARTESIAN_POINT('Ctrl Pts',(1.89436577771389,1.,0.765913193856979));
#25575=CARTESIAN_POINT('Ctrl Pts',(1.90052930393599,1.,0.765772772593395));
#25576=CARTESIAN_POINT('Ctrl Pts',(1.90669961402362,1.,0.765584196937937));
#25577=CARTESIAN_POINT('Ctrl Pts',(1.91287765805174,1.,0.765348465884739));
#25578=CARTESIAN_POINT('Ctrl Pts',(1.91906491634197,1.,0.765066729667095));
#25579=CARTESIAN_POINT('Ctrl Pts',(1.92526263537041,1.,0.764740025488189));
#25580=CARTESIAN_POINT('Ctrl Pts',(1.93147105496367,1.,0.76436901067389));
#25581=CARTESIAN_POINT('Ctrl Pts',(1.93768964875867,1.,0.763954049121394));
#25582=CARTESIAN_POINT('Ctrl Pts',(1.94391746617626,1.,0.763495333538581));
#25583=CARTESIAN_POINT('Ctrl Pts',(1.95015342590025,1.,0.762992990878774));
#25584=CARTESIAN_POINT('Ctrl Pts',(1.95639665309893,1.,0.762447203806264));
#25585=CARTESIAN_POINT('Ctrl Pts',(1.96264672744229,1.,0.761858300014575));
#25586=CARTESIAN_POINT('Ctrl Pts',(1.96890351582545,1.,0.761226690483986));
#25587=CARTESIAN_POINT('Ctrl Pts',(1.97516705321521,1.,0.760552825409856));
#25588=CARTESIAN_POINT('Ctrl Pts',(1.98143741418156,1.,0.759837147452135));
#25589=CARTESIAN_POINT('Ctrl Pts',(1.98771456680806,1.,0.759080037802243));
#25590=CARTESIAN_POINT('Ctrl Pts',(1.9939983109871,1.,0.758281796766377));
#25591=CARTESIAN_POINT('Ctrl Pts',(2.00028834739072,1.,0.757442676862342));
#25592=CARTESIAN_POINT('Ctrl Pts',(2.00658431587682,1.,0.756562904646496));
#25593=CARTESIAN_POINT('Ctrl Pts',(2.01288584328149,1.,0.755642704958101));
#25594=CARTESIAN_POINT('Ctrl Pts',(2.01919259406003,1.,0.75468233072352));
#25595=CARTESIAN_POINT('Ctrl Pts',(2.02550428623587,1.,0.753682061113766));
#25596=CARTESIAN_POINT('Ctrl Pts',(2.03182068456467,1.,0.752642180488104));
#25597=CARTESIAN_POINT('Ctrl Pts',(2.03814160092173,1.,0.751562963361384));
#25598=CARTESIAN_POINT('Ctrl Pts',(2.04446689147754,1.,0.750444657874758));
#25599=CARTESIAN_POINT('Ctrl Pts',(2.05079645591606,1.,0.749287468663053));
#25600=CARTESIAN_POINT('Ctrl Pts',(2.05713023030263,1.,0.748091554181101));
#25601=CARTESIAN_POINT('Ctrl Pts',(2.06220058927162,1.,0.747103932785504));
#25602=CARTESIAN_POINT('Ctrl Pts',(2.06600523016401,1.,0.746345871542696));
#25603=CARTESIAN_POINT('Ctrl Pts',(2.06854248895575,1.,0.74583279137781));
#25604=CARTESIAN_POINT('Ctrl Pts',(2.0698113262342,1.,0.745574324794401));
#25605=CARTESIAN_POINT('',(1.60662857109684,0.,0.693717979106305));
#25606=CARTESIAN_POINT('Origin',(0.,0.,0.));
#25607=CARTESIAN_POINT('',(1.5055822144029,1.,0.892032620296856));
#25608=CARTESIAN_POINT('Origin',(0.,1.,0.));
#25609=CARTESIAN_POINT('',(1.5055822144029,0.,0.892032620296855));
#25610=CARTESIAN_POINT('Ctrl Pts',(1.81978687191668,-1.,1.23627494547115));
#25611=CARTESIAN_POINT('Ctrl Pts',(1.81978687191668,1.,1.23627494547115));
#25612=CARTESIAN_POINT('Ctrl Pts',(1.81925017193666,-1.,1.23509651170476));
#25613=CARTESIAN_POINT('Ctrl Pts',(1.81925017193666,1.,1.23509651170476));
#25614=CARTESIAN_POINT('Ctrl Pts',(1.81817389921279,-1.,1.2327422452705));
#25615=CARTESIAN_POINT('Ctrl Pts',(1.81817389921279,1.,1.2327422452705));
#25616=CARTESIAN_POINT('Ctrl Pts',(1.8165508718364,-1.,1.2292186489137));
#25617=CARTESIAN_POINT('Ctrl Pts',(1.8165508718364,1.,1.2292186489137));
#25618=CARTESIAN_POINT('Ctrl Pts',(1.81436959210434,-1.,1.2245361330495));
#25619=CARTESIAN_POINT('Ctrl Pts',(1.81436959210434,1.,1.2245361330495));
#25620=CARTESIAN_POINT('Ctrl Pts',(1.81161420806656,-1.,1.21870906103557));
#25621=CARTESIAN_POINT('Ctrl Pts',(1.81161420806656,1.,1.21870906103557));
#25622=CARTESIAN_POINT('Ctrl Pts',(1.80882996917129,-1.,1.21290815708314));
#25623=CARTESIAN_POINT('Ctrl Pts',(1.80882996917129,1.,1.21290815708314));
#25624=CARTESIAN_POINT('Ctrl Pts',(1.80601678480707,-1.,1.20713356605475));
#25625=CARTESIAN_POINT('Ctrl Pts',(1.80601678480707,1.,1.20713356605475));
#25626=CARTESIAN_POINT('Ctrl Pts',(1.80317454838603,-1.,1.20138548938974));
#25627=CARTESIAN_POINT('Ctrl Pts',(1.80317454838603,1.,1.20138548938974));
#25628=CARTESIAN_POINT('Ctrl Pts',(1.80030314369879,-1.,1.19566418930242));
#25629=CARTESIAN_POINT('Ctrl Pts',(1.80030314369879,1.,1.19566418930242));
#25630=CARTESIAN_POINT('Ctrl Pts',(1.79740245923478,-1.,1.18996997934445));
#25631=CARTESIAN_POINT('Ctrl Pts',(1.79740245923478,1.,1.18996997934445));
#25632=CARTESIAN_POINT('Ctrl Pts',(1.79447240321515,-1.,1.18430321697432));
#25633=CARTESIAN_POINT('Ctrl Pts',(1.79447240321515,1.,1.18430321697432));
#25634=CARTESIAN_POINT('Ctrl Pts',(1.79151291552689,-1.,1.17866429440809));
#25635=CARTESIAN_POINT('Ctrl Pts',(1.79151291552689,1.,1.17866429440809));
#25636=CARTESIAN_POINT('Ctrl Pts',(1.78852398877616,-1.,1.17305363177328));
#25637=CARTESIAN_POINT('Ctrl Pts',(1.78852398877616,1.,1.17305363177328));
#25638=CARTESIAN_POINT('Ctrl Pts',(1.78550566040443,-1.,1.16747166312303));
#25639=CARTESIAN_POINT('Ctrl Pts',(1.78550566040443,1.,1.16747166312303));
#25640=CARTESIAN_POINT('Ctrl Pts',(1.78245795881009,-1.,1.16191881298499));
#25641=CARTESIAN_POINT('Ctrl Pts',(1.78245795881009,1.,1.16191881298499));
#25642=CARTESIAN_POINT('Ctrl Pts',(1.77938085564275,-1.,1.15639547194698));
#25643=CARTESIAN_POINT('Ctrl Pts',(1.77938085564275,1.,1.15639547194698));
#25644=CARTESIAN_POINT('Ctrl Pts',(1.7762742255701,-1.,1.15090197841515));
#25645=CARTESIAN_POINT('Ctrl Pts',(1.7762742255701,1.,1.15090197841515));
#25646=CARTESIAN_POINT('Ctrl Pts',(1.77313777896194,-1.,1.1454385822692));
#25647=CARTESIAN_POINT('Ctrl Pts',(1.77313777896194,1.,1.1454385822692));
#25648=CARTESIAN_POINT('Ctrl Pts',(1.76997111386769,-1.,1.14000548336975));
#25649=CARTESIAN_POINT('Ctrl Pts',(1.76997111386769,1.,1.14000548336975));
#25650=CARTESIAN_POINT('Ctrl Pts',(1.76677384551862,-1.,1.1346029180462));
#25651=CARTESIAN_POINT('Ctrl Pts',(1.76677384551862,1.,1.1346029180462));
#25652=CARTESIAN_POINT('Ctrl Pts',(1.7635457196617,-1.,1.12923123555075));
#25653=CARTESIAN_POINT('Ctrl Pts',(1.7635457196617,1.,1.12923123555075));
#25654=CARTESIAN_POINT('Ctrl Pts',(1.76028671825096,-1.,1.12389096855086));
#25655=CARTESIAN_POINT('Ctrl Pts',(1.76028671825096,1.,1.12389096855086));
#25656=CARTESIAN_POINT('Ctrl Pts',(1.75699720772105,-1.,1.11858293216763));
#25657=CARTESIAN_POINT('Ctrl Pts',(1.75699720772105,1.,1.11858293216763));
#25658=CARTESIAN_POINT('Ctrl Pts',(1.7536777209463,-1.,1.11330807582551));
#25659=CARTESIAN_POINT('Ctrl Pts',(1.7536777209463,1.,1.11330807582551));
#25660=CARTESIAN_POINT('Ctrl Pts',(1.7503286607592,-1.,1.10806728183007));
#25661=CARTESIAN_POINT('Ctrl Pts',(1.7503286607592,1.,1.10806728183007));
#25662=CARTESIAN_POINT('Ctrl Pts',(1.74695004214923,-1.,1.10286118991143));
#25663=CARTESIAN_POINT('Ctrl Pts',(1.74695004214923,1.,1.10286118991143));
#25664=CARTESIAN_POINT('Ctrl Pts',(1.74354119236208,-1.,1.09768999241226));
#25665=CARTESIAN_POINT('Ctrl Pts',(1.74354119236208,1.,1.09768999241226));
#25666=CARTESIAN_POINT('Ctrl Pts',(1.74010053962247,-1.,1.09255329056493));
#25667=CARTESIAN_POINT('Ctrl Pts',(1.74010053962247,1.,1.09255329056493));
#25668=CARTESIAN_POINT('Ctrl Pts',(1.73662628326091,-1.,1.08745056285427));
#25669=CARTESIAN_POINT('Ctrl Pts',(1.73662628326091,1.,1.08745056285427));
#25670=CARTESIAN_POINT('Ctrl Pts',(1.73311705663407,-1.,1.08238162784749));
#25671=CARTESIAN_POINT('Ctrl Pts',(1.73311705663407,1.,1.08238162784749));
#25672=CARTESIAN_POINT('Ctrl Pts',(1.72957248977424,-1.,1.0773470373727));
#25673=CARTESIAN_POINT('Ctrl Pts',(1.72957248977424,1.,1.0773470373727));
#25674=CARTESIAN_POINT('Ctrl Pts',(1.72599406198488,-1.,1.07234866990252));
#25675=CARTESIAN_POINT('Ctrl Pts',(1.72599406198488,1.,1.07234866990252));
#25676=CARTESIAN_POINT('Ctrl Pts',(1.72238500928453,-1.,1.06738966975462));
#25677=CARTESIAN_POINT('Ctrl Pts',(1.72238500928453,1.,1.06738966975462));
#25678=CARTESIAN_POINT('Ctrl Pts',(1.71874858456904,-1.,1.06247324680647));
#25679=CARTESIAN_POINT('Ctrl Pts',(1.71874858456904,1.,1.06247324680647));
#25680=CARTESIAN_POINT('Ctrl Pts',(1.7150865442702,-1.,1.05760163192479));
#25681=CARTESIAN_POINT('Ctrl Pts',(1.7150865442702,1.,1.05760163192479));
#25682=CARTESIAN_POINT('Ctrl Pts',(1.71139783543989,-1.,1.05277517202855));
#25683=CARTESIAN_POINT('Ctrl Pts',(1.71139783543989,1.,1.05277517202855));
#25684=CARTESIAN_POINT('Ctrl Pts',(1.70767646263649,-1.,1.04799085404995));
#25685=CARTESIAN_POINT('Ctrl Pts',(1.70767646263649,1.,1.04799085404995));
#25686=CARTESIAN_POINT('Ctrl Pts',(1.70391338707982,-1.,1.04324363334554));
#25687=CARTESIAN_POINT('Ctrl Pts',(1.70391338707982,1.,1.04324363334554));
#25688=CARTESIAN_POINT('Ctrl Pts',(1.70010052930962,-1.,1.03852922490789));
#25689=CARTESIAN_POINT('Ctrl Pts',(1.70010052930962,1.,1.03852922490789));
#25690=CARTESIAN_POINT('Ctrl Pts',(1.69623414782771,-1.,1.03384646003588));
#25691=CARTESIAN_POINT('Ctrl Pts',(1.69623414782771,1.,1.03384646003588));
#25692=CARTESIAN_POINT('Ctrl Pts',(1.69231840863458,-1.,1.02919977579147));
#25693=CARTESIAN_POINT('Ctrl Pts',(1.69231840863458,1.,1.02919977579147));
#25694=CARTESIAN_POINT('Ctrl Pts',(1.68836910178447,-1.,1.02460180535255));
#25695=CARTESIAN_POINT('Ctrl Pts',(1.68836910178447,1.,1.02460180535255));
#25696=CARTESIAN_POINT('Ctrl Pts',(1.68440578021706,-1.,1.02006795074201));
#25697=CARTESIAN_POINT('Ctrl Pts',(1.68440578021706,1.,1.02006795074201));
#25698=CARTESIAN_POINT('Ctrl Pts',(1.68044289894798,-1.,1.01561026162773));
#25699=CARTESIAN_POINT('Ctrl Pts',(1.68044289894798,1.,1.01561026162773));
#25700=CARTESIAN_POINT('Ctrl Pts',(1.67648246776464,-1.,1.01123236493511));
#25701=CARTESIAN_POINT('Ctrl Pts',(1.67648246776464,1.,1.01123236493511));
#25702=CARTESIAN_POINT('Ctrl Pts',(1.67250335383293,-1.,1.00692206696414));
#25703=CARTESIAN_POINT('Ctrl Pts',(1.67250335383293,1.,1.00692206696414));
#25704=CARTESIAN_POINT('Ctrl Pts',(1.66846059277303,-1.,1.00265091003727));
#25705=CARTESIAN_POINT('Ctrl Pts',(1.66846059277303,1.,1.00265091003727));
#25706=CARTESIAN_POINT('Ctrl Pts',(1.66430758030376,-1.,0.998389654952758));
#25707=CARTESIAN_POINT('Ctrl Pts',(1.66430758030376,1.,0.998389654952758));
#25708=CARTESIAN_POINT('Ctrl Pts',(1.66001553809947,-1.,0.994121836661306));
#25709=CARTESIAN_POINT('Ctrl Pts',(1.66001553809947,1.,0.994121836661306));
#25710=CARTESIAN_POINT('Ctrl Pts',(1.65559044289699,-1.,0.989855627854165));
#25711=CARTESIAN_POINT('Ctrl Pts',(1.65559044289699,1.,0.989855627854165));
#25712=CARTESIAN_POINT('Ctrl Pts',(1.65110016612638,-1.,0.985642622920821));
#25713=CARTESIAN_POINT('Ctrl Pts',(1.65110016612638,1.,0.985642622920821));
#25714=CARTESIAN_POINT('Ctrl Pts',(1.64665139190656,-1.,0.981562530939489));
#25715=CARTESIAN_POINT('Ctrl Pts',(1.64665139190656,1.,0.981562530939489));
#25716=CARTESIAN_POINT('Ctrl Pts',(1.64233990826687,-1.,0.977689794119417));
#25717=CARTESIAN_POINT('Ctrl Pts',(1.64233990826687,1.,0.977689794119417));
#25718=CARTESIAN_POINT('Ctrl Pts',(1.63820952658144,-1.,0.974066058287419));
#25719=CARTESIAN_POINT('Ctrl Pts',(1.63820952658144,1.,0.974066058287419));
#25720=CARTESIAN_POINT('Ctrl Pts',(1.63420665729798,-1.,0.970669715997509));
#25721=CARTESIAN_POINT('Ctrl Pts',(1.63420665729798,1.,0.970669715997509));
#25722=CARTESIAN_POINT('Ctrl Pts',(1.63013849959461,-1.,0.967387853230345));
#25723=CARTESIAN_POINT('Ctrl Pts',(1.63013849959461,1.,0.967387853230345));
#25724=CARTESIAN_POINT('Ctrl Pts',(1.62571930670187,-1.,0.964046107040536));
#25725=CARTESIAN_POINT('Ctrl Pts',(1.62571930670187,1.,0.964046107040536));
#25726=CARTESIAN_POINT('Ctrl Pts',(1.62061638140221,-1.,0.960438326101729));
#25727=CARTESIAN_POINT('Ctrl Pts',(1.62061638140221,1.,0.960438326101729));
#25728=CARTESIAN_POINT('Ctrl Pts',(1.61449324337085,-1.,0.956354422920671));
#25729=CARTESIAN_POINT('Ctrl Pts',(1.61449324337085,1.,0.956354422920671));
#25730=CARTESIAN_POINT('Ctrl Pts',(1.60706069896936,-1.,0.951613284356035));
#25731=CARTESIAN_POINT('Ctrl Pts',(1.60706069896936,1.,0.951613284356035));
#25732=CARTESIAN_POINT('Ctrl Pts',(1.59810042043673,-1.,0.946078063315257));
#25733=CARTESIAN_POINT('Ctrl Pts',(1.59810042043673,1.,0.946078063315257));
#25734=CARTESIAN_POINT('Ctrl Pts',(1.58744937487176,-1.,0.939646377893399));
#25735=CARTESIAN_POINT('Ctrl Pts',(1.58744937487176,1.,0.939646377893399));
#25736=CARTESIAN_POINT('Ctrl Pts',(1.57499388382243,-1.,0.932246680108685));
#25737=CARTESIAN_POINT('Ctrl Pts',(1.57499388382243,1.,0.932246680108685));
#25738=CARTESIAN_POINT('Ctrl Pts',(1.56065988578893,-1.,0.923832188944341));
#25739=CARTESIAN_POINT('Ctrl Pts',(1.56065988578893,1.,0.923832188944341));
#25740=CARTESIAN_POINT('Ctrl Pts',(1.54440491149498,-1.,0.914375919026456));
#25741=CARTESIAN_POINT('Ctrl Pts',(1.54440491149498,1.,0.914375919026456));
#25742=CARTESIAN_POINT('Ctrl Pts',(1.52984849887993,-1.,0.905967409625651));
#25743=CARTESIAN_POINT('Ctrl Pts',(1.52984849887993,1.,0.905967409625651));
#25744=CARTESIAN_POINT('Ctrl Pts',(1.51805569590094,-1.,0.899185047483511));
#25745=CARTESIAN_POINT('Ctrl Pts',(1.51805569590094,1.,0.899185047483511));
#25746=CARTESIAN_POINT('Ctrl Pts',(1.50980486806688,-1.,0.894452006964544));
#25747=CARTESIAN_POINT('Ctrl Pts',(1.50980486806688,1.,0.894452006964544));
#25748=CARTESIAN_POINT('Ctrl Pts',(1.5055822144029,-1.,0.892032620296856));
#25749=CARTESIAN_POINT('Ctrl Pts',(1.5055822144029,1.,0.892032620296856));
#25750=CARTESIAN_POINT('',(1.81978687191668,1.,1.23627494547115));
#25751=CARTESIAN_POINT('Ctrl Pts',(1.81978687191668,1.,1.23627494547115));
#25752=CARTESIAN_POINT('Ctrl Pts',(1.81925017193666,1.,1.23509651170476));
#25753=CARTESIAN_POINT('Ctrl Pts',(1.81817389921279,1.,1.2327422452705));
#25754=CARTESIAN_POINT('Ctrl Pts',(1.8165508718364,1.,1.2292186489137));
#25755=CARTESIAN_POINT('Ctrl Pts',(1.81436959210434,1.,1.2245361330495));
#25756=CARTESIAN_POINT('Ctrl Pts',(1.81161420806656,1.,1.21870906103557));
#25757=CARTESIAN_POINT('Ctrl Pts',(1.80882996917129,1.,1.21290815708314));
#25758=CARTESIAN_POINT('Ctrl Pts',(1.80601678480707,1.,1.20713356605475));
#25759=CARTESIAN_POINT('Ctrl Pts',(1.80317454838603,1.,1.20138548938974));
#25760=CARTESIAN_POINT('Ctrl Pts',(1.80030314369879,1.,1.19566418930242));
#25761=CARTESIAN_POINT('Ctrl Pts',(1.79740245923478,1.,1.18996997934445));
#25762=CARTESIAN_POINT('Ctrl Pts',(1.79447240321515,1.,1.18430321697432));
#25763=CARTESIAN_POINT('Ctrl Pts',(1.79151291552689,1.,1.17866429440809));
#25764=CARTESIAN_POINT('Ctrl Pts',(1.78852398877616,1.,1.17305363177328));
#25765=CARTESIAN_POINT('Ctrl Pts',(1.78550566040443,1.,1.16747166312303));
#25766=CARTESIAN_POINT('Ctrl Pts',(1.78245795881009,1.,1.16191881298499));
#25767=CARTESIAN_POINT('Ctrl Pts',(1.77938085564275,1.,1.15639547194698));
#25768=CARTESIAN_POINT('Ctrl Pts',(1.7762742255701,1.,1.15090197841515));
#25769=CARTESIAN_POINT('Ctrl Pts',(1.77313777896194,1.,1.1454385822692));
#25770=CARTESIAN_POINT('Ctrl Pts',(1.76997111386769,1.,1.14000548336975));
#25771=CARTESIAN_POINT('Ctrl Pts',(1.76677384551862,1.,1.1346029180462));
#25772=CARTESIAN_POINT('Ctrl Pts',(1.7635457196617,1.,1.12923123555075));
#25773=CARTESIAN_POINT('Ctrl Pts',(1.76028671825096,1.,1.12389096855086));
#25774=CARTESIAN_POINT('Ctrl Pts',(1.75699720772105,1.,1.11858293216763));
#25775=CARTESIAN_POINT('Ctrl Pts',(1.7536777209463,1.,1.11330807582551));
#25776=CARTESIAN_POINT('Ctrl Pts',(1.7503286607592,1.,1.10806728183007));
#25777=CARTESIAN_POINT('Ctrl Pts',(1.74695004214923,1.,1.10286118991143));
#25778=CARTESIAN_POINT('Ctrl Pts',(1.74354119236208,1.,1.09768999241226));
#25779=CARTESIAN_POINT('Ctrl Pts',(1.74010053962247,1.,1.09255329056493));
#25780=CARTESIAN_POINT('Ctrl Pts',(1.73662628326091,1.,1.08745056285427));
#25781=CARTESIAN_POINT('Ctrl Pts',(1.73311705663407,1.,1.08238162784749));
#25782=CARTESIAN_POINT('Ctrl Pts',(1.72957248977424,1.,1.0773470373727));
#25783=CARTESIAN_POINT('Ctrl Pts',(1.72599406198488,1.,1.07234866990252));
#25784=CARTESIAN_POINT('Ctrl Pts',(1.72238500928453,1.,1.06738966975462));
#25785=CARTESIAN_POINT('Ctrl Pts',(1.71874858456904,1.,1.06247324680647));
#25786=CARTESIAN_POINT('Ctrl Pts',(1.7150865442702,1.,1.05760163192479));
#25787=CARTESIAN_POINT('Ctrl Pts',(1.71139783543989,1.,1.05277517202855));
#25788=CARTESIAN_POINT('Ctrl Pts',(1.70767646263649,1.,1.04799085404995));
#25789=CARTESIAN_POINT('Ctrl Pts',(1.70391338707982,1.,1.04324363334554));
#25790=CARTESIAN_POINT('Ctrl Pts',(1.70010052930962,1.,1.03852922490789));
#25791=CARTESIAN_POINT('Ctrl Pts',(1.69623414782771,1.,1.03384646003588));
#25792=CARTESIAN_POINT('Ctrl Pts',(1.69231840863458,1.,1.02919977579147));
#25793=CARTESIAN_POINT('Ctrl Pts',(1.68836910178447,1.,1.02460180535255));
#25794=CARTESIAN_POINT('Ctrl Pts',(1.68440578021706,1.,1.02006795074201));
#25795=CARTESIAN_POINT('Ctrl Pts',(1.68044289894798,1.,1.01561026162773));
#25796=CARTESIAN_POINT('Ctrl Pts',(1.67648246776464,1.,1.01123236493511));
#25797=CARTESIAN_POINT('Ctrl Pts',(1.67250335383293,1.,1.00692206696414));
#25798=CARTESIAN_POINT('Ctrl Pts',(1.66846059277303,1.,1.00265091003727));
#25799=CARTESIAN_POINT('Ctrl Pts',(1.66430758030376,1.,0.998389654952758));
#25800=CARTESIAN_POINT('Ctrl Pts',(1.66001553809947,1.,0.994121836661306));
#25801=CARTESIAN_POINT('Ctrl Pts',(1.65559044289699,1.,0.989855627854165));
#25802=CARTESIAN_POINT('Ctrl Pts',(1.65110016612638,1.,0.985642622920821));
#25803=CARTESIAN_POINT('Ctrl Pts',(1.64665139190656,1.,0.981562530939489));
#25804=CARTESIAN_POINT('Ctrl Pts',(1.64233990826687,1.,0.977689794119417));
#25805=CARTESIAN_POINT('Ctrl Pts',(1.63820952658144,1.,0.974066058287419));
#25806=CARTESIAN_POINT('Ctrl Pts',(1.63420665729798,1.,0.970669715997509));
#25807=CARTESIAN_POINT('Ctrl Pts',(1.63013849959461,1.,0.967387853230345));
#25808=CARTESIAN_POINT('Ctrl Pts',(1.62571930670187,1.,0.964046107040536));
#25809=CARTESIAN_POINT('Ctrl Pts',(1.62061638140221,1.,0.960438326101729));
#25810=CARTESIAN_POINT('Ctrl Pts',(1.61449324337085,1.,0.956354422920671));
#25811=CARTESIAN_POINT('Ctrl Pts',(1.60706069896936,1.,0.951613284356035));
#25812=CARTESIAN_POINT('Ctrl Pts',(1.59810042043673,1.,0.946078063315257));
#25813=CARTESIAN_POINT('Ctrl Pts',(1.58744937487176,1.,0.939646377893399));
#25814=CARTESIAN_POINT('Ctrl Pts',(1.57499388382243,1.,0.932246680108685));
#25815=CARTESIAN_POINT('Ctrl Pts',(1.56065988578893,1.,0.923832188944341));
#25816=CARTESIAN_POINT('Ctrl Pts',(1.54440491149498,1.,0.914375919026456));
#25817=CARTESIAN_POINT('Ctrl Pts',(1.52984849887993,1.,0.905967409625651));
#25818=CARTESIAN_POINT('Ctrl Pts',(1.51805569590094,1.,0.899185047483511));
#25819=CARTESIAN_POINT('Ctrl Pts',(1.50980486806688,1.,0.894452006964544));
#25820=CARTESIAN_POINT('Ctrl Pts',(1.5055822144029,1.,0.892032620296856));
#25821=CARTESIAN_POINT('',(1.81978687191668,0.,1.23627494547115));
#25822=CARTESIAN_POINT('Origin',(1.73811241238545,0.,1.34869019493419));
#25823=CARTESIAN_POINT('',(1.73811241238545,1.,1.34869019493419));
#25824=CARTESIAN_POINT('',(1.81978687191668,1.,1.23627494547115));
#25825=CARTESIAN_POINT('',(1.73811241238545,0.,1.34869019493419));
#25826=CARTESIAN_POINT('Ctrl Pts',(1.31362392696032,-1.,1.15624053661742));
#25827=CARTESIAN_POINT('Ctrl Pts',(1.31362392696032,1.,1.15624053661742));
#25828=CARTESIAN_POINT('Ctrl Pts',(1.31722977216397,-1.,1.15950888730809));
#25829=CARTESIAN_POINT('Ctrl Pts',(1.31722977216397,1.,1.15950888730809));
#25830=CARTESIAN_POINT('Ctrl Pts',(1.32428080721772,-1.,1.16589330093588));
#25831=CARTESIAN_POINT('Ctrl Pts',(1.32428080721772,1.,1.16589330093588));
#25832=CARTESIAN_POINT('Ctrl Pts',(1.33437539347008,-1.,1.17501305789857));
#25833=CARTESIAN_POINT('Ctrl Pts',(1.33437539347008,1.,1.17501305789857));
#25834=CARTESIAN_POINT('Ctrl Pts',(1.34687054001093,-1.,1.18625865667441));
#25835=CARTESIAN_POINT('Ctrl Pts',(1.34687054001093,1.,1.18625865667441));
#25836=CARTESIAN_POINT('Ctrl Pts',(1.36088705043885,-1.,1.1987959077932));
#25837=CARTESIAN_POINT('Ctrl Pts',(1.36088705043885,1.,1.1987959077932));
#25838=CARTESIAN_POINT('Ctrl Pts',(1.37331915607905,-1.,1.20982812925645));
#25839=CARTESIAN_POINT('Ctrl Pts',(1.37331915607905,1.,1.20982812925645));
#25840=CARTESIAN_POINT('Ctrl Pts',(1.38420564527715,-1.,1.21938737280852));
#25841=CARTESIAN_POINT('Ctrl Pts',(1.38420564527715,1.,1.21938737280852));
#25842=CARTESIAN_POINT('Ctrl Pts',(1.39361389568796,-1.,1.22752961899387));
#25843=CARTESIAN_POINT('Ctrl Pts',(1.39361389568796,1.,1.22752961899387));
#25844=CARTESIAN_POINT('Ctrl Pts',(1.40164708206106,-1.,1.23434087290423));
#25845=CARTESIAN_POINT('Ctrl Pts',(1.40164708206106,1.,1.23434087290423));
#25846=CARTESIAN_POINT('Ctrl Pts',(1.40845295531283,-1.,1.23994455029534));
#25847=CARTESIAN_POINT('Ctrl Pts',(1.40845295531283,1.,1.23994455029534));
#25848=CARTESIAN_POINT('Ctrl Pts',(1.41422913175179,-1.,1.24450600513056));
#25849=CARTESIAN_POINT('Ctrl Pts',(1.41422913175179,1.,1.24450600513056));
#25850=CARTESIAN_POINT('Ctrl Pts',(1.41923722596025,-1.,1.24824430986571));
#25851=CARTESIAN_POINT('Ctrl Pts',(1.41923722596025,1.,1.24824430986571));
#25852=CARTESIAN_POINT('Ctrl Pts',(1.42378102115575,-1.,1.2514145557001));
#25853=CARTESIAN_POINT('Ctrl Pts',(1.42378102115575,1.,1.2514145557001));
#25854=CARTESIAN_POINT('Ctrl Pts',(1.42815938799387,-1.,1.25426945222639));
#25855=CARTESIAN_POINT('Ctrl Pts',(1.42815938799387,1.,1.25426945222639));
#25856=CARTESIAN_POINT('Ctrl Pts',(1.43262645609691,-1.,1.25702687965755));
#25857=CARTESIAN_POINT('Ctrl Pts',(1.43262645609691,1.,1.25702687965755));
#25858=CARTESIAN_POINT('Ctrl Pts',(1.43734919180847,-1.,1.25983531012005));
#25859=CARTESIAN_POINT('Ctrl Pts',(1.43734919180847,1.,1.25983531012005));
#25860=CARTESIAN_POINT('Ctrl Pts',(1.44236470511303,-1.,1.26273903323859));
#25861=CARTESIAN_POINT('Ctrl Pts',(1.44236470511303,1.,1.26273903323859));
#25862=CARTESIAN_POINT('Ctrl Pts',(1.44761985001662,-1.,1.26570925118868));
#25863=CARTESIAN_POINT('Ctrl Pts',(1.44761985001662,1.,1.26570925118868));
#25864=CARTESIAN_POINT('Ctrl Pts',(1.45301422764247,-1.,1.2686778680489));
#25865=CARTESIAN_POINT('Ctrl Pts',(1.45301422764247,1.,1.2686778680489));
#25866=CARTESIAN_POINT('Ctrl Pts',(1.45843906294697,-1.,1.27156805265289));
#25867=CARTESIAN_POINT('Ctrl Pts',(1.45843906294697,1.,1.27156805265289));
#25868=CARTESIAN_POINT('Ctrl Pts',(1.46382431332476,-1.,1.27433119897822));
#25869=CARTESIAN_POINT('Ctrl Pts',(1.46382431332476,1.,1.27433119897822));
#25870=CARTESIAN_POINT('Ctrl Pts',(1.46916035917133,-1.,1.2769641483109));
#25871=CARTESIAN_POINT('Ctrl Pts',(1.46916035917133,1.,1.2769641483109));
#25872=CARTESIAN_POINT('Ctrl Pts',(1.4744717526707,-1.,1.2794891824849));
#25873=CARTESIAN_POINT('Ctrl Pts',(1.4744717526707,1.,1.2794891824849));
#25874=CARTESIAN_POINT('Ctrl Pts',(1.47980070347095,-1.,1.28194158939517));
#25875=CARTESIAN_POINT('Ctrl Pts',(1.47980070347095,1.,1.28194158939517));
#25876=CARTESIAN_POINT('Ctrl Pts',(1.4851881711891,-1.,1.28435533880201));
#25877=CARTESIAN_POINT('Ctrl Pts',(1.4851881711891,1.,1.28435533880201));
#25878=CARTESIAN_POINT('Ctrl Pts',(1.4906522831278,-1.,1.2867467611644));
#25879=CARTESIAN_POINT('Ctrl Pts',(1.4906522831278,1.,1.2867467611644));
#25880=CARTESIAN_POINT('Ctrl Pts',(1.49618896881754,-1.,1.28911506584254));
#25881=CARTESIAN_POINT('Ctrl Pts',(1.49618896881754,1.,1.28911506584254));
#25882=CARTESIAN_POINT('Ctrl Pts',(1.50178230149776,-1.,1.29145022885181));
#25883=CARTESIAN_POINT('Ctrl Pts',(1.50178230149776,1.,1.29145022885181));
#25884=CARTESIAN_POINT('Ctrl Pts',(1.50741159078365,-1.,1.29373841372842));
#25885=CARTESIAN_POINT('Ctrl Pts',(1.50741159078365,1.,1.29373841372842));
#25886=CARTESIAN_POINT('Ctrl Pts',(1.51305994241402,-1.,1.29596850710509));
#25887=CARTESIAN_POINT('Ctrl Pts',(1.51305994241402,1.,1.29596850710509));
#25888=CARTESIAN_POINT('Ctrl Pts',(1.51872184912724,-1.,1.29813791800747));
#25889=CARTESIAN_POINT('Ctrl Pts',(1.51872184912724,1.,1.29813791800747));
#25890=CARTESIAN_POINT('Ctrl Pts',(1.52439957861062,-1.,1.30024984366328));
#25891=CARTESIAN_POINT('Ctrl Pts',(1.52439957861062,1.,1.30024984366328));
#25892=CARTESIAN_POINT('Ctrl Pts',(1.53009970283891,-1.,1.30231064395568));
#25893=CARTESIAN_POINT('Ctrl Pts',(1.53009970283891,1.,1.30231064395568));
#25894=CARTESIAN_POINT('Ctrl Pts',(1.53582981268977,-1.,1.30432735639489));
#25895=CARTESIAN_POINT('Ctrl Pts',(1.53582981268977,1.,1.30432735639489));
#25896=CARTESIAN_POINT('Ctrl Pts',(1.54159462645432,-1.,1.30630475189556));
#25897=CARTESIAN_POINT('Ctrl Pts',(1.54159462645432,1.,1.30630475189556));
#25898=CARTESIAN_POINT('Ctrl Pts',(1.54739413957185,-1.,1.30824393907473));
#25899=CARTESIAN_POINT('Ctrl Pts',(1.54739413957185,1.,1.30824393907473));
#25900=CARTESIAN_POINT('Ctrl Pts',(1.55322568759481,-1.,1.31014393684222));
#25901=CARTESIAN_POINT('Ctrl Pts',(1.55322568759481,1.,1.31014393684222));
#25902=CARTESIAN_POINT('Ctrl Pts',(1.55908521254821,-1.,1.31200264341696));
#25903=CARTESIAN_POINT('Ctrl Pts',(1.55908521254821,1.,1.31200264341696));
#25904=CARTESIAN_POINT('Ctrl Pts',(1.56496872402353,-1.,1.31381795281002));
#25905=CARTESIAN_POINT('Ctrl Pts',(1.56496872402353,1.,1.31381795281002));
#25906=CARTESIAN_POINT('Ctrl Pts',(1.57087397835723,-1.,1.31558903860016));
#25907=CARTESIAN_POINT('Ctrl Pts',(1.57087397835723,1.,1.31558903860016));
#25908=CARTESIAN_POINT('Ctrl Pts',(1.5768005650559,-1.,1.31731642317187));
#25909=CARTESIAN_POINT('Ctrl Pts',(1.5768005650559,1.,1.31731642317187));
#25910=CARTESIAN_POINT('Ctrl Pts',(1.58274907898834,-1.,1.31900135021432));
#25911=CARTESIAN_POINT('Ctrl Pts',(1.58274907898834,1.,1.31900135021432));
#25912=CARTESIAN_POINT('Ctrl Pts',(1.58872057258245,-1.,1.32064537110892));
#25913=CARTESIAN_POINT('Ctrl Pts',(1.58872057258245,1.,1.32064537110892));
#25914=CARTESIAN_POINT('Ctrl Pts',(1.59471591079403,-1.,1.32224985747682));
#25915=CARTESIAN_POINT('Ctrl Pts',(1.59471591079403,1.,1.32224985747682));
#25916=CARTESIAN_POINT('Ctrl Pts',(1.60073511858687,-1.,1.32381550858256));
#25917=CARTESIAN_POINT('Ctrl Pts',(1.60073511858687,1.,1.32381550858256));
#25918=CARTESIAN_POINT('Ctrl Pts',(1.60677758290954,-1.,1.32534250785782));
#25919=CARTESIAN_POINT('Ctrl Pts',(1.60677758290954,1.,1.32534250785782));
#25920=CARTESIAN_POINT('Ctrl Pts',(1.6128423401575,-1.,1.32683074483356));
#25921=CARTESIAN_POINT('Ctrl Pts',(1.6128423401575,1.,1.32683074483356));
#25922=CARTESIAN_POINT('Ctrl Pts',(1.61892832270724,-1.,1.32828000610449));
#25923=CARTESIAN_POINT('Ctrl Pts',(1.61892832270724,1.,1.32828000610449));
#25924=CARTESIAN_POINT('Ctrl Pts',(1.62503464209797,-1.,1.3296901950568));
#25925=CARTESIAN_POINT('Ctrl Pts',(1.62503464209797,1.,1.3296901950568));
#25926=CARTESIAN_POINT('Ctrl Pts',(1.63116079730923,-1.,1.33106149345645));
#25927=CARTESIAN_POINT('Ctrl Pts',(1.63116079730923,1.,1.33106149345645));
#25928=CARTESIAN_POINT('Ctrl Pts',(1.63730653475089,-1.,1.33239425103724));
#25929=CARTESIAN_POINT('Ctrl Pts',(1.63730653475089,1.,1.33239425103724));
#25930=CARTESIAN_POINT('Ctrl Pts',(1.6434717485603,-1.,1.33368890676572));
#25931=CARTESIAN_POINT('Ctrl Pts',(1.6434717485603,1.,1.33368890676572));
#25932=CARTESIAN_POINT('Ctrl Pts',(1.6496563728683,-1.,1.33494590467993));
#25933=CARTESIAN_POINT('Ctrl Pts',(1.6496563728683,1.,1.33494590467993));
#25934=CARTESIAN_POINT('Ctrl Pts',(1.65586025952593,-1.,1.33616559745172));
#25935=CARTESIAN_POINT('Ctrl Pts',(1.65586025952593,1.,1.33616559745172));
#25936=CARTESIAN_POINT('Ctrl Pts',(1.66208312541983,-1.,1.33734820885262));
#25937=CARTESIAN_POINT('Ctrl Pts',(1.66208312541983,1.,1.33734820885262));
#25938=CARTESIAN_POINT('Ctrl Pts',(1.66832460783989,-1.,1.33849388654388));
#25939=CARTESIAN_POINT('Ctrl Pts',(1.66832460783989,1.,1.33849388654388));
#25940=CARTESIAN_POINT('Ctrl Pts',(1.67458429426086,-1.,1.3396027347034));
#25941=CARTESIAN_POINT('Ctrl Pts',(1.67458429426086,1.,1.3396027347034));
#25942=CARTESIAN_POINT('Ctrl Pts',(1.68086176030362,-1.,1.34067485185203));
#25943=CARTESIAN_POINT('Ctrl Pts',(1.68086176030362,1.,1.34067485185203));
#25944=CARTESIAN_POINT('Ctrl Pts',(1.68715660868764,-1.,1.341710374848));
#25945=CARTESIAN_POINT('Ctrl Pts',(1.68715660868764,1.,1.341710374848));
#25946=CARTESIAN_POINT('Ctrl Pts',(1.6934684849687,-1.,1.34270948206319));
#25947=CARTESIAN_POINT('Ctrl Pts',(1.6934684849687,1.,1.34270948206319));
#25948=CARTESIAN_POINT('Ctrl Pts',(1.69979707754427,-1.,1.34367237124483));
#25949=CARTESIAN_POINT('Ctrl Pts',(1.69979707754427,1.,1.34367237124483));
#25950=CARTESIAN_POINT('Ctrl Pts',(1.70614212266738,-1.,1.34459924533831));
#25951=CARTESIAN_POINT('Ctrl Pts',(1.70614212266738,1.,1.34459924533831));
#25952=CARTESIAN_POINT('Ctrl Pts',(1.71250340686822,-1.,1.34549029589416));
#25953=CARTESIAN_POINT('Ctrl Pts',(1.71250340686822,1.,1.34549029589416));
#25954=CARTESIAN_POINT('Ctrl Pts',(1.7188807715049,-1.,1.34634568653227));
#25955=CARTESIAN_POINT('Ctrl Pts',(1.7188807715049,1.,1.34634568653227));
#25956=CARTESIAN_POINT('Ctrl Pts',(1.72527410680674,-1.,1.34716554819527));
#25957=CARTESIAN_POINT('Ctrl Pts',(1.72527410680674,1.,1.34716554819527));
#25958=CARTESIAN_POINT('Ctrl Pts',(1.7304014965394,-1.,1.34779309152035));
#25959=CARTESIAN_POINT('Ctrl Pts',(1.7304014965394,1.,1.34779309152035));
#25960=CARTESIAN_POINT('Ctrl Pts',(1.73425417885907,-1.,1.34824783112887));
#25961=CARTESIAN_POINT('Ctrl Pts',(1.73425417885907,1.,1.34824783112887));
#25962=CARTESIAN_POINT('Ctrl Pts',(1.73682580585691,-1.,1.34854391898045));
#25963=CARTESIAN_POINT('Ctrl Pts',(1.73682580585691,1.,1.34854391898045));
#25964=CARTESIAN_POINT('Ctrl Pts',(1.73811241238545,-1.,1.34869019493419));
#25965=CARTESIAN_POINT('Ctrl Pts',(1.73811241238545,1.,1.34869019493419));
#25966=CARTESIAN_POINT('',(1.31362392696032,1.,1.15624053661742));
#25967=CARTESIAN_POINT('Ctrl Pts',(1.31362392696032,1.,1.15624053661742));
#25968=CARTESIAN_POINT('Ctrl Pts',(1.31722977216397,1.,1.15950888730809));
#25969=CARTESIAN_POINT('Ctrl Pts',(1.32428080721772,1.,1.16589330093588));
#25970=CARTESIAN_POINT('Ctrl Pts',(1.33437539347008,1.,1.17501305789857));
#25971=CARTESIAN_POINT('Ctrl Pts',(1.34687054001093,1.,1.18625865667441));
#25972=CARTESIAN_POINT('Ctrl Pts',(1.36088705043885,1.,1.1987959077932));
#25973=CARTESIAN_POINT('Ctrl Pts',(1.37331915607905,1.,1.20982812925645));
#25974=CARTESIAN_POINT('Ctrl Pts',(1.38420564527715,1.,1.21938737280852));
#25975=CARTESIAN_POINT('Ctrl Pts',(1.39361389568796,1.,1.22752961899387));
#25976=CARTESIAN_POINT('Ctrl Pts',(1.40164708206106,1.,1.23434087290423));
#25977=CARTESIAN_POINT('Ctrl Pts',(1.40845295531283,1.,1.23994455029534));
#25978=CARTESIAN_POINT('Ctrl Pts',(1.41422913175179,1.,1.24450600513056));
#25979=CARTESIAN_POINT('Ctrl Pts',(1.41923722596025,1.,1.24824430986571));
#25980=CARTESIAN_POINT('Ctrl Pts',(1.42378102115575,1.,1.2514145557001));
#25981=CARTESIAN_POINT('Ctrl Pts',(1.42815938799387,1.,1.25426945222639));
#25982=CARTESIAN_POINT('Ctrl Pts',(1.43262645609691,1.,1.25702687965755));
#25983=CARTESIAN_POINT('Ctrl Pts',(1.43734919180847,1.,1.25983531012005));
#25984=CARTESIAN_POINT('Ctrl Pts',(1.44236470511303,1.,1.26273903323859));
#25985=CARTESIAN_POINT('Ctrl Pts',(1.44761985001662,1.,1.26570925118868));
#25986=CARTESIAN_POINT('Ctrl Pts',(1.45301422764247,1.,1.2686778680489));
#25987=CARTESIAN_POINT('Ctrl Pts',(1.45843906294697,1.,1.27156805265289));
#25988=CARTESIAN_POINT('Ctrl Pts',(1.46382431332476,1.,1.27433119897822));
#25989=CARTESIAN_POINT('Ctrl Pts',(1.46916035917133,1.,1.2769641483109));
#25990=CARTESIAN_POINT('Ctrl Pts',(1.4744717526707,1.,1.2794891824849));
#25991=CARTESIAN_POINT('Ctrl Pts',(1.47980070347095,1.,1.28194158939517));
#25992=CARTESIAN_POINT('Ctrl Pts',(1.4851881711891,1.,1.28435533880201));
#25993=CARTESIAN_POINT('Ctrl Pts',(1.4906522831278,1.,1.2867467611644));
#25994=CARTESIAN_POINT('Ctrl Pts',(1.49618896881754,1.,1.28911506584254));
#25995=CARTESIAN_POINT('Ctrl Pts',(1.50178230149776,1.,1.29145022885181));
#25996=CARTESIAN_POINT('Ctrl Pts',(1.50741159078365,1.,1.29373841372842));
#25997=CARTESIAN_POINT('Ctrl Pts',(1.51305994241402,1.,1.29596850710509));
#25998=CARTESIAN_POINT('Ctrl Pts',(1.51872184912724,1.,1.29813791800747));
#25999=CARTESIAN_POINT('Ctrl Pts',(1.52439957861062,1.,1.30024984366328));
#26000=CARTESIAN_POINT('Ctrl Pts',(1.53009970283891,1.,1.30231064395568));
#26001=CARTESIAN_POINT('Ctrl Pts',(1.53582981268977,1.,1.30432735639489));
#26002=CARTESIAN_POINT('Ctrl Pts',(1.54159462645432,1.,1.30630475189556));
#26003=CARTESIAN_POINT('Ctrl Pts',(1.54739413957185,1.,1.30824393907473));
#26004=CARTESIAN_POINT('Ctrl Pts',(1.55322568759481,1.,1.31014393684222));
#26005=CARTESIAN_POINT('Ctrl Pts',(1.55908521254821,1.,1.31200264341696));
#26006=CARTESIAN_POINT('Ctrl Pts',(1.56496872402353,1.,1.31381795281002));
#26007=CARTESIAN_POINT('Ctrl Pts',(1.57087397835723,1.,1.31558903860016));
#26008=CARTESIAN_POINT('Ctrl Pts',(1.5768005650559,1.,1.31731642317187));
#26009=CARTESIAN_POINT('Ctrl Pts',(1.58274907898834,1.,1.31900135021432));
#26010=CARTESIAN_POINT('Ctrl Pts',(1.58872057258245,1.,1.32064537110892));
#26011=CARTESIAN_POINT('Ctrl Pts',(1.59471591079403,1.,1.32224985747682));
#26012=CARTESIAN_POINT('Ctrl Pts',(1.60073511858687,1.,1.32381550858256));
#26013=CARTESIAN_POINT('Ctrl Pts',(1.60677758290954,1.,1.32534250785782));
#26014=CARTESIAN_POINT('Ctrl Pts',(1.6128423401575,1.,1.32683074483356));
#26015=CARTESIAN_POINT('Ctrl Pts',(1.61892832270724,1.,1.32828000610449));
#26016=CARTESIAN_POINT('Ctrl Pts',(1.62503464209797,1.,1.3296901950568));
#26017=CARTESIAN_POINT('Ctrl Pts',(1.63116079730923,1.,1.33106149345645));
#26018=CARTESIAN_POINT('Ctrl Pts',(1.63730653475089,1.,1.33239425103724));
#26019=CARTESIAN_POINT('Ctrl Pts',(1.6434717485603,1.,1.33368890676572));
#26020=CARTESIAN_POINT('Ctrl Pts',(1.6496563728683,1.,1.33494590467993));
#26021=CARTESIAN_POINT('Ctrl Pts',(1.65586025952593,1.,1.33616559745172));
#26022=CARTESIAN_POINT('Ctrl Pts',(1.66208312541983,1.,1.33734820885262));
#26023=CARTESIAN_POINT('Ctrl Pts',(1.66832460783989,1.,1.33849388654388));
#26024=CARTESIAN_POINT('Ctrl Pts',(1.67458429426086,1.,1.3396027347034));
#26025=CARTESIAN_POINT('Ctrl Pts',(1.68086176030362,1.,1.34067485185203));
#26026=CARTESIAN_POINT('Ctrl Pts',(1.68715660868764,1.,1.341710374848));
#26027=CARTESIAN_POINT('Ctrl Pts',(1.6934684849687,1.,1.34270948206319));
#26028=CARTESIAN_POINT('Ctrl Pts',(1.69979707754427,1.,1.34367237124483));
#26029=CARTESIAN_POINT('Ctrl Pts',(1.70614212266738,1.,1.34459924533831));
#26030=CARTESIAN_POINT('Ctrl Pts',(1.71250340686822,1.,1.34549029589416));
#26031=CARTESIAN_POINT('Ctrl Pts',(1.7188807715049,1.,1.34634568653227));
#26032=CARTESIAN_POINT('Ctrl Pts',(1.72527410680674,1.,1.34716554819527));
#26033=CARTESIAN_POINT('Ctrl Pts',(1.7304014965394,1.,1.34779309152035));
#26034=CARTESIAN_POINT('Ctrl Pts',(1.73425417885907,1.,1.34824783112887));
#26035=CARTESIAN_POINT('Ctrl Pts',(1.73682580585691,1.,1.34854391898045));
#26036=CARTESIAN_POINT('Ctrl Pts',(1.73811241238545,1.,1.34869019493419));
#26037=CARTESIAN_POINT('',(1.31362392696032,0.,1.15624053661742));
#26038=CARTESIAN_POINT('Origin',(0.,0.,0.));
#26039=CARTESIAN_POINT('',(1.15624053661742,1.,1.31362392696033));
#26040=CARTESIAN_POINT('Origin',(0.,1.,0.));
#26041=CARTESIAN_POINT('',(1.15624053661742,0.,1.31362392696032));
#26042=CARTESIAN_POINT('Ctrl Pts',(1.34869019493419,-1.,1.73811241238545));
#26043=CARTESIAN_POINT('Ctrl Pts',(1.34869019493419,1.,1.73811241238545));
#26044=CARTESIAN_POINT('Ctrl Pts',(1.34854391898145,-1.,1.73682580585819));
#26045=CARTESIAN_POINT('Ctrl Pts',(1.34854391898145,1.,1.73682580585819));
#26046=CARTESIAN_POINT('Ctrl Pts',(1.34824783113158,-1.,1.73425417886255));
#26047=CARTESIAN_POINT('Ctrl Pts',(1.34824783113158,1.,1.73425417886255));
#26048=CARTESIAN_POINT('Ctrl Pts',(1.3477930915247,-1.,1.73040149654497));
#26049=CARTESIAN_POINT('Ctrl Pts',(1.3477930915247,1.,1.73040149654497));
#26050=CARTESIAN_POINT('Ctrl Pts',(1.34716554820013,-1.,1.72527410681298));
#26051=CARTESIAN_POINT('Ctrl Pts',(1.34716554820013,1.,1.72527410681298));
#26052=CARTESIAN_POINT('Ctrl Pts',(1.34634568653586,-1.,1.7188807715095));
#26053=CARTESIAN_POINT('Ctrl Pts',(1.34634568653586,1.,1.7188807715095));
#26054=CARTESIAN_POINT('Ctrl Pts',(1.34549029589563,-1.,1.71250340687011));
#26055=CARTESIAN_POINT('Ctrl Pts',(1.34549029589563,1.,1.71250340687011));
#26056=CARTESIAN_POINT('Ctrl Pts',(1.34459924533783,-1.,1.70614212266676));
#26057=CARTESIAN_POINT('Ctrl Pts',(1.34459924533783,1.,1.70614212266676));
#26058=CARTESIAN_POINT('Ctrl Pts',(1.34367237124322,-1.,1.69979707754221));
#26059=CARTESIAN_POINT('Ctrl Pts',(1.34367237124322,1.,1.69979707754221));
#26060=CARTESIAN_POINT('Ctrl Pts',(1.34270948206139,-1.,1.6934684849664));
#26061=CARTESIAN_POINT('Ctrl Pts',(1.34270948206139,1.,1.6934684849664));
#26062=CARTESIAN_POINT('Ctrl Pts',(1.34171037484673,-1.,1.68715660868602));
#26063=CARTESIAN_POINT('Ctrl Pts',(1.34171037484673,1.,1.68715660868602));
#26064=CARTESIAN_POINT('Ctrl Pts',(1.3406748518516,-1.,1.68086176030308));
#26065=CARTESIAN_POINT('Ctrl Pts',(1.3406748518516,1.,1.68086176030308));
#26066=CARTESIAN_POINT('Ctrl Pts',(1.33960273470372,-1.,1.67458429426126));
#26067=CARTESIAN_POINT('Ctrl Pts',(1.33960273470372,1.,1.67458429426126));
#26068=CARTESIAN_POINT('Ctrl Pts',(1.33849388654458,-1.,1.66832460784078));
#26069=CARTESIAN_POINT('Ctrl Pts',(1.33849388654458,1.,1.66832460784078));
#26070=CARTESIAN_POINT('Ctrl Pts',(1.33734820885331,-1.,1.66208312542073));
#26071=CARTESIAN_POINT('Ctrl Pts',(1.33734820885331,1.,1.66208312542073));
#26072=CARTESIAN_POINT('Ctrl Pts',(1.33616559745217,-1.,1.65586025952651));
#26073=CARTESIAN_POINT('Ctrl Pts',(1.33616559745217,1.,1.65586025952651));
#26074=CARTESIAN_POINT('Ctrl Pts',(1.33494590468003,-1.,1.64965637286843));
#26075=CARTESIAN_POINT('Ctrl Pts',(1.33494590468003,1.,1.64965637286843));
#26076=CARTESIAN_POINT('Ctrl Pts',(1.33368890676554,-1.,1.64347174856007));
#26077=CARTESIAN_POINT('Ctrl Pts',(1.33368890676554,1.,1.64347174856007));
#26078=CARTESIAN_POINT('Ctrl Pts',(1.33239425103694,-1.,1.6373065347505));
#26079=CARTESIAN_POINT('Ctrl Pts',(1.33239425103694,1.,1.6373065347505));
#26080=CARTESIAN_POINT('Ctrl Pts',(1.33106149345618,-1.,1.63116079730887));
#26081=CARTESIAN_POINT('Ctrl Pts',(1.33106149345618,1.,1.63116079730887));
#26082=CARTESIAN_POINT('Ctrl Pts',(1.32969019505665,-1.,1.62503464209777));
#26083=CARTESIAN_POINT('Ctrl Pts',(1.32969019505665,1.,1.62503464209777));
#26084=CARTESIAN_POINT('Ctrl Pts',(1.32828000610448,-1.,1.61892832270723));
#26085=CARTESIAN_POINT('Ctrl Pts',(1.32828000610448,1.,1.61892832270723));
#26086=CARTESIAN_POINT('Ctrl Pts',(1.32683074483365,-1.,1.61284234015762));
#26087=CARTESIAN_POINT('Ctrl Pts',(1.32683074483365,1.,1.61284234015762));
#26088=CARTESIAN_POINT('Ctrl Pts',(1.32534250785794,-1.,1.6067775829097));
#26089=CARTESIAN_POINT('Ctrl Pts',(1.32534250785794,1.,1.6067775829097));
#26090=CARTESIAN_POINT('Ctrl Pts',(1.32381550858266,-1.,1.600735118587));
#26091=CARTESIAN_POINT('Ctrl Pts',(1.32381550858266,1.,1.600735118587));
#26092=CARTESIAN_POINT('Ctrl Pts',(1.32224985747686,-1.,1.59471591079408));
#26093=CARTESIAN_POINT('Ctrl Pts',(1.32224985747686,1.,1.59471591079408));
#26094=CARTESIAN_POINT('Ctrl Pts',(1.32064537110891,-1.,1.58872057258244));
#26095=CARTESIAN_POINT('Ctrl Pts',(1.32064537110891,1.,1.58872057258244));
#26096=CARTESIAN_POINT('Ctrl Pts',(1.31900135021428,-1.,1.58274907898829));
#26097=CARTESIAN_POINT('Ctrl Pts',(1.31900135021428,1.,1.58274907898829));
#26098=CARTESIAN_POINT('Ctrl Pts',(1.31731642317183,-1.,1.57680056505585));
#26099=CARTESIAN_POINT('Ctrl Pts',(1.31731642317183,1.,1.57680056505585));
#26100=CARTESIAN_POINT('Ctrl Pts',(1.31558903860015,-1.,1.57087397835721));
#26101=CARTESIAN_POINT('Ctrl Pts',(1.31558903860015,1.,1.57087397835721));
#26102=CARTESIAN_POINT('Ctrl Pts',(1.31381795281002,-1.,1.56496872402352));
#26103=CARTESIAN_POINT('Ctrl Pts',(1.31381795281002,1.,1.56496872402352));
#26104=CARTESIAN_POINT('Ctrl Pts',(1.31200264341696,-1.,1.55908521254822));
#26105=CARTESIAN_POINT('Ctrl Pts',(1.31200264341696,1.,1.55908521254822));
#26106=CARTESIAN_POINT('Ctrl Pts',(1.31014393684221,-1.,1.55322568759481));
#26107=CARTESIAN_POINT('Ctrl Pts',(1.31014393684221,1.,1.55322568759481));
#26108=CARTESIAN_POINT('Ctrl Pts',(1.30824393907471,-1.,1.54739413957183));
#26109=CARTESIAN_POINT('Ctrl Pts',(1.30824393907471,1.,1.54739413957183));
#26110=CARTESIAN_POINT('Ctrl Pts',(1.30630475189553,-1.,1.54159462645428));
#26111=CARTESIAN_POINT('Ctrl Pts',(1.30630475189553,1.,1.54159462645428));
#26112=CARTESIAN_POINT('Ctrl Pts',(1.30432735639487,-1.,1.53582981268976));
#26113=CARTESIAN_POINT('Ctrl Pts',(1.30432735639487,1.,1.53582981268976));
#26114=CARTESIAN_POINT('Ctrl Pts',(1.3023106439557,-1.,1.53009970283893));
#26115=CARTESIAN_POINT('Ctrl Pts',(1.3023106439557,1.,1.53009970283893));
#26116=CARTESIAN_POINT('Ctrl Pts',(1.30024984366334,-1.,1.5243995786107));
#26117=CARTESIAN_POINT('Ctrl Pts',(1.30024984366334,1.,1.5243995786107));
#26118=CARTESIAN_POINT('Ctrl Pts',(1.29813791800757,-1.,1.51872184912735));
#26119=CARTESIAN_POINT('Ctrl Pts',(1.29813791800757,1.,1.51872184912735));
#26120=CARTESIAN_POINT('Ctrl Pts',(1.29596850710518,-1.,1.51305994241412));
#26121=CARTESIAN_POINT('Ctrl Pts',(1.29596850710518,1.,1.51305994241412));
#26122=CARTESIAN_POINT('Ctrl Pts',(1.29373841372843,-1.,1.50741159078367));
#26123=CARTESIAN_POINT('Ctrl Pts',(1.29373841372843,1.,1.50741159078367));
#26124=CARTESIAN_POINT('Ctrl Pts',(1.29145022885171,-1.,1.50178230149764));
#26125=CARTESIAN_POINT('Ctrl Pts',(1.29145022885171,1.,1.50178230149764));
#26126=CARTESIAN_POINT('Ctrl Pts',(1.28911506584232,-1.,1.49618896881729));
#26127=CARTESIAN_POINT('Ctrl Pts',(1.28911506584232,1.,1.49618896881729));
#26128=CARTESIAN_POINT('Ctrl Pts',(1.28674676116415,-1.,1.4906522831275));
#26129=CARTESIAN_POINT('Ctrl Pts',(1.28674676116415,1.,1.4906522831275));
#26130=CARTESIAN_POINT('Ctrl Pts',(1.28435533880184,-1.,1.48518817118891));
#26131=CARTESIAN_POINT('Ctrl Pts',(1.28435533880184,1.,1.48518817118891));
#26132=CARTESIAN_POINT('Ctrl Pts',(1.28194158939522,-1.,1.47980070347102));
#26133=CARTESIAN_POINT('Ctrl Pts',(1.28194158939522,1.,1.47980070347102));
#26134=CARTESIAN_POINT('Ctrl Pts',(1.27948918248524,-1.,1.4744717526711));
#26135=CARTESIAN_POINT('Ctrl Pts',(1.27948918248524,1.,1.4744717526711));
#26136=CARTESIAN_POINT('Ctrl Pts',(1.27696414831144,-1.,1.46916035917197));
#26137=CARTESIAN_POINT('Ctrl Pts',(1.27696414831144,1.,1.46916035917197));
#26138=CARTESIAN_POINT('Ctrl Pts',(1.27433119897877,-1.,1.4638243133254));
#26139=CARTESIAN_POINT('Ctrl Pts',(1.27433119897877,1.,1.4638243133254));
#26140=CARTESIAN_POINT('Ctrl Pts',(1.27156805265312,-1.,1.45843906294725));
#26141=CARTESIAN_POINT('Ctrl Pts',(1.27156805265312,1.,1.45843906294725));
#26142=CARTESIAN_POINT('Ctrl Pts',(1.26867786804854,-1.,1.45301422764205));
#26143=CARTESIAN_POINT('Ctrl Pts',(1.26867786804854,1.,1.45301422764205));
#26144=CARTESIAN_POINT('Ctrl Pts',(1.26570925118767,-1.,1.44761985001544));
#26145=CARTESIAN_POINT('Ctrl Pts',(1.26570925118767,1.,1.44761985001544));
#26146=CARTESIAN_POINT('Ctrl Pts',(1.26273903323723,-1.,1.44236470511145));
#26147=CARTESIAN_POINT('Ctrl Pts',(1.26273903323723,1.,1.44236470511145));
#26148=CARTESIAN_POINT('Ctrl Pts',(1.25983531011894,-1.,1.43734919180719));
#26149=CARTESIAN_POINT('Ctrl Pts',(1.25983531011894,1.,1.43734919180719));
#26150=CARTESIAN_POINT('Ctrl Pts',(1.25702687965744,-1.,1.43262645609679));
#26151=CARTESIAN_POINT('Ctrl Pts',(1.25702687965744,1.,1.43262645609679));
#26152=CARTESIAN_POINT('Ctrl Pts',(1.25426945222783,-1.,1.42815938799555));
#26153=CARTESIAN_POINT('Ctrl Pts',(1.25426945222783,1.,1.42815938799555));
#26154=CARTESIAN_POINT('Ctrl Pts',(1.25141455570299,-1.,1.42378102115911));
#26155=CARTESIAN_POINT('Ctrl Pts',(1.25141455570299,1.,1.42378102115911));
#26156=CARTESIAN_POINT('Ctrl Pts',(1.24824430986911,-1.,1.41923722596421));
#26157=CARTESIAN_POINT('Ctrl Pts',(1.24824430986911,1.,1.41923722596421));
#26158=CARTESIAN_POINT('Ctrl Pts',(1.24450600513278,-1.,1.41422913175437));
#26159=CARTESIAN_POINT('Ctrl Pts',(1.24450600513278,1.,1.41422913175437));
#26160=CARTESIAN_POINT('Ctrl Pts',(1.23994455029421,-1.,1.40845295531151));
#26161=CARTESIAN_POINT('Ctrl Pts',(1.23994455029421,1.,1.40845295531151));
#26162=CARTESIAN_POINT('Ctrl Pts',(1.23434087289768,-1.,1.40164708205345));
#26163=CARTESIAN_POINT('Ctrl Pts',(1.23434087289768,1.,1.40164708205345));
#26164=CARTESIAN_POINT('Ctrl Pts',(1.22752961898063,-1.,1.39361389567257));
#26165=CARTESIAN_POINT('Ctrl Pts',(1.22752961898063,1.,1.39361389567257));
#26166=CARTESIAN_POINT('Ctrl Pts',(1.21938737278853,-1.,1.38420564525391));
#26167=CARTESIAN_POINT('Ctrl Pts',(1.21938737278853,1.,1.38420564525391));
#26168=CARTESIAN_POINT('Ctrl Pts',(1.20982812923113,-1.,1.37331915604962));
#26169=CARTESIAN_POINT('Ctrl Pts',(1.20982812923113,1.,1.37331915604962));
#26170=CARTESIAN_POINT('Ctrl Pts',(1.1987959077656,-1.,1.36088705040677));
#26171=CARTESIAN_POINT('Ctrl Pts',(1.1987959077656,1.,1.36088705040677));
#26172=CARTESIAN_POINT('Ctrl Pts',(1.18625865664915,-1.,1.34687053998157));
#26173=CARTESIAN_POINT('Ctrl Pts',(1.18625865664915,1.,1.34687053998157));
#26174=CARTESIAN_POINT('Ctrl Pts',(1.17501305787994,-1.,1.33437539344842));
#26175=CARTESIAN_POINT('Ctrl Pts',(1.17501305787994,1.,1.33437539344842));
#26176=CARTESIAN_POINT('Ctrl Pts',(1.16589330092532,-1.,1.32428080720544));
#26177=CARTESIAN_POINT('Ctrl Pts',(1.16589330092532,1.,1.32428080720544));
#26178=CARTESIAN_POINT('Ctrl Pts',(1.15950888730433,-1.,1.3172297721596));
#26179=CARTESIAN_POINT('Ctrl Pts',(1.15950888730433,1.,1.3172297721596));
#26180=CARTESIAN_POINT('Ctrl Pts',(1.15624053661742,-1.,1.31362392696033));
#26181=CARTESIAN_POINT('Ctrl Pts',(1.15624053661742,1.,1.31362392696033));
#26182=CARTESIAN_POINT('',(1.34869019493419,1.,1.73811241238545));
#26183=CARTESIAN_POINT('Ctrl Pts',(1.34869019493419,1.,1.73811241238545));
#26184=CARTESIAN_POINT('Ctrl Pts',(1.34854391898145,1.,1.73682580585819));
#26185=CARTESIAN_POINT('Ctrl Pts',(1.34824783113158,1.,1.73425417886255));
#26186=CARTESIAN_POINT('Ctrl Pts',(1.3477930915247,1.,1.73040149654497));
#26187=CARTESIAN_POINT('Ctrl Pts',(1.34716554820013,1.,1.72527410681298));
#26188=CARTESIAN_POINT('Ctrl Pts',(1.34634568653586,1.,1.7188807715095));
#26189=CARTESIAN_POINT('Ctrl Pts',(1.34549029589563,1.,1.71250340687011));
#26190=CARTESIAN_POINT('Ctrl Pts',(1.34459924533783,1.,1.70614212266676));
#26191=CARTESIAN_POINT('Ctrl Pts',(1.34367237124322,1.,1.69979707754221));
#26192=CARTESIAN_POINT('Ctrl Pts',(1.34270948206139,1.,1.6934684849664));
#26193=CARTESIAN_POINT('Ctrl Pts',(1.34171037484673,1.,1.68715660868602));
#26194=CARTESIAN_POINT('Ctrl Pts',(1.3406748518516,1.,1.68086176030308));
#26195=CARTESIAN_POINT('Ctrl Pts',(1.33960273470372,1.,1.67458429426126));
#26196=CARTESIAN_POINT('Ctrl Pts',(1.33849388654458,1.,1.66832460784078));
#26197=CARTESIAN_POINT('Ctrl Pts',(1.33734820885331,1.,1.66208312542073));
#26198=CARTESIAN_POINT('Ctrl Pts',(1.33616559745217,1.,1.65586025952651));
#26199=CARTESIAN_POINT('Ctrl Pts',(1.33494590468003,1.,1.64965637286843));
#26200=CARTESIAN_POINT('Ctrl Pts',(1.33368890676554,1.,1.64347174856007));
#26201=CARTESIAN_POINT('Ctrl Pts',(1.33239425103694,1.,1.6373065347505));
#26202=CARTESIAN_POINT('Ctrl Pts',(1.33106149345618,1.,1.63116079730887));
#26203=CARTESIAN_POINT('Ctrl Pts',(1.32969019505665,1.,1.62503464209777));
#26204=CARTESIAN_POINT('Ctrl Pts',(1.32828000610448,1.,1.61892832270723));
#26205=CARTESIAN_POINT('Ctrl Pts',(1.32683074483365,1.,1.61284234015762));
#26206=CARTESIAN_POINT('Ctrl Pts',(1.32534250785794,1.,1.6067775829097));
#26207=CARTESIAN_POINT('Ctrl Pts',(1.32381550858266,1.,1.600735118587));
#26208=CARTESIAN_POINT('Ctrl Pts',(1.32224985747686,1.,1.59471591079408));
#26209=CARTESIAN_POINT('Ctrl Pts',(1.32064537110891,1.,1.58872057258244));
#26210=CARTESIAN_POINT('Ctrl Pts',(1.31900135021428,1.,1.58274907898829));
#26211=CARTESIAN_POINT('Ctrl Pts',(1.31731642317183,1.,1.57680056505585));
#26212=CARTESIAN_POINT('Ctrl Pts',(1.31558903860015,1.,1.57087397835721));
#26213=CARTESIAN_POINT('Ctrl Pts',(1.31381795281002,1.,1.56496872402352));
#26214=CARTESIAN_POINT('Ctrl Pts',(1.31200264341696,1.,1.55908521254822));
#26215=CARTESIAN_POINT('Ctrl Pts',(1.31014393684221,1.,1.55322568759481));
#26216=CARTESIAN_POINT('Ctrl Pts',(1.30824393907471,1.,1.54739413957183));
#26217=CARTESIAN_POINT('Ctrl Pts',(1.30630475189553,1.,1.54159462645428));
#26218=CARTESIAN_POINT('Ctrl Pts',(1.30432735639487,1.,1.53582981268976));
#26219=CARTESIAN_POINT('Ctrl Pts',(1.3023106439557,1.,1.53009970283893));
#26220=CARTESIAN_POINT('Ctrl Pts',(1.30024984366334,1.,1.5243995786107));
#26221=CARTESIAN_POINT('Ctrl Pts',(1.29813791800757,1.,1.51872184912735));
#26222=CARTESIAN_POINT('Ctrl Pts',(1.29596850710518,1.,1.51305994241412));
#26223=CARTESIAN_POINT('Ctrl Pts',(1.29373841372843,1.,1.50741159078367));
#26224=CARTESIAN_POINT('Ctrl Pts',(1.29145022885171,1.,1.50178230149764));
#26225=CARTESIAN_POINT('Ctrl Pts',(1.28911506584232,1.,1.49618896881729));
#26226=CARTESIAN_POINT('Ctrl Pts',(1.28674676116415,1.,1.4906522831275));
#26227=CARTESIAN_POINT('Ctrl Pts',(1.28435533880184,1.,1.48518817118891));
#26228=CARTESIAN_POINT('Ctrl Pts',(1.28194158939522,1.,1.47980070347102));
#26229=CARTESIAN_POINT('Ctrl Pts',(1.27948918248524,1.,1.4744717526711));
#26230=CARTESIAN_POINT('Ctrl Pts',(1.27696414831144,1.,1.46916035917197));
#26231=CARTESIAN_POINT('Ctrl Pts',(1.27433119897877,1.,1.4638243133254));
#26232=CARTESIAN_POINT('Ctrl Pts',(1.27156805265312,1.,1.45843906294725));
#26233=CARTESIAN_POINT('Ctrl Pts',(1.26867786804854,1.,1.45301422764205));
#26234=CARTESIAN_POINT('Ctrl Pts',(1.26570925118767,1.,1.44761985001544));
#26235=CARTESIAN_POINT('Ctrl Pts',(1.26273903323723,1.,1.44236470511145));
#26236=CARTESIAN_POINT('Ctrl Pts',(1.25983531011894,1.,1.43734919180719));
#26237=CARTESIAN_POINT('Ctrl Pts',(1.25702687965744,1.,1.43262645609679));
#26238=CARTESIAN_POINT('Ctrl Pts',(1.25426945222783,1.,1.42815938799555));
#26239=CARTESIAN_POINT('Ctrl Pts',(1.25141455570299,1.,1.42378102115911));
#26240=CARTESIAN_POINT('Ctrl Pts',(1.24824430986911,1.,1.41923722596421));
#26241=CARTESIAN_POINT('Ctrl Pts',(1.24450600513278,1.,1.41422913175437));
#26242=CARTESIAN_POINT('Ctrl Pts',(1.23994455029421,1.,1.40845295531151));
#26243=CARTESIAN_POINT('Ctrl Pts',(1.23434087289768,1.,1.40164708205345));
#26244=CARTESIAN_POINT('Ctrl Pts',(1.22752961898063,1.,1.39361389567257));
#26245=CARTESIAN_POINT('Ctrl Pts',(1.21938737278853,1.,1.38420564525391));
#26246=CARTESIAN_POINT('Ctrl Pts',(1.20982812923113,1.,1.37331915604962));
#26247=CARTESIAN_POINT('Ctrl Pts',(1.1987959077656,1.,1.36088705040677));
#26248=CARTESIAN_POINT('Ctrl Pts',(1.18625865664915,1.,1.34687053998157));
#26249=CARTESIAN_POINT('Ctrl Pts',(1.17501305787994,1.,1.33437539344842));
#26250=CARTESIAN_POINT('Ctrl Pts',(1.16589330092532,1.,1.32428080720544));
#26251=CARTESIAN_POINT('Ctrl Pts',(1.15950888730433,1.,1.3172297721596));
#26252=CARTESIAN_POINT('Ctrl Pts',(1.15624053661742,1.,1.31362392696033));
#26253=CARTESIAN_POINT('',(1.34869019493419,0.,1.73811241238545));
#26254=CARTESIAN_POINT('Origin',(1.23627494547115,0.,1.81978687191668));
#26255=CARTESIAN_POINT('',(1.23627494547115,1.,1.81978687191668));
#26256=CARTESIAN_POINT('',(1.34869019493419,1.,1.73811241238545));
#26257=CARTESIAN_POINT('',(1.23627494547115,0.,1.81978687191668));
#26258=CARTESIAN_POINT('Ctrl Pts',(0.892032620296855,-1.,1.5055822144029));
#26259=CARTESIAN_POINT('Ctrl Pts',(0.892032620296855,1.,1.5055822144029));
#26260=CARTESIAN_POINT('Ctrl Pts',(0.894452006967538,-1.,1.50980486807181));
#26261=CARTESIAN_POINT('Ctrl Pts',(0.894452006967538,1.,1.50980486807181));
#26262=CARTESIAN_POINT('Ctrl Pts',(0.89918504749193,-1.,1.51805569591479));
#26263=CARTESIAN_POINT('Ctrl Pts',(0.89918504749193,1.,1.51805569591479));
#26264=CARTESIAN_POINT('Ctrl Pts',(0.905967409640498,-1.,1.52984849890434));
#26265=CARTESIAN_POINT('Ctrl Pts',(0.905967409640498,1.,1.52984849890434));
#26266=CARTESIAN_POINT('Ctrl Pts',(0.914375919046579,-1.,1.54440491152808));
#26267=CARTESIAN_POINT('Ctrl Pts',(0.914375919046579,1.,1.54440491152808));
#26268=CARTESIAN_POINT('Ctrl Pts',(0.923832188966322,-1.,1.56065988582509));
#26269=CARTESIAN_POINT('Ctrl Pts',(0.923832188966322,1.,1.56065988582509));
#26270=CARTESIAN_POINT('Ctrl Pts',(0.932246680128848,-1.,1.57499388385561));
#26271=CARTESIAN_POINT('Ctrl Pts',(0.932246680128848,1.,1.57499388385561));
#26272=CARTESIAN_POINT('Ctrl Pts',(0.939646377909319,-1.,1.58744937489796));
#26273=CARTESIAN_POINT('Ctrl Pts',(0.939646377909319,1.,1.58744937489796));
#26274=CARTESIAN_POINT('Ctrl Pts',(0.946078063325795,-1.,1.59810042045408));
#26275=CARTESIAN_POINT('Ctrl Pts',(0.946078063325795,1.,1.59810042045408));
#26276=CARTESIAN_POINT('Ctrl Pts',(0.951613284361247,-1.,1.60706069897794));
#26277=CARTESIAN_POINT('Ctrl Pts',(0.951613284361247,1.,1.60706069897794));
#26278=CARTESIAN_POINT('Ctrl Pts',(0.956354422921572,-1.,1.61449324337233));
#26279=CARTESIAN_POINT('Ctrl Pts',(0.956354422921572,1.,1.61449324337233));
#26280=CARTESIAN_POINT('Ctrl Pts',(0.960438326099958,-1.,1.62061638139929));
#26281=CARTESIAN_POINT('Ctrl Pts',(0.960438326099958,1.,1.62061638139929));
#26282=CARTESIAN_POINT('Ctrl Pts',(0.964046107037821,-1.,1.6257193066974));
#26283=CARTESIAN_POINT('Ctrl Pts',(0.964046107037821,1.,1.6257193066974));
#26284=CARTESIAN_POINT('Ctrl Pts',(0.967387853228041,-1.,1.63013849959083));
#26285=CARTESIAN_POINT('Ctrl Pts',(0.967387853228041,1.,1.63013849959083));
#26286=CARTESIAN_POINT('Ctrl Pts',(0.970669715996356,-1.,1.63420665729609));
#26287=CARTESIAN_POINT('Ctrl Pts',(0.970669715996356,1.,1.63420665729609));
#26288=CARTESIAN_POINT('Ctrl Pts',(0.974066058287501,-1.,1.63820952658157));
#26289=CARTESIAN_POINT('Ctrl Pts',(0.974066058287501,1.,1.63820952658157));
#26290=CARTESIAN_POINT('Ctrl Pts',(0.977689794120296,-1.,1.64233990826831));
#26291=CARTESIAN_POINT('Ctrl Pts',(0.977689794120296,1.,1.64233990826831));
#26292=CARTESIAN_POINT('Ctrl Pts',(0.981562530940574,-1.,1.64665139190834));
#26293=CARTESIAN_POINT('Ctrl Pts',(0.981562530940574,1.,1.64665139190834));
#26294=CARTESIAN_POINT('Ctrl Pts',(0.985642622921626,-1.,1.6511001661277));
#26295=CARTESIAN_POINT('Ctrl Pts',(0.985642622921626,1.,1.6511001661277));
#26296=CARTESIAN_POINT('Ctrl Pts',(0.98985562785445,-1.,1.65559044289746));
#26297=CARTESIAN_POINT('Ctrl Pts',(0.98985562785445,1.,1.65559044289746));
#26298=CARTESIAN_POINT('Ctrl Pts',(0.994121836661115,-1.,1.66001553809916));
#26299=CARTESIAN_POINT('Ctrl Pts',(0.994121836661115,1.,1.66001553809916));
#26300=CARTESIAN_POINT('Ctrl Pts',(0.998389654952317,-1.,1.66430758030304));
#26301=CARTESIAN_POINT('Ctrl Pts',(0.998389654952317,1.,1.66430758030304));
#26302=CARTESIAN_POINT('Ctrl Pts',(1.00265091003682,-1.,1.66846059277231));
#26303=CARTESIAN_POINT('Ctrl Pts',(1.00265091003682,1.,1.66846059277231));
#26304=CARTESIAN_POINT('Ctrl Pts',(1.00692206696387,-1.,1.67250335383248));
#26305=CARTESIAN_POINT('Ctrl Pts',(1.00692206696387,1.,1.67250335383248));
#26306=CARTESIAN_POINT('Ctrl Pts',(1.01123236493507,-1.,1.67648246776457));
#26307=CARTESIAN_POINT('Ctrl Pts',(1.01123236493507,1.,1.67648246776457));
#26308=CARTESIAN_POINT('Ctrl Pts',(1.01561026162786,-1.,1.6804428989482));
#26309=CARTESIAN_POINT('Ctrl Pts',(1.01561026162786,1.,1.6804428989482));
#26310=CARTESIAN_POINT('Ctrl Pts',(1.02006795074222,-1.,1.68440578021739));
#26311=CARTESIAN_POINT('Ctrl Pts',(1.02006795074222,1.,1.68440578021739));
#26312=CARTESIAN_POINT('Ctrl Pts',(1.02460180535272,-1.,1.68836910178475));
#26313=CARTESIAN_POINT('Ctrl Pts',(1.02460180535272,1.,1.68836910178475));
#26314=CARTESIAN_POINT('Ctrl Pts',(1.02919977579155,-1.,1.69231840863471));
#26315=CARTESIAN_POINT('Ctrl Pts',(1.02919977579155,1.,1.69231840863471));
#26316=CARTESIAN_POINT('Ctrl Pts',(1.03384646003587,-1.,1.69623414782769));
#26317=CARTESIAN_POINT('Ctrl Pts',(1.03384646003587,1.,1.69623414782769));
#26318=CARTESIAN_POINT('Ctrl Pts',(1.03852922490782,-1.,1.70010052930951));
#26319=CARTESIAN_POINT('Ctrl Pts',(1.03852922490782,1.,1.70010052930951));
#26320=CARTESIAN_POINT('Ctrl Pts',(1.04324363334546,-1.,1.70391338707969));
#26321=CARTESIAN_POINT('Ctrl Pts',(1.04324363334546,1.,1.70391338707969));
#26322=CARTESIAN_POINT('Ctrl Pts',(1.0479908540499,-1.,1.70767646263641));
#26323=CARTESIAN_POINT('Ctrl Pts',(1.0479908540499,1.,1.70767646263641));
#26324=CARTESIAN_POINT('Ctrl Pts',(1.05277517202853,-1.,1.71139783543986));
#26325=CARTESIAN_POINT('Ctrl Pts',(1.05277517202853,1.,1.71139783543986));
#26326=CARTESIAN_POINT('Ctrl Pts',(1.05760163192481,-1.,1.71508654427022));
#26327=CARTESIAN_POINT('Ctrl Pts',(1.05760163192481,1.,1.71508654427022));
#26328=CARTESIAN_POINT('Ctrl Pts',(1.06247324680649,-1.,1.71874858456908));
#26329=CARTESIAN_POINT('Ctrl Pts',(1.06247324680649,1.,1.71874858456908));
#26330=CARTESIAN_POINT('Ctrl Pts',(1.06738966975463,-1.,1.72238500928456));
#26331=CARTESIAN_POINT('Ctrl Pts',(1.06738966975463,1.,1.72238500928456));
#26332=CARTESIAN_POINT('Ctrl Pts',(1.07234866990252,-1.,1.72599406198489));
#26333=CARTESIAN_POINT('Ctrl Pts',(1.07234866990252,1.,1.72599406198489));
#26334=CARTESIAN_POINT('Ctrl Pts',(1.0773470373727,-1.,1.72957248977424));
#26335=CARTESIAN_POINT('Ctrl Pts',(1.0773470373727,1.,1.72957248977424));
#26336=CARTESIAN_POINT('Ctrl Pts',(1.08238162784749,-1.,1.73311705663407));
#26337=CARTESIAN_POINT('Ctrl Pts',(1.08238162784749,1.,1.73311705663407));
#26338=CARTESIAN_POINT('Ctrl Pts',(1.08745056285429,-1.,1.73662628326093));
#26339=CARTESIAN_POINT('Ctrl Pts',(1.08745056285429,1.,1.73662628326093));
#26340=CARTESIAN_POINT('Ctrl Pts',(1.09255329056496,-1.,1.74010053962252));
#26341=CARTESIAN_POINT('Ctrl Pts',(1.09255329056496,1.,1.74010053962252));
#26342=CARTESIAN_POINT('Ctrl Pts',(1.09768999241229,-1.,1.74354119236212));
#26343=CARTESIAN_POINT('Ctrl Pts',(1.09768999241229,1.,1.74354119236212));
#26344=CARTESIAN_POINT('Ctrl Pts',(1.10286118991144,-1.,1.74695004214924));
#26345=CARTESIAN_POINT('Ctrl Pts',(1.10286118991144,1.,1.74695004214924));
#26346=CARTESIAN_POINT('Ctrl Pts',(1.10806728183003,-1.,1.75032866075914));
#26347=CARTESIAN_POINT('Ctrl Pts',(1.10806728183003,1.,1.75032866075914));
#26348=CARTESIAN_POINT('Ctrl Pts',(1.11330807582542,-1.,1.75367772094617));
#26349=CARTESIAN_POINT('Ctrl Pts',(1.11330807582542,1.,1.75367772094617));
#26350=CARTESIAN_POINT('Ctrl Pts',(1.11858293216752,-1.,1.75699720772089));
#26351=CARTESIAN_POINT('Ctrl Pts',(1.11858293216752,1.,1.75699720772089));
#26352=CARTESIAN_POINT('Ctrl Pts',(1.12389096855078,-1.,1.76028671825084));
#26353=CARTESIAN_POINT('Ctrl Pts',(1.12389096855078,1.,1.76028671825084));
#26354=CARTESIAN_POINT('Ctrl Pts',(1.12923123555076,-1.,1.76354571966171));
#26355=CARTESIAN_POINT('Ctrl Pts',(1.12923123555076,1.,1.76354571966171));
#26356=CARTESIAN_POINT('Ctrl Pts',(1.13460291804634,-1.,1.76677384551883));
#26357=CARTESIAN_POINT('Ctrl Pts',(1.13460291804634,1.,1.76677384551883));
#26358=CARTESIAN_POINT('Ctrl Pts',(1.14000548337,-1.,1.76997111386806));
#26359=CARTESIAN_POINT('Ctrl Pts',(1.14000548337,1.,1.76997111386806));
#26360=CARTESIAN_POINT('Ctrl Pts',(1.14543858226948,-1.,1.77313777896234));
#26361=CARTESIAN_POINT('Ctrl Pts',(1.14543858226948,1.,1.77313777896234));
#26362=CARTESIAN_POINT('Ctrl Pts',(1.15090197841531,-1.,1.77627422557034));
#26363=CARTESIAN_POINT('Ctrl Pts',(1.15090197841531,1.,1.77627422557034));
#26364=CARTESIAN_POINT('Ctrl Pts',(1.15639547194689,-1.,1.77938085564261));
#26365=CARTESIAN_POINT('Ctrl Pts',(1.15639547194689,1.,1.77938085564261));
#26366=CARTESIAN_POINT('Ctrl Pts',(1.16191881298458,-1.,1.78245795880949));
#26367=CARTESIAN_POINT('Ctrl Pts',(1.16191881298458,1.,1.78245795880949));
#26368=CARTESIAN_POINT('Ctrl Pts',(1.16747166312239,-1.,1.78550566040349));
#26369=CARTESIAN_POINT('Ctrl Pts',(1.16747166312239,1.,1.78550566040349));
#26370=CARTESIAN_POINT('Ctrl Pts',(1.17305363177265,-1.,1.78852398877523));
#26371=CARTESIAN_POINT('Ctrl Pts',(1.17305363177265,1.,1.78852398877523));
#26372=CARTESIAN_POINT('Ctrl Pts',(1.17866429440781,-1.,1.79151291552646));
#26373=CARTESIAN_POINT('Ctrl Pts',(1.17866429440781,1.,1.79151291552646));
#26374=CARTESIAN_POINT('Ctrl Pts',(1.18430321697471,-1.,1.79447240321572));
#26375=CARTESIAN_POINT('Ctrl Pts',(1.18430321697471,1.,1.79447240321572));
#26376=CARTESIAN_POINT('Ctrl Pts',(1.1899699793456,-1.,1.79740245923649));
#26377=CARTESIAN_POINT('Ctrl Pts',(1.1899699793456,1.,1.79740245923649));
#26378=CARTESIAN_POINT('Ctrl Pts',(1.19566418930405,-1.,1.80030314370121));
#26379=CARTESIAN_POINT('Ctrl Pts',(1.19566418930405,1.,1.80030314370121));
#26380=CARTESIAN_POINT('Ctrl Pts',(1.2013854893912,-1.,1.8031745483882));
#26381=CARTESIAN_POINT('Ctrl Pts',(1.2013854893912,1.,1.8031745483882));
#26382=CARTESIAN_POINT('Ctrl Pts',(1.20713356605519,-1.,1.80601678480772));
#26383=CARTESIAN_POINT('Ctrl Pts',(1.20713356605519,1.,1.80601678480772));
#26384=CARTESIAN_POINT('Ctrl Pts',(1.2129081570818,-1.,1.80882996916931));
#26385=CARTESIAN_POINT('Ctrl Pts',(1.2129081570818,1.,1.80882996916931));
#26386=CARTESIAN_POINT('Ctrl Pts',(1.2187090610323,-1.,1.81161420806172));
#26387=CARTESIAN_POINT('Ctrl Pts',(1.2187090610323,1.,1.81161420806172));
#26388=CARTESIAN_POINT('Ctrl Pts',(1.22453613304507,-1.,1.81436959209778));
#26389=CARTESIAN_POINT('Ctrl Pts',(1.22453613304507,1.,1.81436959209778));
#26390=CARTESIAN_POINT('Ctrl Pts',(1.22921864890975,-1.,1.81655087183054));
#26391=CARTESIAN_POINT('Ctrl Pts',(1.22921864890975,1.,1.81655087183054));
#26392=CARTESIAN_POINT('Ctrl Pts',(1.23274224526804,-1.,1.81817389920914));
#26393=CARTESIAN_POINT('Ctrl Pts',(1.23274224526804,1.,1.81817389920914));
#26394=CARTESIAN_POINT('Ctrl Pts',(1.23509651170384,-1.,1.81925017193531));
#26395=CARTESIAN_POINT('Ctrl Pts',(1.23509651170384,1.,1.81925017193531));
#26396=CARTESIAN_POINT('Ctrl Pts',(1.23627494547115,-1.,1.81978687191668));
#26397=CARTESIAN_POINT('Ctrl Pts',(1.23627494547115,1.,1.81978687191668));
#26398=CARTESIAN_POINT('',(0.892032620296855,1.,1.5055822144029));
#26399=CARTESIAN_POINT('Ctrl Pts',(0.892032620296855,1.,1.5055822144029));
#26400=CARTESIAN_POINT('Ctrl Pts',(0.894452006967538,1.,1.50980486807181));
#26401=CARTESIAN_POINT('Ctrl Pts',(0.89918504749193,1.,1.51805569591479));
#26402=CARTESIAN_POINT('Ctrl Pts',(0.905967409640498,1.,1.52984849890434));
#26403=CARTESIAN_POINT('Ctrl Pts',(0.914375919046579,1.,1.54440491152808));
#26404=CARTESIAN_POINT('Ctrl Pts',(0.923832188966322,1.,1.56065988582509));
#26405=CARTESIAN_POINT('Ctrl Pts',(0.932246680128848,1.,1.57499388385561));
#26406=CARTESIAN_POINT('Ctrl Pts',(0.939646377909319,1.,1.58744937489796));
#26407=CARTESIAN_POINT('Ctrl Pts',(0.946078063325795,1.,1.59810042045408));
#26408=CARTESIAN_POINT('Ctrl Pts',(0.951613284361247,1.,1.60706069897794));
#26409=CARTESIAN_POINT('Ctrl Pts',(0.956354422921572,1.,1.61449324337233));
#26410=CARTESIAN_POINT('Ctrl Pts',(0.960438326099958,1.,1.62061638139929));
#26411=CARTESIAN_POINT('Ctrl Pts',(0.964046107037821,1.,1.6257193066974));
#26412=CARTESIAN_POINT('Ctrl Pts',(0.967387853228041,1.,1.63013849959083));
#26413=CARTESIAN_POINT('Ctrl Pts',(0.970669715996356,1.,1.63420665729609));
#26414=CARTESIAN_POINT('Ctrl Pts',(0.974066058287501,1.,1.63820952658157));
#26415=CARTESIAN_POINT('Ctrl Pts',(0.977689794120296,1.,1.64233990826831));
#26416=CARTESIAN_POINT('Ctrl Pts',(0.981562530940574,1.,1.64665139190834));
#26417=CARTESIAN_POINT('Ctrl Pts',(0.985642622921626,1.,1.6511001661277));
#26418=CARTESIAN_POINT('Ctrl Pts',(0.98985562785445,1.,1.65559044289746));
#26419=CARTESIAN_POINT('Ctrl Pts',(0.994121836661115,1.,1.66001553809916));
#26420=CARTESIAN_POINT('Ctrl Pts',(0.998389654952317,1.,1.66430758030304));
#26421=CARTESIAN_POINT('Ctrl Pts',(1.00265091003682,1.,1.66846059277231));
#26422=CARTESIAN_POINT('Ctrl Pts',(1.00692206696387,1.,1.67250335383248));
#26423=CARTESIAN_POINT('Ctrl Pts',(1.01123236493507,1.,1.67648246776457));
#26424=CARTESIAN_POINT('Ctrl Pts',(1.01561026162786,1.,1.6804428989482));
#26425=CARTESIAN_POINT('Ctrl Pts',(1.02006795074222,1.,1.68440578021739));
#26426=CARTESIAN_POINT('Ctrl Pts',(1.02460180535272,1.,1.68836910178475));
#26427=CARTESIAN_POINT('Ctrl Pts',(1.02919977579155,1.,1.69231840863471));
#26428=CARTESIAN_POINT('Ctrl Pts',(1.03384646003587,1.,1.69623414782769));
#26429=CARTESIAN_POINT('Ctrl Pts',(1.03852922490782,1.,1.70010052930951));
#26430=CARTESIAN_POINT('Ctrl Pts',(1.04324363334546,1.,1.70391338707969));
#26431=CARTESIAN_POINT('Ctrl Pts',(1.0479908540499,1.,1.70767646263641));
#26432=CARTESIAN_POINT('Ctrl Pts',(1.05277517202853,1.,1.71139783543986));
#26433=CARTESIAN_POINT('Ctrl Pts',(1.05760163192481,1.,1.71508654427022));
#26434=CARTESIAN_POINT('Ctrl Pts',(1.06247324680649,1.,1.71874858456908));
#26435=CARTESIAN_POINT('Ctrl Pts',(1.06738966975463,1.,1.72238500928456));
#26436=CARTESIAN_POINT('Ctrl Pts',(1.07234866990252,1.,1.72599406198489));
#26437=CARTESIAN_POINT('Ctrl Pts',(1.0773470373727,1.,1.72957248977424));
#26438=CARTESIAN_POINT('Ctrl Pts',(1.08238162784749,1.,1.73311705663407));
#26439=CARTESIAN_POINT('Ctrl Pts',(1.08745056285429,1.,1.73662628326093));
#26440=CARTESIAN_POINT('Ctrl Pts',(1.09255329056496,1.,1.74010053962252));
#26441=CARTESIAN_POINT('Ctrl Pts',(1.09768999241229,1.,1.74354119236212));
#26442=CARTESIAN_POINT('Ctrl Pts',(1.10286118991144,1.,1.74695004214924));
#26443=CARTESIAN_POINT('Ctrl Pts',(1.10806728183003,1.,1.75032866075914));
#26444=CARTESIAN_POINT('Ctrl Pts',(1.11330807582542,1.,1.75367772094617));
#26445=CARTESIAN_POINT('Ctrl Pts',(1.11858293216752,1.,1.75699720772089));
#26446=CARTESIAN_POINT('Ctrl Pts',(1.12389096855078,1.,1.76028671825084));
#26447=CARTESIAN_POINT('Ctrl Pts',(1.12923123555076,1.,1.76354571966171));
#26448=CARTESIAN_POINT('Ctrl Pts',(1.13460291804634,1.,1.76677384551883));
#26449=CARTESIAN_POINT('Ctrl Pts',(1.14000548337,1.,1.76997111386806));
#26450=CARTESIAN_POINT('Ctrl Pts',(1.14543858226948,1.,1.77313777896234));
#26451=CARTESIAN_POINT('Ctrl Pts',(1.15090197841531,1.,1.77627422557034));
#26452=CARTESIAN_POINT('Ctrl Pts',(1.15639547194689,1.,1.77938085564261));
#26453=CARTESIAN_POINT('Ctrl Pts',(1.16191881298458,1.,1.78245795880949));
#26454=CARTESIAN_POINT('Ctrl Pts',(1.16747166312239,1.,1.78550566040349));
#26455=CARTESIAN_POINT('Ctrl Pts',(1.17305363177265,1.,1.78852398877523));
#26456=CARTESIAN_POINT('Ctrl Pts',(1.17866429440781,1.,1.79151291552646));
#26457=CARTESIAN_POINT('Ctrl Pts',(1.18430321697471,1.,1.79447240321572));
#26458=CARTESIAN_POINT('Ctrl Pts',(1.1899699793456,1.,1.79740245923649));
#26459=CARTESIAN_POINT('Ctrl Pts',(1.19566418930405,1.,1.80030314370121));
#26460=CARTESIAN_POINT('Ctrl Pts',(1.2013854893912,1.,1.8031745483882));
#26461=CARTESIAN_POINT('Ctrl Pts',(1.20713356605519,1.,1.80601678480772));
#26462=CARTESIAN_POINT('Ctrl Pts',(1.2129081570818,1.,1.80882996916931));
#26463=CARTESIAN_POINT('Ctrl Pts',(1.2187090610323,1.,1.81161420806172));
#26464=CARTESIAN_POINT('Ctrl Pts',(1.22453613304507,1.,1.81436959209778));
#26465=CARTESIAN_POINT('Ctrl Pts',(1.22921864890975,1.,1.81655087183054));
#26466=CARTESIAN_POINT('Ctrl Pts',(1.23274224526804,1.,1.81817389920914));
#26467=CARTESIAN_POINT('Ctrl Pts',(1.23509651170384,1.,1.81925017193531));
#26468=CARTESIAN_POINT('Ctrl Pts',(1.23627494547115,1.,1.81978687191668));
#26469=CARTESIAN_POINT('',(0.892032620296854,0.,1.5055822144029));
#26470=CARTESIAN_POINT('Origin',(0.,0.,0.));
#26471=CARTESIAN_POINT('',(0.693717979106305,1.,1.60662857109684));
#26472=CARTESIAN_POINT('Origin',(0.,1.,0.));
#26473=CARTESIAN_POINT('',(0.693717979106305,0.,1.60662857109684));
#26474=CARTESIAN_POINT('Ctrl Pts',(0.7455743247944,-1.,2.0698113262342));
#26475=CARTESIAN_POINT('Ctrl Pts',(0.7455743247944,1.,2.0698113262342));
#26476=CARTESIAN_POINT('Ctrl Pts',(0.745832791378367,-1.,2.06854248895728));
#26477=CARTESIAN_POINT('Ctrl Pts',(0.745832791378367,1.,2.06854248895728));
#26478=CARTESIAN_POINT('Ctrl Pts',(0.7463458715442,-1.,2.06600523016815));
#26479=CARTESIAN_POINT('Ctrl Pts',(0.7463458715442,1.,2.06600523016815));
#26480=CARTESIAN_POINT('Ctrl Pts',(0.747103932787919,-1.,2.06220058927826));
#26481=CARTESIAN_POINT('Ctrl Pts',(0.747103932787919,1.,2.06220058927826));
#26482=CARTESIAN_POINT('Ctrl Pts',(0.748091554183802,-1.,2.05713023031007));
#26483=CARTESIAN_POINT('Ctrl Pts',(0.748091554183802,1.,2.05713023031007));
#26484=CARTESIAN_POINT('Ctrl Pts',(0.749287468665046,-1.,2.05079645592154));
#26485=CARTESIAN_POINT('Ctrl Pts',(0.749287468665046,1.,2.05079645592154));
#26486=CARTESIAN_POINT('Ctrl Pts',(0.750444657875575,-1.,2.04446689147979));
#26487=CARTESIAN_POINT('Ctrl Pts',(0.750444657875575,1.,2.04446689147979));
#26488=CARTESIAN_POINT('Ctrl Pts',(0.751562963361115,-1.,2.03814160092099));
#26489=CARTESIAN_POINT('Ctrl Pts',(0.751562963361115,1.,2.03814160092099));
#26490=CARTESIAN_POINT('Ctrl Pts',(0.75264218048721,-1.,2.03182068456221));
#26491=CARTESIAN_POINT('Ctrl Pts',(0.75264218048721,1.,2.03182068456221));
#26492=CARTESIAN_POINT('Ctrl Pts',(0.753682061112768,-1.,2.02550428623313));
#26493=CARTESIAN_POINT('Ctrl Pts',(0.753682061112768,1.,2.02550428623313));
#26494=CARTESIAN_POINT('Ctrl Pts',(0.754682330722816,-1.,2.01919259405809));
#26495=CARTESIAN_POINT('Ctrl Pts',(0.754682330722816,1.,2.01919259405809));
#26496=CARTESIAN_POINT('Ctrl Pts',(0.755642704957865,-1.,2.01288584328084));
#26497=CARTESIAN_POINT('Ctrl Pts',(0.755642704957865,1.,2.01288584328084));
#26498=CARTESIAN_POINT('Ctrl Pts',(0.75656290464667,-1.,2.0065843158773));
#26499=CARTESIAN_POINT('Ctrl Pts',(0.75656290464667,1.,2.0065843158773));
#26500=CARTESIAN_POINT('Ctrl Pts',(0.757442676862724,-1.,2.00028834739178));
#26501=CARTESIAN_POINT('Ctrl Pts',(0.757442676862724,1.,2.00028834739178));
#26502=CARTESIAN_POINT('Ctrl Pts',(0.758281796766761,-1.,1.99399831098817));
#26503=CARTESIAN_POINT('Ctrl Pts',(0.758281796766761,1.,1.99399831098817));
#26504=CARTESIAN_POINT('Ctrl Pts',(0.759080037802488,-1.,1.98771456680874));
#26505=CARTESIAN_POINT('Ctrl Pts',(0.759080037802488,1.,1.98771456680874));
#26506=CARTESIAN_POINT('Ctrl Pts',(0.75983714745219,-1.,1.98143741418172));
#26507=CARTESIAN_POINT('Ctrl Pts',(0.75983714745219,1.,1.98143741418172));
#26508=CARTESIAN_POINT('Ctrl Pts',(0.760552825409757,-1.,1.97516705321494));
#26509=CARTESIAN_POINT('Ctrl Pts',(0.760552825409757,1.,1.97516705321494));
#26510=CARTESIAN_POINT('Ctrl Pts',(0.76122669048382,-1.,1.96890351582499));
#26511=CARTESIAN_POINT('Ctrl Pts',(0.76122669048382,1.,1.96890351582499));
#26512=CARTESIAN_POINT('Ctrl Pts',(0.761858300014423,-1.,1.96264672744186));
#26513=CARTESIAN_POINT('Ctrl Pts',(0.761858300014423,1.,1.96264672744186));
#26514=CARTESIAN_POINT('Ctrl Pts',(0.762447203806178,-1.,1.95639665309869));
#26515=CARTESIAN_POINT('Ctrl Pts',(0.762447203806178,1.,1.95639665309869));
#26516=CARTESIAN_POINT('Ctrl Pts',(0.762992990878769,-1.,1.95015342590024));
#26517=CARTESIAN_POINT('Ctrl Pts',(0.762992990878769,1.,1.95015342590024));
#26518=CARTESIAN_POINT('Ctrl Pts',(0.763495333538629,-1.,1.9439174661764));
#26519=CARTESIAN_POINT('Ctrl Pts',(0.763495333538629,1.,1.9439174661764));
#26520=CARTESIAN_POINT('Ctrl Pts',(0.763954049121458,-1.,1.93768964875886));
#26521=CARTESIAN_POINT('Ctrl Pts',(0.763954049121458,1.,1.93768964875886));
#26522=CARTESIAN_POINT('Ctrl Pts',(0.76436901067394,-1.,1.93147105496382));
#26523=CARTESIAN_POINT('Ctrl Pts',(0.76436901067394,1.,1.93147105496382));
#26524=CARTESIAN_POINT('Ctrl Pts',(0.764740025488211,-1.,1.92526263537048));
#26525=CARTESIAN_POINT('Ctrl Pts',(0.764740025488211,1.,1.92526263537048));
#26526=CARTESIAN_POINT('Ctrl Pts',(0.765066729667088,-1.,1.91906491634196));
#26527=CARTESIAN_POINT('Ctrl Pts',(0.765066729667088,1.,1.91906491634196));
#26528=CARTESIAN_POINT('Ctrl Pts',(0.765348465884722,-1.,1.91287765805169));
#26529=CARTESIAN_POINT('Ctrl Pts',(0.765348465884722,1.,1.91287765805169));
#26530=CARTESIAN_POINT('Ctrl Pts',(0.765584196937919,-1.,1.90669961402356));
#26531=CARTESIAN_POINT('Ctrl Pts',(0.765584196937919,1.,1.90669961402356));
#26532=CARTESIAN_POINT('Ctrl Pts',(0.765772772593386,-1.,1.90052930393596));
#26533=CARTESIAN_POINT('Ctrl Pts',(0.765772772593386,1.,1.90052930393596));
#26534=CARTESIAN_POINT('Ctrl Pts',(0.765913193856978,-1.,1.89436577771388));
#26535=CARTESIAN_POINT('Ctrl Pts',(0.765913193856978,1.,1.89436577771388));
#26536=CARTESIAN_POINT('Ctrl Pts',(0.766004837062091,-1.,1.88820926433409));
#26537=CARTESIAN_POINT('Ctrl Pts',(0.766004837062091,1.,1.88820926433409));
#26538=CARTESIAN_POINT('Ctrl Pts',(0.766047794851864,-1.,1.88206215302561));
#26539=CARTESIAN_POINT('Ctrl Pts',(0.766047794851864,1.,1.88206215302561));
#26540=CARTESIAN_POINT('Ctrl Pts',(0.766042837036744,-1.,1.87592888967883));
#26541=CARTESIAN_POINT('Ctrl Pts',(0.766042837036744,1.,1.87592888967883));
#26542=CARTESIAN_POINT('Ctrl Pts',(0.765990708546091,-1.,1.86981398314341));
#26543=CARTESIAN_POINT('Ctrl Pts',(0.765990708546091,1.,1.86981398314341));
#26544=CARTESIAN_POINT('Ctrl Pts',(0.765891519092547,-1.,1.86372027063312));
#26545=CARTESIAN_POINT('Ctrl Pts',(0.765891519092547,1.,1.86372027063312));
#26546=CARTESIAN_POINT('Ctrl Pts',(0.765744212909318,-1.,1.85764741390394));
#26547=CARTESIAN_POINT('Ctrl Pts',(0.765744212909318,1.,1.85764741390394));
#26548=CARTESIAN_POINT('Ctrl Pts',(0.765545710619062,-1.,1.85158945130063));
#26549=CARTESIAN_POINT('Ctrl Pts',(0.765545710619062,1.,1.85158945130063));
#26550=CARTESIAN_POINT('Ctrl Pts',(0.765291664862029,-1.,1.84553698875924));
#26551=CARTESIAN_POINT('Ctrl Pts',(0.765291664862029,1.,1.84553698875924));
#26552=CARTESIAN_POINT('Ctrl Pts',(0.764978057881737,-1.,1.83948181064835));
#26553=CARTESIAN_POINT('Ctrl Pts',(0.764978057881737,1.,1.83948181064835));
#26554=CARTESIAN_POINT('Ctrl Pts',(0.764602549687853,-1.,1.83342077227142));
#26555=CARTESIAN_POINT('Ctrl Pts',(0.764602549687853,1.,1.83342077227142));
#26556=CARTESIAN_POINT('Ctrl Pts',(0.764165902605995,-1.,1.82735991200065));
#26557=CARTESIAN_POINT('Ctrl Pts',(0.764165902605995,1.,1.82735991200065));
#26558=CARTESIAN_POINT('Ctrl Pts',(0.763673465462726,-1.,1.82131873145266));
#26559=CARTESIAN_POINT('Ctrl Pts',(0.763673465462726,1.,1.82131873145266));
#26560=CARTESIAN_POINT('Ctrl Pts',(0.763132003836634,-1.,1.8153211840553));
#26561=CARTESIAN_POINT('Ctrl Pts',(0.763132003836634,1.,1.8153211840553));
#26562=CARTESIAN_POINT('Ctrl Pts',(0.762546129463938,-1.,1.80938551463965));
#26563=CARTESIAN_POINT('Ctrl Pts',(0.762546129463938,1.,1.80938551463965));
#26564=CARTESIAN_POINT('Ctrl Pts',(0.761915336443547,-1.,1.80351583877342));
#26565=CARTESIAN_POINT('Ctrl Pts',(0.761915336443547,1.,1.80351583877342));
#26566=CARTESIAN_POINT('Ctrl Pts',(0.761229695230558,-1.,1.79768986997783));
#26567=CARTESIAN_POINT('Ctrl Pts',(0.761229695230558,1.,1.79768986997783));
#26568=CARTESIAN_POINT('Ctrl Pts',(0.760469555880749,-1.,1.7918581561088));
#26569=CARTESIAN_POINT('Ctrl Pts',(0.760469555880749,1.,1.7918581561088));
#26570=CARTESIAN_POINT('Ctrl Pts',(0.759614401110189,-1.,1.78596964884604));
#26571=CARTESIAN_POINT('Ctrl Pts',(0.759614401110189,1.,1.78596964884604));
#26572=CARTESIAN_POINT('Ctrl Pts',(0.758650626677518,-1.,1.77999411220945));
#26573=CARTESIAN_POINT('Ctrl Pts',(0.758650626677518,1.,1.77999411220945));
#26574=CARTESIAN_POINT('Ctrl Pts',(0.757578264077028,-1.,1.77394167108292));
#26575=CARTESIAN_POINT('Ctrl Pts',(0.757578264077028,1.,1.77394167108292));
#26576=CARTESIAN_POINT('Ctrl Pts',(0.75642189602781,-1.,1.76789396002998));
#26577=CARTESIAN_POINT('Ctrl Pts',(0.75642189602781,1.,1.76789396002998));
#26578=CARTESIAN_POINT('Ctrl Pts',(0.755220979974461,-1.,1.76197817240128));
#26579=CARTESIAN_POINT('Ctrl Pts',(0.755220979974461,1.,1.76197817240128));
#26580=CARTESIAN_POINT('Ctrl Pts',(0.754009254027828,-1.,1.75631083600019));
#26581=CARTESIAN_POINT('Ctrl Pts',(0.754009254027828,1.,1.75631083600019));
#26582=CARTESIAN_POINT('Ctrl Pts',(0.752797683531314,-1.,1.75095139468794));
#26583=CARTESIAN_POINT('Ctrl Pts',(0.752797683531314,1.,1.75095139468794));
#26584=CARTESIAN_POINT('Ctrl Pts',(0.751555614164482,-1.,1.74585086852502));
#26585=CARTESIAN_POINT('Ctrl Pts',(0.751555614164482,1.,1.74585086852502));
#26586=CARTESIAN_POINT('Ctrl Pts',(0.750193435981249,-1.,1.74080458267114));
#26587=CARTESIAN_POINT('Ctrl Pts',(0.750193435981249,1.,1.74080458267114));
#26588=CARTESIAN_POINT('Ctrl Pts',(0.74858246295687,-1.,1.7355035168033));
#26589=CARTESIAN_POINT('Ctrl Pts',(0.74858246295687,1.,1.7355035168033));
#26590=CARTESIAN_POINT('Ctrl Pts',(0.746574710097752,-1.,1.72958533647714));
#26591=CARTESIAN_POINT('Ctrl Pts',(0.746574710097752,1.,1.72958533647714));
#26592=CARTESIAN_POINT('Ctrl Pts',(0.744021445433093,-1.,1.72268229916769));
#26593=CARTESIAN_POINT('Ctrl Pts',(0.744021445433093,1.,1.72268229916769));
#26594=CARTESIAN_POINT('Ctrl Pts',(0.74079516202821,-1.,1.71447789751001));
#26595=CARTESIAN_POINT('Ctrl Pts',(0.74079516202821,1.,1.71447789751001));
#26596=CARTESIAN_POINT('Ctrl Pts',(0.736799665716932,-1.,1.70473309004249));
#26597=CARTESIAN_POINT('Ctrl Pts',(0.736799665716932,1.,1.70473309004249));
#26598=CARTESIAN_POINT('Ctrl Pts',(0.731963238685357,-1.,1.69326921972915));
#26599=CARTESIAN_POINT('Ctrl Pts',(0.731963238685357,1.,1.69326921972915));
#26600=CARTESIAN_POINT('Ctrl Pts',(0.726235967982445,-1.,1.67996158451922));
#26601=CARTESIAN_POINT('Ctrl Pts',(0.726235967982445,1.,1.67996158451922));
#26602=CARTESIAN_POINT('Ctrl Pts',(0.719585433787949,-1.,1.66472880551777));
#26603=CARTESIAN_POINT('Ctrl Pts',(0.719585433787949,1.,1.66472880551777));
#26604=CARTESIAN_POINT('Ctrl Pts',(0.711993139340447,-1.,1.64752408828442));
#26605=CARTESIAN_POINT('Ctrl Pts',(0.711993139340447,1.,1.64752408828442));
#26606=CARTESIAN_POINT('Ctrl Pts',(0.705159151977294,-1.,1.6321654166204));
#26607=CARTESIAN_POINT('Ctrl Pts',(0.705159151977294,1.,1.6321654166204));
#26608=CARTESIAN_POINT('Ctrl Pts',(0.699605146398836,-1.,1.61974673471117));
#26609=CARTESIAN_POINT('Ctrl Pts',(0.699605146398836,1.,1.61974673471117));
#26610=CARTESIAN_POINT('Ctrl Pts',(0.69571209787897,-1.,1.61106790957619));
#26611=CARTESIAN_POINT('Ctrl Pts',(0.69571209787897,1.,1.61106790957619));
#26612=CARTESIAN_POINT('Ctrl Pts',(0.693717979106305,-1.,1.60662857109684));
#26613=CARTESIAN_POINT('Ctrl Pts',(0.693717979106305,1.,1.60662857109684));
#26614=CARTESIAN_POINT('',(0.7455743247944,1.,2.0698113262342));
#26615=CARTESIAN_POINT('Ctrl Pts',(0.7455743247944,1.,2.0698113262342));
#26616=CARTESIAN_POINT('Ctrl Pts',(0.745832791378367,1.,2.06854248895728));
#26617=CARTESIAN_POINT('Ctrl Pts',(0.7463458715442,1.,2.06600523016815));
#26618=CARTESIAN_POINT('Ctrl Pts',(0.747103932787919,1.,2.06220058927826));
#26619=CARTESIAN_POINT('Ctrl Pts',(0.748091554183802,1.,2.05713023031007));
#26620=CARTESIAN_POINT('Ctrl Pts',(0.749287468665046,1.,2.05079645592154));
#26621=CARTESIAN_POINT('Ctrl Pts',(0.750444657875575,1.,2.04446689147979));
#26622=CARTESIAN_POINT('Ctrl Pts',(0.751562963361115,1.,2.03814160092099));
#26623=CARTESIAN_POINT('Ctrl Pts',(0.75264218048721,1.,2.03182068456221));
#26624=CARTESIAN_POINT('Ctrl Pts',(0.753682061112768,1.,2.02550428623313));
#26625=CARTESIAN_POINT('Ctrl Pts',(0.754682330722816,1.,2.01919259405809));
#26626=CARTESIAN_POINT('Ctrl Pts',(0.755642704957865,1.,2.01288584328084));
#26627=CARTESIAN_POINT('Ctrl Pts',(0.75656290464667,1.,2.0065843158773));
#26628=CARTESIAN_POINT('Ctrl Pts',(0.757442676862724,1.,2.00028834739178));
#26629=CARTESIAN_POINT('Ctrl Pts',(0.758281796766761,1.,1.99399831098817));
#26630=CARTESIAN_POINT('Ctrl Pts',(0.759080037802488,1.,1.98771456680874));
#26631=CARTESIAN_POINT('Ctrl Pts',(0.75983714745219,1.,1.98143741418172));
#26632=CARTESIAN_POINT('Ctrl Pts',(0.760552825409757,1.,1.97516705321494));
#26633=CARTESIAN_POINT('Ctrl Pts',(0.76122669048382,1.,1.96890351582499));
#26634=CARTESIAN_POINT('Ctrl Pts',(0.761858300014423,1.,1.96264672744186));
#26635=CARTESIAN_POINT('Ctrl Pts',(0.762447203806178,1.,1.95639665309869));
#26636=CARTESIAN_POINT('Ctrl Pts',(0.762992990878769,1.,1.95015342590024));
#26637=CARTESIAN_POINT('Ctrl Pts',(0.763495333538629,1.,1.9439174661764));
#26638=CARTESIAN_POINT('Ctrl Pts',(0.763954049121458,1.,1.93768964875886));
#26639=CARTESIAN_POINT('Ctrl Pts',(0.76436901067394,1.,1.93147105496382));
#26640=CARTESIAN_POINT('Ctrl Pts',(0.764740025488211,1.,1.92526263537048));
#26641=CARTESIAN_POINT('Ctrl Pts',(0.765066729667088,1.,1.91906491634196));
#26642=CARTESIAN_POINT('Ctrl Pts',(0.765348465884722,1.,1.91287765805169));
#26643=CARTESIAN_POINT('Ctrl Pts',(0.765584196937919,1.,1.90669961402356));
#26644=CARTESIAN_POINT('Ctrl Pts',(0.765772772593386,1.,1.90052930393596));
#26645=CARTESIAN_POINT('Ctrl Pts',(0.765913193856978,1.,1.89436577771388));
#26646=CARTESIAN_POINT('Ctrl Pts',(0.766004837062091,1.,1.88820926433409));
#26647=CARTESIAN_POINT('Ctrl Pts',(0.766047794851864,1.,1.88206215302561));
#26648=CARTESIAN_POINT('Ctrl Pts',(0.766042837036744,1.,1.87592888967883));
#26649=CARTESIAN_POINT('Ctrl Pts',(0.765990708546091,1.,1.86981398314341));
#26650=CARTESIAN_POINT('Ctrl Pts',(0.765891519092547,1.,1.86372027063312));
#26651=CARTESIAN_POINT('Ctrl Pts',(0.765744212909318,1.,1.85764741390394));
#26652=CARTESIAN_POINT('Ctrl Pts',(0.765545710619062,1.,1.85158945130063));
#26653=CARTESIAN_POINT('Ctrl Pts',(0.765291664862029,1.,1.84553698875924));
#26654=CARTESIAN_POINT('Ctrl Pts',(0.764978057881737,1.,1.83948181064835));
#26655=CARTESIAN_POINT('Ctrl Pts',(0.764602549687853,1.,1.83342077227142));
#26656=CARTESIAN_POINT('Ctrl Pts',(0.764165902605995,1.,1.82735991200065));
#26657=CARTESIAN_POINT('Ctrl Pts',(0.763673465462726,1.,1.82131873145266));
#26658=CARTESIAN_POINT('Ctrl Pts',(0.763132003836634,1.,1.8153211840553));
#26659=CARTESIAN_POINT('Ctrl Pts',(0.762546129463938,1.,1.80938551463965));
#26660=CARTESIAN_POINT('Ctrl Pts',(0.761915336443547,1.,1.80351583877342));
#26661=CARTESIAN_POINT('Ctrl Pts',(0.761229695230558,1.,1.79768986997783));
#26662=CARTESIAN_POINT('Ctrl Pts',(0.760469555880749,1.,1.7918581561088));
#26663=CARTESIAN_POINT('Ctrl Pts',(0.759614401110189,1.,1.78596964884604));
#26664=CARTESIAN_POINT('Ctrl Pts',(0.758650626677518,1.,1.77999411220945));
#26665=CARTESIAN_POINT('Ctrl Pts',(0.757578264077028,1.,1.77394167108292));
#26666=CARTESIAN_POINT('Ctrl Pts',(0.75642189602781,1.,1.76789396002998));
#26667=CARTESIAN_POINT('Ctrl Pts',(0.755220979974461,1.,1.76197817240128));
#26668=CARTESIAN_POINT('Ctrl Pts',(0.754009254027828,1.,1.75631083600019));
#26669=CARTESIAN_POINT('Ctrl Pts',(0.752797683531314,1.,1.75095139468794));
#26670=CARTESIAN_POINT('Ctrl Pts',(0.751555614164482,1.,1.74585086852502));
#26671=CARTESIAN_POINT('Ctrl Pts',(0.750193435981249,1.,1.74080458267114));
#26672=CARTESIAN_POINT('Ctrl Pts',(0.74858246295687,1.,1.7355035168033));
#26673=CARTESIAN_POINT('Ctrl Pts',(0.746574710097752,1.,1.72958533647714));
#26674=CARTESIAN_POINT('Ctrl Pts',(0.744021445433093,1.,1.72268229916769));
#26675=CARTESIAN_POINT('Ctrl Pts',(0.74079516202821,1.,1.71447789751001));
#26676=CARTESIAN_POINT('Ctrl Pts',(0.736799665716932,1.,1.70473309004249));
#26677=CARTESIAN_POINT('Ctrl Pts',(0.731963238685357,1.,1.69326921972915));
#26678=CARTESIAN_POINT('Ctrl Pts',(0.726235967982445,1.,1.67996158451922));
#26679=CARTESIAN_POINT('Ctrl Pts',(0.719585433787949,1.,1.66472880551777));
#26680=CARTESIAN_POINT('Ctrl Pts',(0.711993139340447,1.,1.64752408828442));
#26681=CARTESIAN_POINT('Ctrl Pts',(0.705159151977294,1.,1.6321654166204));
#26682=CARTESIAN_POINT('Ctrl Pts',(0.699605146398836,1.,1.61974673471117));
#26683=CARTESIAN_POINT('Ctrl Pts',(0.69571209787897,1.,1.61106790957619));
#26684=CARTESIAN_POINT('Ctrl Pts',(0.693717979106305,1.,1.60662857109684));
#26685=CARTESIAN_POINT('',(0.7455743247944,0.,2.0698113262342));
#26686=CARTESIAN_POINT('Origin',(0.61342227326009,0.,2.11275013067528));
#26687=CARTESIAN_POINT('',(0.61342227326009,1.,2.11275013067528));
#26688=CARTESIAN_POINT('',(0.7455743247944,1.,2.0698113262342));
#26689=CARTESIAN_POINT('',(0.61342227326009,0.,2.11275013067528));
#26690=CARTESIAN_POINT('Ctrl Pts',(0.383122945602004,-1.,1.7075470150345));
#26691=CARTESIAN_POINT('Ctrl Pts',(0.383122945602004,1.,1.7075470150345));
#26692=CARTESIAN_POINT('Ctrl Pts',(0.384119047315541,-1.,1.71231062891958));
#26693=CARTESIAN_POINT('Ctrl Pts',(0.384119047315541,1.,1.71231062891958));
#26694=CARTESIAN_POINT('Ctrl Pts',(0.38607079032701,-1.,1.72162022246158));
#26695=CARTESIAN_POINT('Ctrl Pts',(0.38607079032701,1.,1.72162022246158));
#26696=CARTESIAN_POINT('Ctrl Pts',(0.388877023509191,-1.,1.7349317097561));
#26697=CARTESIAN_POINT('Ctrl Pts',(0.388877023509191,1.,1.7349317097561));
#26698=CARTESIAN_POINT('Ctrl Pts',(0.392375812294307,-1.,1.75137405313962));
#26699=CARTESIAN_POINT('Ctrl Pts',(0.392375812294307,1.,1.75137405313962));
#26700=CARTESIAN_POINT('Ctrl Pts',(0.39634619612042,-1.,1.7697556004756));
#26701=CARTESIAN_POINT('Ctrl Pts',(0.39634619612042,1.,1.7697556004756));
#26702=CARTESIAN_POINT('Ctrl Pts',(0.39991940378308,-1.,1.78598826347533));
#26703=CARTESIAN_POINT('Ctrl Pts',(0.39991940378308,1.,1.78598826347533));
#26704=CARTESIAN_POINT('Ctrl Pts',(0.403107976170441,-1.,1.80012077176221));
#26705=CARTESIAN_POINT('Ctrl Pts',(0.403107976170441,1.,1.80012077176221));
#26706=CARTESIAN_POINT('Ctrl Pts',(0.405933518411838,-1.,1.81223801813988));
#26707=CARTESIAN_POINT('Ctrl Pts',(0.405933518411838,1.,1.81223801813988));
#26708=CARTESIAN_POINT('Ctrl Pts',(0.408428948108533,-1.,1.8224702267854));
#26709=CARTESIAN_POINT('Ctrl Pts',(0.408428948108533,1.,1.8224702267854));
#26710=CARTESIAN_POINT('Ctrl Pts',(0.410641256301674,-1.,1.83100408895216));
#26711=CARTESIAN_POINT('Ctrl Pts',(0.410641256301674,1.,1.83100408895216));
#26712=CARTESIAN_POINT('Ctrl Pts',(0.412633125322161,-1.,1.83808953475839));
#26713=CARTESIAN_POINT('Ctrl Pts',(0.412633125322161,1.,1.83808953475839));
#26714=CARTESIAN_POINT('Ctrl Pts',(0.41448743825434,-1.,1.8440575707371));
#26715=CARTESIAN_POINT('Ctrl Pts',(0.41448743825434,1.,1.8440575707371));
#26716=CARTESIAN_POINT('Ctrl Pts',(0.416300022038864,-1.,1.84929312929882));
#26717=CARTESIAN_POINT('Ctrl Pts',(0.416300022038864,1.,1.84929312929882));
#26718=CARTESIAN_POINT('Ctrl Pts',(0.418164129143534,-1.,1.85417632856234));
#26719=CARTESIAN_POINT('Ctrl Pts',(0.418164129143534,1.,1.85417632856234));
#26720=CARTESIAN_POINT('Ctrl Pts',(0.420157287975619,-1.,1.85903281096686));
#26721=CARTESIAN_POINT('Ctrl Pts',(0.420157287975619,1.,1.85903281096686));
#26722=CARTESIAN_POINT('Ctrl Pts',(0.422327307418275,-1.,1.86408083334028));
#26723=CARTESIAN_POINT('Ctrl Pts',(0.422327307418275,1.,1.86408083334028));
#26724=CARTESIAN_POINT('Ctrl Pts',(0.424678177291358,-1.,1.86937803944323));
#26725=CARTESIAN_POINT('Ctrl Pts',(0.424678177291358,1.,1.86937803944323));
#26726=CARTESIAN_POINT('Ctrl Pts',(0.427183828519102,-1.,1.87486989291484));
#26727=CARTESIAN_POINT('Ctrl Pts',(0.427183828519102,1.,1.87486989291484));
#26728=CARTESIAN_POINT('Ctrl Pts',(0.429803062482344,-1.,1.88044229001832));
#26729=CARTESIAN_POINT('Ctrl Pts',(0.429803062482344,1.,1.88044229001832));
#26730=CARTESIAN_POINT('Ctrl Pts',(0.432493038548748,-1.,1.88596913666793));
#26731=CARTESIAN_POINT('Ctrl Pts',(0.432493038548748,1.,1.88596913666793));
#26732=CARTESIAN_POINT('Ctrl Pts',(0.435225660963383,-1.,1.89136993975504));
#26733=CARTESIAN_POINT('Ctrl Pts',(0.435225660963383,1.,1.89136993975504));
#26734=CARTESIAN_POINT('Ctrl Pts',(0.437995003948244,-1.,1.89663648956466));
#26735=CARTESIAN_POINT('Ctrl Pts',(0.437995003948244,1.,1.89663648956466));
#26736=CARTESIAN_POINT('Ctrl Pts',(0.440807833704038,-1.,1.90180124389086));
#26737=CARTESIAN_POINT('Ctrl Pts',(0.440807833704038,1.,1.90180124389086));
#26738=CARTESIAN_POINT('Ctrl Pts',(0.44367755684915,-1.,1.90691756144898));
#26739=CARTESIAN_POINT('Ctrl Pts',(0.44367755684915,1.,1.90691756144898));
#26740=CARTESIAN_POINT('Ctrl Pts',(0.446617343485711,-1.,1.9120369998112));
#26741=CARTESIAN_POINT('Ctrl Pts',(0.446617343485711,1.,1.9120369998112));
#26742=CARTESIAN_POINT('Ctrl Pts',(0.449632260106662,-1.,1.91718342555755));
#26743=CARTESIAN_POINT('Ctrl Pts',(0.449632260106662,1.,1.91718342555755));
#26744=CARTESIAN_POINT('Ctrl Pts',(0.452719478359432,-1.,1.92235380648502));
#26745=CARTESIAN_POINT('Ctrl Pts',(0.452719478359432,1.,1.92235380648502));
#26746=CARTESIAN_POINT('Ctrl Pts',(0.45587200517437,-1.,1.92753067150476));
#26747=CARTESIAN_POINT('Ctrl Pts',(0.45587200517437,1.,1.92753067150476));
#26748=CARTESIAN_POINT('Ctrl Pts',(0.459081234547926,-1.,1.93269066517934));
#26749=CARTESIAN_POINT('Ctrl Pts',(0.459081234547926,1.,1.93269066517934));
#26750=CARTESIAN_POINT('Ctrl Pts',(0.462340031009056,-1.,1.93781486640821));
#26751=CARTESIAN_POINT('Ctrl Pts',(0.462340031009056,1.,1.93781486640821));
#26752=CARTESIAN_POINT('Ctrl Pts',(0.46564546202603,-1.,1.9428979419619));
#26753=CARTESIAN_POINT('Ctrl Pts',(0.46564546202603,1.,1.9428979419619));
#26754=CARTESIAN_POINT('Ctrl Pts',(0.468997482913135,-1.,1.94794381136514));
#26755=CARTESIAN_POINT('Ctrl Pts',(0.468997482913135,1.,1.94794381136514));
#26756=CARTESIAN_POINT('Ctrl Pts',(0.472397672264072,-1.,1.95296148278133));
#26757=CARTESIAN_POINT('Ctrl Pts',(0.472397672264072,1.,1.95296148278133));
#26758=CARTESIAN_POINT('Ctrl Pts',(0.475848034683176,-1.,1.95796111148177));
#26759=CARTESIAN_POINT('Ctrl Pts',(0.475848034683176,1.,1.95796111148177));
#26760=CARTESIAN_POINT('Ctrl Pts',(0.479349583074855,-1.,1.96294933055943));
#26761=CARTESIAN_POINT('Ctrl Pts',(0.479349583074855,1.,1.96294933055943));
#26762=CARTESIAN_POINT('Ctrl Pts',(0.48290166212069,-1.,1.96792703422362));
#26763=CARTESIAN_POINT('Ctrl Pts',(0.48290166212069,1.,1.96792703422362));
#26764=CARTESIAN_POINT('Ctrl Pts',(0.486502692907658,-1.,1.97289186263272));
#26765=CARTESIAN_POINT('Ctrl Pts',(0.486502692907658,1.,1.97289186263272));
#26766=CARTESIAN_POINT('Ctrl Pts',(0.490150627860952,-1.,1.97783973019229));
#26767=CARTESIAN_POINT('Ctrl Pts',(0.490150627860952,1.,1.97783973019229));
#26768=CARTESIAN_POINT('Ctrl Pts',(0.493843476541494,-1.,1.98276658761821));
#26769=CARTESIAN_POINT('Ctrl Pts',(0.493843476541494,1.,1.98276658761821));
#26770=CARTESIAN_POINT('Ctrl Pts',(0.497579909545574,-1.,1.98767044752932));
#26771=CARTESIAN_POINT('Ctrl Pts',(0.497579909545574,1.,1.98767044752932));
#26772=CARTESIAN_POINT('Ctrl Pts',(0.501359287727146,-1.,1.99255149126155));
#26773=CARTESIAN_POINT('Ctrl Pts',(0.501359287727146,1.,1.99255149126155));
#26774=CARTESIAN_POINT('Ctrl Pts',(0.505181361323026,-1.,1.99741107463572));
#26775=CARTESIAN_POINT('Ctrl Pts',(0.505181361323026,1.,1.99741107463572));
#26776=CARTESIAN_POINT('Ctrl Pts',(0.509046069886157,-1.,2.00225107134734));
#26777=CARTESIAN_POINT('Ctrl Pts',(0.509046069886157,1.,2.00225107134734));
#26778=CARTESIAN_POINT('Ctrl Pts',(0.512953306961792,-1.,2.00707309946949));
#26779=CARTESIAN_POINT('Ctrl Pts',(0.512953306961792,1.,2.00707309946949));
#26780=CARTESIAN_POINT('Ctrl Pts',(0.516902681728687,-1.,2.01187773939242));
#26781=CARTESIAN_POINT('Ctrl Pts',(0.516902681728687,1.,2.01187773939242));
#26782=CARTESIAN_POINT('Ctrl Pts',(0.52089359039937,-1.,2.01666477917286));
#26783=CARTESIAN_POINT('Ctrl Pts',(0.52089359039937,1.,2.01666477917286));
#26784=CARTESIAN_POINT('Ctrl Pts',(0.524925318333476,-1.,2.02143356304698));
#26785=CARTESIAN_POINT('Ctrl Pts',(0.524925318333476,1.,2.02143356304698));
#26786=CARTESIAN_POINT('Ctrl Pts',(0.528997127241914,-1.,2.0261832908329));
#26787=CARTESIAN_POINT('Ctrl Pts',(0.528997127241914,1.,2.0261832908329));
#26788=CARTESIAN_POINT('Ctrl Pts',(0.533108355132976,-1.,2.03091336214426));
#26789=CARTESIAN_POINT('Ctrl Pts',(0.533108355132976,1.,2.03091336214426));
#26790=CARTESIAN_POINT('Ctrl Pts',(0.537258489833262,-1.,2.03562362954037));
#26791=CARTESIAN_POINT('Ctrl Pts',(0.537258489833262,1.,2.03562362954037));
#26792=CARTESIAN_POINT('Ctrl Pts',(0.541447120615659,-1.,2.04031422690527));
#26793=CARTESIAN_POINT('Ctrl Pts',(0.541447120615659,1.,2.04031422690527));
#26794=CARTESIAN_POINT('Ctrl Pts',(0.54567390381743,-1.,2.04498544714588));
#26795=CARTESIAN_POINT('Ctrl Pts',(0.54567390381743,1.,2.04498544714588));
#26796=CARTESIAN_POINT('Ctrl Pts',(0.549938525150295,-1.,2.04963761077958));
#26797=CARTESIAN_POINT('Ctrl Pts',(0.549938525150295,1.,2.04963761077958));
#26798=CARTESIAN_POINT('Ctrl Pts',(0.554240657463906,-1.,2.05427091604413));
#26799=CARTESIAN_POINT('Ctrl Pts',(0.554240657463906,1.,2.05427091604413));
#26800=CARTESIAN_POINT('Ctrl Pts',(0.558579940185151,-1.,2.05888537756462));
#26801=CARTESIAN_POINT('Ctrl Pts',(0.558579940185151,1.,2.05888537756462));
#26802=CARTESIAN_POINT('Ctrl Pts',(0.562955993082261,-1.,2.06348090160589));
#26803=CARTESIAN_POINT('Ctrl Pts',(0.562955993082261,1.,2.06348090160589));
#26804=CARTESIAN_POINT('Ctrl Pts',(0.567368421181087,-1.,2.06805732997334));
#26805=CARTESIAN_POINT('Ctrl Pts',(0.567368421181087,1.,2.06805732997334));
#26806=CARTESIAN_POINT('Ctrl Pts',(0.571816823242602,-1.,2.07261449292824));
#26807=CARTESIAN_POINT('Ctrl Pts',(0.571816823242602,1.,2.07261449292824));
#26808=CARTESIAN_POINT('Ctrl Pts',(0.576300797416844,-1.,2.07715226767559));
#26809=CARTESIAN_POINT('Ctrl Pts',(0.576300797416844,1.,2.07715226767559));
#26810=CARTESIAN_POINT('Ctrl Pts',(0.580819952108063,-1.,2.08167059018418));
#26811=CARTESIAN_POINT('Ctrl Pts',(0.580819952108063,1.,2.08167059018418));
#26812=CARTESIAN_POINT('Ctrl Pts',(0.585373918991617,-1.,2.08616943727951));
#26813=CARTESIAN_POINT('Ctrl Pts',(0.585373918991617,1.,2.08616943727951));
#26814=CARTESIAN_POINT('Ctrl Pts',(0.589962365403406,-1.,2.09064881812129));
#26815=CARTESIAN_POINT('Ctrl Pts',(0.589962365403406,1.,2.09064881812129));
#26816=CARTESIAN_POINT('Ctrl Pts',(0.594585006052162,-1.,2.0951087622027));
#26817=CARTESIAN_POINT('Ctrl Pts',(0.594585006052162,1.,2.0951087622027));
#26818=CARTESIAN_POINT('Ctrl Pts',(0.599241616420533,-1.,2.0995493086477));
#26819=CARTESIAN_POINT('Ctrl Pts',(0.599241616420533,1.,2.0995493086477));
#26820=CARTESIAN_POINT('Ctrl Pts',(0.60393203073603,-1.,2.10397049886949));
#26821=CARTESIAN_POINT('Ctrl Pts',(0.60393203073603,1.,2.10397049886949));
#26822=CARTESIAN_POINT('Ctrl Pts',(0.607711315454876,-1.,2.1074919961518));
#26823=CARTESIAN_POINT('Ctrl Pts',(0.607711315454876,1.,2.1074919961518));
#26824=CARTESIAN_POINT('Ctrl Pts',(0.610560911689898,-1.,2.11012443807238));
#26825=CARTESIAN_POINT('Ctrl Pts',(0.610560911689898,1.,2.11012443807238));
#26826=CARTESIAN_POINT('Ctrl Pts',(0.6124673655618,-1.,2.11187554259986));
#26827=CARTESIAN_POINT('Ctrl Pts',(0.6124673655618,1.,2.11187554259986));
#26828=CARTESIAN_POINT('Ctrl Pts',(0.61342227326009,-1.,2.11275013067528));
#26829=CARTESIAN_POINT('Ctrl Pts',(0.61342227326009,1.,2.11275013067528));
#26830=CARTESIAN_POINT('',(0.383122945602004,1.,1.7075470150345));
#26831=CARTESIAN_POINT('Ctrl Pts',(0.383122945602004,1.,1.7075470150345));
#26832=CARTESIAN_POINT('Ctrl Pts',(0.384119047315541,1.,1.71231062891958));
#26833=CARTESIAN_POINT('Ctrl Pts',(0.38607079032701,1.,1.72162022246158));
#26834=CARTESIAN_POINT('Ctrl Pts',(0.388877023509191,1.,1.7349317097561));
#26835=CARTESIAN_POINT('Ctrl Pts',(0.392375812294307,1.,1.75137405313962));
#26836=CARTESIAN_POINT('Ctrl Pts',(0.39634619612042,1.,1.7697556004756));
#26837=CARTESIAN_POINT('Ctrl Pts',(0.39991940378308,1.,1.78598826347533));
#26838=CARTESIAN_POINT('Ctrl Pts',(0.403107976170441,1.,1.80012077176221));
#26839=CARTESIAN_POINT('Ctrl Pts',(0.405933518411838,1.,1.81223801813988));
#26840=CARTESIAN_POINT('Ctrl Pts',(0.408428948108533,1.,1.8224702267854));
#26841=CARTESIAN_POINT('Ctrl Pts',(0.410641256301674,1.,1.83100408895216));
#26842=CARTESIAN_POINT('Ctrl Pts',(0.412633125322161,1.,1.83808953475839));
#26843=CARTESIAN_POINT('Ctrl Pts',(0.41448743825434,1.,1.8440575707371));
#26844=CARTESIAN_POINT('Ctrl Pts',(0.416300022038864,1.,1.84929312929882));
#26845=CARTESIAN_POINT('Ctrl Pts',(0.418164129143534,1.,1.85417632856234));
#26846=CARTESIAN_POINT('Ctrl Pts',(0.420157287975619,1.,1.85903281096686));
#26847=CARTESIAN_POINT('Ctrl Pts',(0.422327307418275,1.,1.86408083334028));
#26848=CARTESIAN_POINT('Ctrl Pts',(0.424678177291358,1.,1.86937803944323));
#26849=CARTESIAN_POINT('Ctrl Pts',(0.427183828519102,1.,1.87486989291484));
#26850=CARTESIAN_POINT('Ctrl Pts',(0.429803062482344,1.,1.88044229001832));
#26851=CARTESIAN_POINT('Ctrl Pts',(0.432493038548748,1.,1.88596913666793));
#26852=CARTESIAN_POINT('Ctrl Pts',(0.435225660963383,1.,1.89136993975504));
#26853=CARTESIAN_POINT('Ctrl Pts',(0.437995003948244,1.,1.89663648956466));
#26854=CARTESIAN_POINT('Ctrl Pts',(0.440807833704038,1.,1.90180124389086));
#26855=CARTESIAN_POINT('Ctrl Pts',(0.44367755684915,1.,1.90691756144898));
#26856=CARTESIAN_POINT('Ctrl Pts',(0.446617343485711,1.,1.9120369998112));
#26857=CARTESIAN_POINT('Ctrl Pts',(0.449632260106662,1.,1.91718342555755));
#26858=CARTESIAN_POINT('Ctrl Pts',(0.452719478359432,1.,1.92235380648502));
#26859=CARTESIAN_POINT('Ctrl Pts',(0.45587200517437,1.,1.92753067150476));
#26860=CARTESIAN_POINT('Ctrl Pts',(0.459081234547926,1.,1.93269066517934));
#26861=CARTESIAN_POINT('Ctrl Pts',(0.462340031009056,1.,1.93781486640821));
#26862=CARTESIAN_POINT('Ctrl Pts',(0.46564546202603,1.,1.9428979419619));
#26863=CARTESIAN_POINT('Ctrl Pts',(0.468997482913135,1.,1.94794381136514));
#26864=CARTESIAN_POINT('Ctrl Pts',(0.472397672264072,1.,1.95296148278133));
#26865=CARTESIAN_POINT('Ctrl Pts',(0.475848034683176,1.,1.95796111148177));
#26866=CARTESIAN_POINT('Ctrl Pts',(0.479349583074855,1.,1.96294933055943));
#26867=CARTESIAN_POINT('Ctrl Pts',(0.48290166212069,1.,1.96792703422362));
#26868=CARTESIAN_POINT('Ctrl Pts',(0.486502692907658,1.,1.97289186263272));
#26869=CARTESIAN_POINT('Ctrl Pts',(0.490150627860952,1.,1.97783973019229));
#26870=CARTESIAN_POINT('Ctrl Pts',(0.493843476541494,1.,1.98276658761821));
#26871=CARTESIAN_POINT('Ctrl Pts',(0.497579909545574,1.,1.98767044752932));
#26872=CARTESIAN_POINT('Ctrl Pts',(0.501359287727146,1.,1.99255149126155));
#26873=CARTESIAN_POINT('Ctrl Pts',(0.505181361323026,1.,1.99741107463572));
#26874=CARTESIAN_POINT('Ctrl Pts',(0.509046069886157,1.,2.00225107134734));
#26875=CARTESIAN_POINT('Ctrl Pts',(0.512953306961792,1.,2.00707309946949));
#26876=CARTESIAN_POINT('Ctrl Pts',(0.516902681728687,1.,2.01187773939242));
#26877=CARTESIAN_POINT('Ctrl Pts',(0.52089359039937,1.,2.01666477917286));
#26878=CARTESIAN_POINT('Ctrl Pts',(0.524925318333476,1.,2.02143356304698));
#26879=CARTESIAN_POINT('Ctrl Pts',(0.528997127241914,1.,2.0261832908329));
#26880=CARTESIAN_POINT('Ctrl Pts',(0.533108355132976,1.,2.03091336214426));
#26881=CARTESIAN_POINT('Ctrl Pts',(0.537258489833262,1.,2.03562362954037));
#26882=CARTESIAN_POINT('Ctrl Pts',(0.541447120615659,1.,2.04031422690527));
#26883=CARTESIAN_POINT('Ctrl Pts',(0.54567390381743,1.,2.04498544714588));
#26884=CARTESIAN_POINT('Ctrl Pts',(0.549938525150295,1.,2.04963761077958));
#26885=CARTESIAN_POINT('Ctrl Pts',(0.554240657463906,1.,2.05427091604413));
#26886=CARTESIAN_POINT('Ctrl Pts',(0.558579940185151,1.,2.05888537756462));
#26887=CARTESIAN_POINT('Ctrl Pts',(0.562955993082261,1.,2.06348090160589));
#26888=CARTESIAN_POINT('Ctrl Pts',(0.567368421181087,1.,2.06805732997334));
#26889=CARTESIAN_POINT('Ctrl Pts',(0.571816823242602,1.,2.07261449292824));
#26890=CARTESIAN_POINT('Ctrl Pts',(0.576300797416844,1.,2.07715226767559));
#26891=CARTESIAN_POINT('Ctrl Pts',(0.580819952108063,1.,2.08167059018418));
#26892=CARTESIAN_POINT('Ctrl Pts',(0.585373918991617,1.,2.08616943727951));
#26893=CARTESIAN_POINT('Ctrl Pts',(0.589962365403406,1.,2.09064881812129));
#26894=CARTESIAN_POINT('Ctrl Pts',(0.594585006052162,1.,2.0951087622027));
#26895=CARTESIAN_POINT('Ctrl Pts',(0.599241616420533,1.,2.0995493086477));
#26896=CARTESIAN_POINT('Ctrl Pts',(0.60393203073603,1.,2.10397049886949));
#26897=CARTESIAN_POINT('Ctrl Pts',(0.607711315454876,1.,2.1074919961518));
#26898=CARTESIAN_POINT('Ctrl Pts',(0.610560911689898,1.,2.11012443807238));
#26899=CARTESIAN_POINT('Ctrl Pts',(0.6124673655618,1.,2.11187554259986));
#26900=CARTESIAN_POINT('Ctrl Pts',(0.61342227326009,1.,2.11275013067528));
#26901=CARTESIAN_POINT('',(0.383122945602003,0.,1.7075470150345));
#26902=CARTESIAN_POINT('Origin',(0.,0.,0.));
#26903=CARTESIAN_POINT('',(0.163289472382896,1.,1.74236521665491));
#26904=CARTESIAN_POINT('Origin',(0.,1.,0.));
#26905=CARTESIAN_POINT('',(0.163289472382896,0.,1.74236521665491));
#26906=CARTESIAN_POINT('Ctrl Pts',(0.0694764450219578,-1.,2.19890268624765));
#26907=CARTESIAN_POINT('Ctrl Pts',(0.0694764450219578,1.,2.19890268624765));
#26908=CARTESIAN_POINT('Ctrl Pts',(0.0701143536325487,-1.,2.19777582085423));
#26909=CARTESIAN_POINT('Ctrl Pts',(0.0701143536325487,1.,2.19777582085423));
#26910=CARTESIAN_POINT('Ctrl Pts',(0.0713863779526151,-1.,2.19552129484002));
#26911=CARTESIAN_POINT('Ctrl Pts',(0.0713863779526151,1.,2.19552129484002));
#26912=CARTESIAN_POINT('Ctrl Pts',(0.0732830357306722,-1.,2.19213712013662));
#26913=CARTESIAN_POINT('Ctrl Pts',(0.0732830357306722,1.,2.19213712013662));
#26914=CARTESIAN_POINT('Ctrl Pts',(0.0757891465836145,-1.,2.1876201139953));
#26915=CARTESIAN_POINT('Ctrl Pts',(0.0757891465836145,1.,2.1876201139953));
#26916=CARTESIAN_POINT('Ctrl Pts',(0.078883772768524,-1.,2.18196589448887));
#26917=CARTESIAN_POINT('Ctrl Pts',(0.078883772768524,1.,2.18196589448887));
#26918=CARTESIAN_POINT('Ctrl Pts',(0.0819402680872763,-1.,2.176303712113));
#26919=CARTESIAN_POINT('Ctrl Pts',(0.0819402680872763,1.,2.176303712113));
#26920=CARTESIAN_POINT('Ctrl Pts',(0.084958462083537,-1.,2.17063357870952));
#26921=CARTESIAN_POINT('Ctrl Pts',(0.084958462083537,1.,2.17063357870952));
#26922=CARTESIAN_POINT('Ctrl Pts',(0.087938129138692,-1.,2.16495552645014));
#26923=CARTESIAN_POINT('Ctrl Pts',(0.087938129138692,1.,2.16495552645014));
#26924=CARTESIAN_POINT('Ctrl Pts',(0.0908789888107263,-1.,2.15926961544516));
#26925=CARTESIAN_POINT('Ctrl Pts',(0.0908789888107263,1.,2.15926961544516));
#26926=CARTESIAN_POINT('Ctrl Pts',(0.0937807218867641,-1.,2.1535759397817));
#26927=CARTESIAN_POINT('Ctrl Pts',(0.0937807218867641,1.,2.1535759397817));
#26928=CARTESIAN_POINT('Ctrl Pts',(0.0966429852305456,-1.,2.14787463531795));
#26929=CARTESIAN_POINT('Ctrl Pts',(0.0966429852305456,1.,2.14787463531795));
#26930=CARTESIAN_POINT('Ctrl Pts',(0.0994654261990913,-1.,2.14216588396025));
#26931=CARTESIAN_POINT('Ctrl Pts',(0.0994654261990913,1.,2.14216588396025));
#26932=CARTESIAN_POINT('Ctrl Pts',(0.1022477005561,-1.,2.13644992667165));
#26933=CARTESIAN_POINT('Ctrl Pts',(0.1022477005561,1.,2.13644992667165));
#26934=CARTESIAN_POINT('Ctrl Pts',(0.104989479152739,-1.,2.13072704887293));
#26935=CARTESIAN_POINT('Ctrl Pts',(0.104989479152739,1.,2.13072704887293));
#26936=CARTESIAN_POINT('Ctrl Pts',(0.10769043523109,-1.,2.12499752307));
#26937=CARTESIAN_POINT('Ctrl Pts',(0.10769043523109,1.,2.12499752307));
#26938=CARTESIAN_POINT('Ctrl Pts',(0.110350236135025,-1.,2.11926155590865));
#26939=CARTESIAN_POINT('Ctrl Pts',(0.110350236135025,1.,2.11926155590865));
#26940=CARTESIAN_POINT('Ctrl Pts',(0.112968534419737,-1.,2.11351924490306));
#26941=CARTESIAN_POINT('Ctrl Pts',(0.112968534419737,1.,2.11351924490306));
#26942=CARTESIAN_POINT('Ctrl Pts',(0.115544957687926,-1.,2.10777050261309));
#26943=CARTESIAN_POINT('Ctrl Pts',(0.115544957687926,1.,2.10777050261309));
#26944=CARTESIAN_POINT('Ctrl Pts',(0.118079107988355,-1.,2.102015121329));
#26945=CARTESIAN_POINT('Ctrl Pts',(0.118079107988355,1.,2.102015121329));
#26946=CARTESIAN_POINT('Ctrl Pts',(0.120570567965122,-1.,2.0962529286773));
#26947=CARTESIAN_POINT('Ctrl Pts',(0.120570567965122,1.,2.0962529286773));
#26948=CARTESIAN_POINT('Ctrl Pts',(0.123018905621083,-1.,2.09048392424825));
#26949=CARTESIAN_POINT('Ctrl Pts',(0.123018905621083,1.,2.09048392424825));
#26950=CARTESIAN_POINT('Ctrl Pts',(0.125423679412061,-1.,2.08470840653643));
#26951=CARTESIAN_POINT('Ctrl Pts',(0.125423679412061,1.,2.08470840653643));
#26952=CARTESIAN_POINT('Ctrl Pts',(0.12778444527612,-1.,2.07892715110987));
#26953=CARTESIAN_POINT('Ctrl Pts',(0.12778444527612,1.,2.07892715110987));
#26954=CARTESIAN_POINT('Ctrl Pts',(0.130100748328403,-1.,2.07314114713063));
#26955=CARTESIAN_POINT('Ctrl Pts',(0.130100748328403,1.,2.07314114713063));
#26956=CARTESIAN_POINT('Ctrl Pts',(0.13237211154771,-1.,2.06735123910326));
#26957=CARTESIAN_POINT('Ctrl Pts',(0.13237211154771,1.,2.06735123910326));
#26958=CARTESIAN_POINT('Ctrl Pts',(0.134598026192106,-1.,2.06155781517842));
#26959=CARTESIAN_POINT('Ctrl Pts',(0.134598026192106,1.,2.06155781517842));
#26960=CARTESIAN_POINT('Ctrl Pts',(0.136777941218043,-1.,2.05576044414264));
#26961=CARTESIAN_POINT('Ctrl Pts',(0.136777941218043,1.,2.05576044414264));
#26962=CARTESIAN_POINT('Ctrl Pts',(0.138911255368966,-1.,2.04995762001328));
#26963=CARTESIAN_POINT('Ctrl Pts',(0.138911255368966,1.,2.04995762001328));
#26964=CARTESIAN_POINT('Ctrl Pts',(0.140997332152546,-1.,2.04414757947916));
#26965=CARTESIAN_POINT('Ctrl Pts',(0.140997332152546,1.,2.04414757947916));
#26966=CARTESIAN_POINT('Ctrl Pts',(0.143035515058208,-1.,2.03832911025912));
#26967=CARTESIAN_POINT('Ctrl Pts',(0.143035515058208,1.,2.03832911025912));
#26968=CARTESIAN_POINT('Ctrl Pts',(0.145025140186057,-1.,2.03250223739942));
#26969=CARTESIAN_POINT('Ctrl Pts',(0.145025140186057,1.,2.03250223739942));
#26970=CARTESIAN_POINT('Ctrl Pts',(0.146965557332583,-1.,2.02666926182017));
#26971=CARTESIAN_POINT('Ctrl Pts',(0.146965557332583,1.,2.02666926182017));
#26972=CARTESIAN_POINT('Ctrl Pts',(0.148856124775337,-1.,2.02083464969894));
#26973=CARTESIAN_POINT('Ctrl Pts',(0.148856124775337,1.,2.02083464969894));
#26974=CARTESIAN_POINT('Ctrl Pts',(0.150696157673078,-1.,2.01500291940238));
#26975=CARTESIAN_POINT('Ctrl Pts',(0.150696157673078,1.,2.01500291940238));
#26976=CARTESIAN_POINT('Ctrl Pts',(0.152484883621449,-1.,2.00917680318424));
#26977=CARTESIAN_POINT('Ctrl Pts',(0.152484883621449,1.,2.00917680318424));
#26978=CARTESIAN_POINT('Ctrl Pts',(0.154221403049722,-1.,2.00335565310543));
#26979=CARTESIAN_POINT('Ctrl Pts',(0.154221403049722,1.,2.00335565310543));
#26980=CARTESIAN_POINT('Ctrl Pts',(0.155904629548783,-1.,1.99753284771497));
#26981=CARTESIAN_POINT('Ctrl Pts',(0.155904629548783,1.,1.99753284771497));
#26982=CARTESIAN_POINT('Ctrl Pts',(0.157533331459227,-1.,1.99169810931908));
#26983=CARTESIAN_POINT('Ctrl Pts',(0.157533331459227,1.,1.99169810931908));
#26984=CARTESIAN_POINT('Ctrl Pts',(0.159106226437299,-1.,1.98584238283292));
#26985=CARTESIAN_POINT('Ctrl Pts',(0.159106226437299,1.,1.98584238283292));
#26986=CARTESIAN_POINT('Ctrl Pts',(0.160622060784611,-1.,1.97996195437559));
#26987=CARTESIAN_POINT('Ctrl Pts',(0.160622060784611,1.,1.97996195437559));
#26988=CARTESIAN_POINT('Ctrl Pts',(0.162079693556288,-1.,1.97406280235188));
#26989=CARTESIAN_POINT('Ctrl Pts',(0.162079693556288,1.,1.97406280235188));
#26990=CARTESIAN_POINT('Ctrl Pts',(0.163478185457734,-1.,1.96816512677967));
#26991=CARTESIAN_POINT('Ctrl Pts',(0.163478185457734,1.,1.96816512677967));
#26992=CARTESIAN_POINT('Ctrl Pts',(0.164816568920269,-1.,1.96229379940136));
#26993=CARTESIAN_POINT('Ctrl Pts',(0.164816568920269,1.,1.96229379940136));
#26994=CARTESIAN_POINT('Ctrl Pts',(0.166093592002812,-1.,1.9564675971873));
#26995=CARTESIAN_POINT('Ctrl Pts',(0.166093592002812,1.,1.9564675971873));
#26996=CARTESIAN_POINT('Ctrl Pts',(0.167307501784475,-1.,1.95069027794294));
#26997=CARTESIAN_POINT('Ctrl Pts',(0.167307501784475,1.,1.95069027794294));
#26998=CARTESIAN_POINT('Ctrl Pts',(0.168455741607556,-1.,1.94493757756931));
#26999=CARTESIAN_POINT('Ctrl Pts',(0.168455741607556,1.,1.94493757756931));
#27000=CARTESIAN_POINT('Ctrl Pts',(0.16953490481749,-1.,1.93915639211581));
#27001=CARTESIAN_POINT('Ctrl Pts',(0.16953490481749,1.,1.93915639211581));
#27002=CARTESIAN_POINT('Ctrl Pts',(0.170541253116201,-1.,1.93329183155539));
#27003=CARTESIAN_POINT('Ctrl Pts',(0.170541253116201,1.,1.93329183155539));
#27004=CARTESIAN_POINT('Ctrl Pts',(0.171471191532988,-1.,1.92731093582036));
#27005=CARTESIAN_POINT('Ctrl Pts',(0.171471191532988,1.,1.92731093582036));
#27006=CARTESIAN_POINT('Ctrl Pts',(0.172321621259513,-1.,1.9212233439798));
#27007=CARTESIAN_POINT('Ctrl Pts',(0.172321621259513,1.,1.9212233439798));
#27008=CARTESIAN_POINT('Ctrl Pts',(0.173090695383496,-1.,1.91511429159527));
#27009=CARTESIAN_POINT('Ctrl Pts',(0.173090695383496,1.,1.91511429159527));
#27010=CARTESIAN_POINT('Ctrl Pts',(0.173776635257816,-1.,1.90911693975267));
#27011=CARTESIAN_POINT('Ctrl Pts',(0.173776635257816,1.,1.90911693975267));
#27012=CARTESIAN_POINT('Ctrl Pts',(0.174375518661085,-1.,1.90335253862834));
#27013=CARTESIAN_POINT('Ctrl Pts',(0.174375518661085,1.,1.90335253862834));
#27014=CARTESIAN_POINT('Ctrl Pts',(0.174879405091263,-1.,1.89788101117132));
#27015=CARTESIAN_POINT('Ctrl Pts',(0.174879405091263,1.,1.89788101117132));
#27016=CARTESIAN_POINT('Ctrl Pts',(0.175274276190844,-1.,1.892646301985));
#27017=CARTESIAN_POINT('Ctrl Pts',(0.175274276190844,1.,1.892646301985));
#27018=CARTESIAN_POINT('Ctrl Pts',(0.175538155840648,-1.,1.88742606273259));
#27019=CARTESIAN_POINT('Ctrl Pts',(0.175538155840648,1.,1.88742606273259));
#27020=CARTESIAN_POINT('Ctrl Pts',(0.175644148889698,-1.,1.88188663145367));
#27021=CARTESIAN_POINT('Ctrl Pts',(0.175644148889698,1.,1.88188663145367));
#27022=CARTESIAN_POINT('Ctrl Pts',(0.175563480746485,-1.,1.87563767773588));
#27023=CARTESIAN_POINT('Ctrl Pts',(0.175563480746485,1.,1.87563767773588));
#27024=CARTESIAN_POINT('Ctrl Pts',(0.175268337590757,-1.,1.86828349694799));
#27025=CARTESIAN_POINT('Ctrl Pts',(0.175268337590757,1.,1.86828349694799));
#27026=CARTESIAN_POINT('Ctrl Pts',(0.17473525927603,-1.,1.85948367088837));
#27027=CARTESIAN_POINT('Ctrl Pts',(0.17473525927603,1.,1.85948367088837));
#27028=CARTESIAN_POINT('Ctrl Pts',(0.173946627587731,-1.,1.8489811319852));
#27029=CARTESIAN_POINT('Ctrl Pts',(0.173946627587731,1.,1.8489811319852));
#27030=CARTESIAN_POINT('Ctrl Pts',(0.1728894428919,-1.,1.83658380527692));
#27031=CARTESIAN_POINT('Ctrl Pts',(0.1728894428919,1.,1.83658380527692));
#27032=CARTESIAN_POINT('Ctrl Pts',(0.171554770204119,-1.,1.82215766811545));
#27033=CARTESIAN_POINT('Ctrl Pts',(0.171554770204119,1.,1.82215766811545));
#27034=CARTESIAN_POINT('Ctrl Pts',(0.169936923904608,-1.,1.80561530629706));
#27035=CARTESIAN_POINT('Ctrl Pts',(0.169936923904608,1.,1.80561530629706));
#27036=CARTESIAN_POINT('Ctrl Pts',(0.168032772805197,-1.,1.7869064998507));
#27037=CARTESIAN_POINT('Ctrl Pts',(0.168032772805197,1.,1.7869064998507));
#27038=CARTESIAN_POINT('Ctrl Pts',(0.1662793551464,-1.,1.77018771684844));
#27039=CARTESIAN_POINT('Ctrl Pts',(0.1662793551464,1.,1.77018771684844));
#27040=CARTESIAN_POINT('Ctrl Pts',(0.164834765707158,-1.,1.75666056638427));
#27041=CARTESIAN_POINT('Ctrl Pts',(0.164834765707158,1.,1.75666056638427));
#27042=CARTESIAN_POINT('Ctrl Pts',(0.163814161002002,-1.,1.7472034950333));
#27043=CARTESIAN_POINT('Ctrl Pts',(0.163814161002002,1.,1.7472034950333));
#27044=CARTESIAN_POINT('Ctrl Pts',(0.163289472382896,-1.,1.74236521665491));
#27045=CARTESIAN_POINT('Ctrl Pts',(0.163289472382896,1.,1.74236521665491));
#27046=CARTESIAN_POINT('',(0.0694764450219578,1.,2.19890268624765));
#27047=CARTESIAN_POINT('Ctrl Pts',(0.0694764450219578,1.,2.19890268624765));
#27048=CARTESIAN_POINT('Ctrl Pts',(0.0701143536325487,1.,2.19777582085423));
#27049=CARTESIAN_POINT('Ctrl Pts',(0.0713863779526151,1.,2.19552129484002));
#27050=CARTESIAN_POINT('Ctrl Pts',(0.0732830357306722,1.,2.19213712013662));
#27051=CARTESIAN_POINT('Ctrl Pts',(0.0757891465836145,1.,2.1876201139953));
#27052=CARTESIAN_POINT('Ctrl Pts',(0.078883772768524,1.,2.18196589448887));
#27053=CARTESIAN_POINT('Ctrl Pts',(0.0819402680872763,1.,2.176303712113));
#27054=CARTESIAN_POINT('Ctrl Pts',(0.084958462083537,1.,2.17063357870952));
#27055=CARTESIAN_POINT('Ctrl Pts',(0.087938129138692,1.,2.16495552645014));
#27056=CARTESIAN_POINT('Ctrl Pts',(0.0908789888107263,1.,2.15926961544516));
#27057=CARTESIAN_POINT('Ctrl Pts',(0.0937807218867641,1.,2.1535759397817));
#27058=CARTESIAN_POINT('Ctrl Pts',(0.0966429852305456,1.,2.14787463531795));
#27059=CARTESIAN_POINT('Ctrl Pts',(0.0994654261990913,1.,2.14216588396025));
#27060=CARTESIAN_POINT('Ctrl Pts',(0.1022477005561,1.,2.13644992667165));
#27061=CARTESIAN_POINT('Ctrl Pts',(0.104989479152739,1.,2.13072704887293));
#27062=CARTESIAN_POINT('Ctrl Pts',(0.10769043523109,1.,2.12499752307));
#27063=CARTESIAN_POINT('Ctrl Pts',(0.110350236135025,1.,2.11926155590865));
#27064=CARTESIAN_POINT('Ctrl Pts',(0.112968534419737,1.,2.11351924490306));
#27065=CARTESIAN_POINT('Ctrl Pts',(0.115544957687926,1.,2.10777050261309));
#27066=CARTESIAN_POINT('Ctrl Pts',(0.118079107988355,1.,2.102015121329));
#27067=CARTESIAN_POINT('Ctrl Pts',(0.120570567965122,1.,2.0962529286773));
#27068=CARTESIAN_POINT('Ctrl Pts',(0.123018905621083,1.,2.09048392424825));
#27069=CARTESIAN_POINT('Ctrl Pts',(0.125423679412061,1.,2.08470840653643));
#27070=CARTESIAN_POINT('Ctrl Pts',(0.12778444527612,1.,2.07892715110987));
#27071=CARTESIAN_POINT('Ctrl Pts',(0.130100748328403,1.,2.07314114713063));
#27072=CARTESIAN_POINT('Ctrl Pts',(0.13237211154771,1.,2.06735123910326));
#27073=CARTESIAN_POINT('Ctrl Pts',(0.134598026192106,1.,2.06155781517842));
#27074=CARTESIAN_POINT('Ctrl Pts',(0.136777941218043,1.,2.05576044414264));
#27075=CARTESIAN_POINT('Ctrl Pts',(0.138911255368966,1.,2.04995762001328));
#27076=CARTESIAN_POINT('Ctrl Pts',(0.140997332152546,1.,2.04414757947916));
#27077=CARTESIAN_POINT('Ctrl Pts',(0.143035515058208,1.,2.03832911025912));
#27078=CARTESIAN_POINT('Ctrl Pts',(0.145025140186057,1.,2.03250223739942));
#27079=CARTESIAN_POINT('Ctrl Pts',(0.146965557332583,1.,2.02666926182017));
#27080=CARTESIAN_POINT('Ctrl Pts',(0.148856124775337,1.,2.02083464969894));
#27081=CARTESIAN_POINT('Ctrl Pts',(0.150696157673078,1.,2.01500291940238));
#27082=CARTESIAN_POINT('Ctrl Pts',(0.152484883621449,1.,2.00917680318424));
#27083=CARTESIAN_POINT('Ctrl Pts',(0.154221403049722,1.,2.00335565310543));
#27084=CARTESIAN_POINT('Ctrl Pts',(0.155904629548783,1.,1.99753284771497));
#27085=CARTESIAN_POINT('Ctrl Pts',(0.157533331459227,1.,1.99169810931908));
#27086=CARTESIAN_POINT('Ctrl Pts',(0.159106226437299,1.,1.98584238283292));
#27087=CARTESIAN_POINT('Ctrl Pts',(0.160622060784611,1.,1.97996195437559));
#27088=CARTESIAN_POINT('Ctrl Pts',(0.162079693556288,1.,1.97406280235188));
#27089=CARTESIAN_POINT('Ctrl Pts',(0.163478185457734,1.,1.96816512677967));
#27090=CARTESIAN_POINT('Ctrl Pts',(0.164816568920269,1.,1.96229379940136));
#27091=CARTESIAN_POINT('Ctrl Pts',(0.166093592002812,1.,1.9564675971873));
#27092=CARTESIAN_POINT('Ctrl Pts',(0.167307501784475,1.,1.95069027794294));
#27093=CARTESIAN_POINT('Ctrl Pts',(0.168455741607556,1.,1.94493757756931));
#27094=CARTESIAN_POINT('Ctrl Pts',(0.16953490481749,1.,1.93915639211581));
#27095=CARTESIAN_POINT('Ctrl Pts',(0.170541253116201,1.,1.93329183155539));
#27096=CARTESIAN_POINT('Ctrl Pts',(0.171471191532988,1.,1.92731093582036));
#27097=CARTESIAN_POINT('Ctrl Pts',(0.172321621259513,1.,1.9212233439798));
#27098=CARTESIAN_POINT('Ctrl Pts',(0.173090695383496,1.,1.91511429159527));
#27099=CARTESIAN_POINT('Ctrl Pts',(0.173776635257816,1.,1.90911693975267));
#27100=CARTESIAN_POINT('Ctrl Pts',(0.174375518661085,1.,1.90335253862834));
#27101=CARTESIAN_POINT('Ctrl Pts',(0.174879405091263,1.,1.89788101117132));
#27102=CARTESIAN_POINT('Ctrl Pts',(0.175274276190844,1.,1.892646301985));
#27103=CARTESIAN_POINT('Ctrl Pts',(0.175538155840648,1.,1.88742606273259));
#27104=CARTESIAN_POINT('Ctrl Pts',(0.175644148889698,1.,1.88188663145367));
#27105=CARTESIAN_POINT('Ctrl Pts',(0.175563480746485,1.,1.87563767773588));
#27106=CARTESIAN_POINT('Ctrl Pts',(0.175268337590757,1.,1.86828349694799));
#27107=CARTESIAN_POINT('Ctrl Pts',(0.17473525927603,1.,1.85948367088837));
#27108=CARTESIAN_POINT('Ctrl Pts',(0.173946627587731,1.,1.8489811319852));
#27109=CARTESIAN_POINT('Ctrl Pts',(0.1728894428919,1.,1.83658380527692));
#27110=CARTESIAN_POINT('Ctrl Pts',(0.171554770204119,1.,1.82215766811545));
#27111=CARTESIAN_POINT('Ctrl Pts',(0.169936923904608,1.,1.80561530629706));
#27112=CARTESIAN_POINT('Ctrl Pts',(0.168032772805197,1.,1.7869064998507));
#27113=CARTESIAN_POINT('Ctrl Pts',(0.1662793551464,1.,1.77018771684844));
#27114=CARTESIAN_POINT('Ctrl Pts',(0.164834765707158,1.,1.75666056638427));
#27115=CARTESIAN_POINT('Ctrl Pts',(0.163814161002002,1.,1.7472034950333));
#27116=CARTESIAN_POINT('Ctrl Pts',(0.163289472382896,1.,1.74236521665491));
#27117=CARTESIAN_POINT('',(0.0694764450219578,0.,2.19890268624765));
#27118=CARTESIAN_POINT('Origin',(-0.0694764450219586,0.,2.19890268624765));
#27119=CARTESIAN_POINT('',(-0.0694764450219586,1.,2.19890268624765));
#27120=CARTESIAN_POINT('',(0.0694764450219578,1.,2.19890268624765));
#27121=CARTESIAN_POINT('',(-0.0694764450219586,0.,2.19890268624765));
#27122=CARTESIAN_POINT('Ctrl Pts',(-0.163289472382896,-1.,1.74236521665491));
#27123=CARTESIAN_POINT('Ctrl Pts',(-0.163289472382896,1.,1.74236521665491));
#27124=CARTESIAN_POINT('Ctrl Pts',(-0.163814161002474,-1.,1.74720349503904));
#27125=CARTESIAN_POINT('Ctrl Pts',(-0.163814161002474,1.,1.74720349503904));
#27126=CARTESIAN_POINT('Ctrl Pts',(-0.164834765708484,-1.,1.75666056640041));
#27127=CARTESIAN_POINT('Ctrl Pts',(-0.164834765708484,1.,1.75666056640041));
#27128=CARTESIAN_POINT('Ctrl Pts',(-0.166279355148738,-1.,1.77018771687692));
#27129=CARTESIAN_POINT('Ctrl Pts',(-0.166279355148738,1.,1.77018771687692));
#27130=CARTESIAN_POINT('Ctrl Pts',(-0.16803277280837,-1.,1.78690649988931));
#27131=CARTESIAN_POINT('Ctrl Pts',(-0.16803277280837,1.,1.78690649988931));
#27132=CARTESIAN_POINT('Ctrl Pts',(-0.169936923908078,-1.,1.80561530633924));
#27133=CARTESIAN_POINT('Ctrl Pts',(-0.169936923908078,1.,1.80561530633924));
#27134=CARTESIAN_POINT('Ctrl Pts',(-0.171554770207306,-1.,1.82215766815414));
#27135=CARTESIAN_POINT('Ctrl Pts',(-0.171554770207306,1.,1.82215766815414));
#27136=CARTESIAN_POINT('Ctrl Pts',(-0.17288944289442,-1.,1.83658380530747));
#27137=CARTESIAN_POINT('Ctrl Pts',(-0.17288944289442,1.,1.83658380530747));
#27138=CARTESIAN_POINT('Ctrl Pts',(-0.173946627589401,-1.,1.84898113200543));
#27139=CARTESIAN_POINT('Ctrl Pts',(-0.173946627589401,1.,1.84898113200543));
#27140=CARTESIAN_POINT('Ctrl Pts',(-0.174735259276856,-1.,1.85948367089838));
#27141=CARTESIAN_POINT('Ctrl Pts',(-0.174735259276856,1.,1.85948367089838));
#27142=CARTESIAN_POINT('Ctrl Pts',(-0.175268337590901,-1.,1.86828349694972));
#27143=CARTESIAN_POINT('Ctrl Pts',(-0.175268337590901,1.,1.86828349694972));
#27144=CARTESIAN_POINT('Ctrl Pts',(-0.175563480746206,-1.,1.87563767773249));
#27145=CARTESIAN_POINT('Ctrl Pts',(-0.175563480746206,1.,1.87563767773249));
#27146=CARTESIAN_POINT('Ctrl Pts',(-0.175644148889271,-1.,1.88188663144846));
#27147=CARTESIAN_POINT('Ctrl Pts',(-0.175644148889271,1.,1.88188663144846));
#27148=CARTESIAN_POINT('Ctrl Pts',(-0.175538155840286,-1.,1.88742606272818));
#27149=CARTESIAN_POINT('Ctrl Pts',(-0.175538155840286,1.,1.88742606272818));
#27150=CARTESIAN_POINT('Ctrl Pts',(-0.175274276190664,-1.,1.89264630198279));
#27151=CARTESIAN_POINT('Ctrl Pts',(-0.175274276190664,1.,1.89264630198279));
#27152=CARTESIAN_POINT('Ctrl Pts',(-0.174879405091277,-1.,1.89788101117148));
#27153=CARTESIAN_POINT('Ctrl Pts',(-0.174879405091277,1.,1.89788101117148));
#27154=CARTESIAN_POINT('Ctrl Pts',(-0.174375518661222,-1.,1.90335253863003));
#27155=CARTESIAN_POINT('Ctrl Pts',(-0.174375518661222,1.,1.90335253863003));
#27156=CARTESIAN_POINT('Ctrl Pts',(-0.173776635257984,-1.,1.90911693975475));
#27157=CARTESIAN_POINT('Ctrl Pts',(-0.173776635257984,1.,1.90911693975475));
#27158=CARTESIAN_POINT('Ctrl Pts',(-0.173090695383619,-1.,1.91511429159681));
#27159=CARTESIAN_POINT('Ctrl Pts',(-0.173090695383619,1.,1.91511429159681));
#27160=CARTESIAN_POINT('Ctrl Pts',(-0.172321621259557,-1.,1.92122334398034));
#27161=CARTESIAN_POINT('Ctrl Pts',(-0.172321621259557,1.,1.92122334398034));
#27162=CARTESIAN_POINT('Ctrl Pts',(-0.17147119153296,-1.,1.92731093582));
#27163=CARTESIAN_POINT('Ctrl Pts',(-0.17147119153296,1.,1.92731093582));
#27164=CARTESIAN_POINT('Ctrl Pts',(-0.170541253116136,-1.,1.93329183155455));
#27165=CARTESIAN_POINT('Ctrl Pts',(-0.170541253116136,1.,1.93329183155455));
#27166=CARTESIAN_POINT('Ctrl Pts',(-0.169534904817425,-1.,1.93915639211497));
#27167=CARTESIAN_POINT('Ctrl Pts',(-0.169534904817425,1.,1.93915639211497));
#27168=CARTESIAN_POINT('Ctrl Pts',(-0.168455741607516,-1.,1.94493757756879));
#27169=CARTESIAN_POINT('Ctrl Pts',(-0.168455741607516,1.,1.94493757756879));
#27170=CARTESIAN_POINT('Ctrl Pts',(-0.167307501784469,-1.,1.95069027794286));
#27171=CARTESIAN_POINT('Ctrl Pts',(-0.167307501784469,1.,1.95069027794286));
#27172=CARTESIAN_POINT('Ctrl Pts',(-0.166093592002833,-1.,1.95646759718755));
#27173=CARTESIAN_POINT('Ctrl Pts',(-0.166093592002833,1.,1.95646759718755));
#27174=CARTESIAN_POINT('Ctrl Pts',(-0.1648165689203,-1.,1.96229379940174));
#27175=CARTESIAN_POINT('Ctrl Pts',(-0.1648165689203,1.,1.96229379940174));
#27176=CARTESIAN_POINT('Ctrl Pts',(-0.16347818545776,-1.,1.96816512678));
#27177=CARTESIAN_POINT('Ctrl Pts',(-0.16347818545776,1.,1.96816512678));
#27178=CARTESIAN_POINT('Ctrl Pts',(-0.162079693556302,-1.,1.97406280235204));
#27179=CARTESIAN_POINT('Ctrl Pts',(-0.162079693556302,1.,1.97406280235204));
#27180=CARTESIAN_POINT('Ctrl Pts',(-0.16062206078461,-1.,1.97996195437557));
#27181=CARTESIAN_POINT('Ctrl Pts',(-0.16062206078461,1.,1.97996195437557));
#27182=CARTESIAN_POINT('Ctrl Pts',(-0.159106226437289,-1.,1.98584238283279));
#27183=CARTESIAN_POINT('Ctrl Pts',(-0.159106226437289,1.,1.98584238283279));
#27184=CARTESIAN_POINT('Ctrl Pts',(-0.157533331459215,-1.,1.99169810931893));
#27185=CARTESIAN_POINT('Ctrl Pts',(-0.157533331459215,1.,1.99169810931893));
#27186=CARTESIAN_POINT('Ctrl Pts',(-0.155904629548775,-1.,1.99753284771487));
#27187=CARTESIAN_POINT('Ctrl Pts',(-0.155904629548775,1.,1.99753284771487));
#27188=CARTESIAN_POINT('Ctrl Pts',(-0.154221403049719,-1.,2.00335565310539));
#27189=CARTESIAN_POINT('Ctrl Pts',(-0.154221403049719,1.,2.00335565310539));
#27190=CARTESIAN_POINT('Ctrl Pts',(-0.152484883621452,-1.,2.00917680318426));
#27191=CARTESIAN_POINT('Ctrl Pts',(-0.152484883621452,1.,2.00917680318426));
#27192=CARTESIAN_POINT('Ctrl Pts',(-0.150696157673084,-1.,2.01500291940243));
#27193=CARTESIAN_POINT('Ctrl Pts',(-0.150696157673084,1.,2.01500291940243));
#27194=CARTESIAN_POINT('Ctrl Pts',(-0.148856124775343,-1.,2.02083464969897));
#27195=CARTESIAN_POINT('Ctrl Pts',(-0.148856124775343,1.,2.02083464969897));
#27196=CARTESIAN_POINT('Ctrl Pts',(-0.146965557332586,-1.,2.02666926182017));
#27197=CARTESIAN_POINT('Ctrl Pts',(-0.146965557332586,1.,2.02666926182017));
#27198=CARTESIAN_POINT('Ctrl Pts',(-0.145025140186058,-1.,2.03250223739941));
#27199=CARTESIAN_POINT('Ctrl Pts',(-0.145025140186058,1.,2.03250223739941));
#27200=CARTESIAN_POINT('Ctrl Pts',(-0.143035515058208,-1.,2.03832911025913));
#27201=CARTESIAN_POINT('Ctrl Pts',(-0.143035515058208,1.,2.03832911025913));
#27202=CARTESIAN_POINT('Ctrl Pts',(-0.140997332152546,-1.,2.04414757947919));
#27203=CARTESIAN_POINT('Ctrl Pts',(-0.140997332152546,1.,2.04414757947919));
#27204=CARTESIAN_POINT('Ctrl Pts',(-0.138911255368966,-1.,2.04995762001333));
#27205=CARTESIAN_POINT('Ctrl Pts',(-0.138911255368966,1.,2.04995762001333));
#27206=CARTESIAN_POINT('Ctrl Pts',(-0.136777941218044,-1.,2.0557604441427));
#27207=CARTESIAN_POINT('Ctrl Pts',(-0.136777941218044,1.,2.0557604441427));
#27208=CARTESIAN_POINT('Ctrl Pts',(-0.134598026192107,-1.,2.06155781517844));
#27209=CARTESIAN_POINT('Ctrl Pts',(-0.134598026192107,1.,2.06155781517844));
#27210=CARTESIAN_POINT('Ctrl Pts',(-0.13237211154771,-1.,2.06735123910319));
#27211=CARTESIAN_POINT('Ctrl Pts',(-0.13237211154771,1.,2.06735123910319));
#27212=CARTESIAN_POINT('Ctrl Pts',(-0.130100748328401,-1.,2.07314114713047));
#27213=CARTESIAN_POINT('Ctrl Pts',(-0.130100748328401,1.,2.07314114713047));
#27214=CARTESIAN_POINT('Ctrl Pts',(-0.127784445276116,-1.,2.07892715110967));
#27215=CARTESIAN_POINT('Ctrl Pts',(-0.127784445276116,1.,2.07892715110967));
#27216=CARTESIAN_POINT('Ctrl Pts',(-0.125423679412058,-1.,2.08470840653628));
#27217=CARTESIAN_POINT('Ctrl Pts',(-0.125423679412058,1.,2.08470840653628));
#27218=CARTESIAN_POINT('Ctrl Pts',(-0.123018905621083,-1.,2.09048392424826));
#27219=CARTESIAN_POINT('Ctrl Pts',(-0.123018905621083,1.,2.09048392424826));
#27220=CARTESIAN_POINT('Ctrl Pts',(-0.120570567965129,-1.,2.09625292867756));
#27221=CARTESIAN_POINT('Ctrl Pts',(-0.120570567965129,1.,2.09625292867756));
#27222=CARTESIAN_POINT('Ctrl Pts',(-0.118079107988368,-1.,2.10201512132945));
#27223=CARTESIAN_POINT('Ctrl Pts',(-0.118079107988368,1.,2.10201512132945));
#27224=CARTESIAN_POINT('Ctrl Pts',(-0.115544957687941,-1.,2.10777050261359));
#27225=CARTESIAN_POINT('Ctrl Pts',(-0.115544957687941,1.,2.10777050261359));
#27226=CARTESIAN_POINT('Ctrl Pts',(-0.112968534419746,-1.,2.11351924490335));
#27227=CARTESIAN_POINT('Ctrl Pts',(-0.112968534419746,1.,2.11351924490335));
#27228=CARTESIAN_POINT('Ctrl Pts',(-0.11035023613502,-1.,2.11926155590849));
#27229=CARTESIAN_POINT('Ctrl Pts',(-0.11035023613502,1.,2.11926155590849));
#27230=CARTESIAN_POINT('Ctrl Pts',(-0.107690435231068,-1.,2.12499752306927));
#27231=CARTESIAN_POINT('Ctrl Pts',(-0.107690435231068,1.,2.12499752306927));
#27232=CARTESIAN_POINT('Ctrl Pts',(-0.104989479152703,-1.,2.1307270488718));
#27233=CARTESIAN_POINT('Ctrl Pts',(-0.104989479152703,1.,2.1307270488718));
#27234=CARTESIAN_POINT('Ctrl Pts',(-0.102247700556064,-1.,2.13644992667052));
#27235=CARTESIAN_POINT('Ctrl Pts',(-0.102247700556064,1.,2.13644992667052));
#27236=CARTESIAN_POINT('Ctrl Pts',(-0.0994654261990745,-1.,2.14216588395974));
#27237=CARTESIAN_POINT('Ctrl Pts',(-0.0994654261990745,1.,2.14216588395974));
#27238=CARTESIAN_POINT('Ctrl Pts',(-0.0966429852305691,-1.,2.14787463531864));
#27239=CARTESIAN_POINT('Ctrl Pts',(-0.0966429852305691,1.,2.14787463531864));
#27240=CARTESIAN_POINT('Ctrl Pts',(-0.0937807218868348,-1.,2.15357593978377));
#27241=CARTESIAN_POINT('Ctrl Pts',(-0.0937807218868348,1.,2.15357593978377));
#27242=CARTESIAN_POINT('Ctrl Pts',(-0.0908789888108269,-1.,2.15926961544808));
#27243=CARTESIAN_POINT('Ctrl Pts',(-0.0908789888108269,1.,2.15926961544808));
#27244=CARTESIAN_POINT('Ctrl Pts',(-0.0879381291387825,-1.,2.16495552645275));
#27245=CARTESIAN_POINT('Ctrl Pts',(-0.0879381291387825,1.,2.16495552645275));
#27246=CARTESIAN_POINT('Ctrl Pts',(-0.0849584620835646,-1.,2.17063357871031));
#27247=CARTESIAN_POINT('Ctrl Pts',(-0.0849584620835646,1.,2.17063357871031));
#27248=CARTESIAN_POINT('Ctrl Pts',(-0.0819402680871942,-1.,2.1763037121106));
#27249=CARTESIAN_POINT('Ctrl Pts',(-0.0819402680871942,1.,2.1763037121106));
#27250=CARTESIAN_POINT('Ctrl Pts',(-0.078883772768323,-1.,2.18196589448304));
#27251=CARTESIAN_POINT('Ctrl Pts',(-0.078883772768323,1.,2.18196589448304));
#27252=CARTESIAN_POINT('Ctrl Pts',(-0.0757891465833414,-1.,2.1876201139874));
#27253=CARTESIAN_POINT('Ctrl Pts',(-0.0757891465833414,1.,2.1876201139874));
#27254=CARTESIAN_POINT('Ctrl Pts',(-0.0732830357304279,-1.,2.19213712012956));
#27255=CARTESIAN_POINT('Ctrl Pts',(-0.0732830357304279,1.,2.19213712012956));
#27256=CARTESIAN_POINT('Ctrl Pts',(-0.071386377952463,-1.,2.19552129483562));
#27257=CARTESIAN_POINT('Ctrl Pts',(-0.071386377952463,1.,2.19552129483562));
#27258=CARTESIAN_POINT('Ctrl Pts',(-0.0701143536324929,-1.,2.19777582085261));
#27259=CARTESIAN_POINT('Ctrl Pts',(-0.0701143536324929,1.,2.19777582085261));
#27260=CARTESIAN_POINT('Ctrl Pts',(-0.0694764450219586,-1.,2.19890268624765));
#27261=CARTESIAN_POINT('Ctrl Pts',(-0.0694764450219586,1.,2.19890268624765));
#27262=CARTESIAN_POINT('',(-0.163289472382896,1.,1.74236521665491));
#27263=CARTESIAN_POINT('Ctrl Pts',(-0.163289472382896,1.,1.74236521665491));
#27264=CARTESIAN_POINT('Ctrl Pts',(-0.163814161002474,1.,1.74720349503904));
#27265=CARTESIAN_POINT('Ctrl Pts',(-0.164834765708484,1.,1.75666056640041));
#27266=CARTESIAN_POINT('Ctrl Pts',(-0.166279355148738,1.,1.77018771687692));
#27267=CARTESIAN_POINT('Ctrl Pts',(-0.16803277280837,1.,1.78690649988931));
#27268=CARTESIAN_POINT('Ctrl Pts',(-0.169936923908078,1.,1.80561530633924));
#27269=CARTESIAN_POINT('Ctrl Pts',(-0.171554770207306,1.,1.82215766815414));
#27270=CARTESIAN_POINT('Ctrl Pts',(-0.17288944289442,1.,1.83658380530747));
#27271=CARTESIAN_POINT('Ctrl Pts',(-0.173946627589401,1.,1.84898113200543));
#27272=CARTESIAN_POINT('Ctrl Pts',(-0.174735259276856,1.,1.85948367089838));
#27273=CARTESIAN_POINT('Ctrl Pts',(-0.175268337590901,1.,1.86828349694972));
#27274=CARTESIAN_POINT('Ctrl Pts',(-0.175563480746206,1.,1.87563767773249));
#27275=CARTESIAN_POINT('Ctrl Pts',(-0.175644148889271,1.,1.88188663144846));
#27276=CARTESIAN_POINT('Ctrl Pts',(-0.175538155840286,1.,1.88742606272818));
#27277=CARTESIAN_POINT('Ctrl Pts',(-0.175274276190664,1.,1.89264630198279));
#27278=CARTESIAN_POINT('Ctrl Pts',(-0.174879405091277,1.,1.89788101117148));
#27279=CARTESIAN_POINT('Ctrl Pts',(-0.174375518661222,1.,1.90335253863003));
#27280=CARTESIAN_POINT('Ctrl Pts',(-0.173776635257984,1.,1.90911693975475));
#27281=CARTESIAN_POINT('Ctrl Pts',(-0.173090695383619,1.,1.91511429159681));
#27282=CARTESIAN_POINT('Ctrl Pts',(-0.172321621259557,1.,1.92122334398034));
#27283=CARTESIAN_POINT('Ctrl Pts',(-0.17147119153296,1.,1.92731093582));
#27284=CARTESIAN_POINT('Ctrl Pts',(-0.170541253116136,1.,1.93329183155455));
#27285=CARTESIAN_POINT('Ctrl Pts',(-0.169534904817425,1.,1.93915639211497));
#27286=CARTESIAN_POINT('Ctrl Pts',(-0.168455741607516,1.,1.94493757756879));
#27287=CARTESIAN_POINT('Ctrl Pts',(-0.167307501784469,1.,1.95069027794286));
#27288=CARTESIAN_POINT('Ctrl Pts',(-0.166093592002833,1.,1.95646759718755));
#27289=CARTESIAN_POINT('Ctrl Pts',(-0.1648165689203,1.,1.96229379940174));
#27290=CARTESIAN_POINT('Ctrl Pts',(-0.16347818545776,1.,1.96816512678));
#27291=CARTESIAN_POINT('Ctrl Pts',(-0.162079693556302,1.,1.97406280235204));
#27292=CARTESIAN_POINT('Ctrl Pts',(-0.16062206078461,1.,1.97996195437557));
#27293=CARTESIAN_POINT('Ctrl Pts',(-0.159106226437289,1.,1.98584238283279));
#27294=CARTESIAN_POINT('Ctrl Pts',(-0.157533331459215,1.,1.99169810931893));
#27295=CARTESIAN_POINT('Ctrl Pts',(-0.155904629548775,1.,1.99753284771487));
#27296=CARTESIAN_POINT('Ctrl Pts',(-0.154221403049719,1.,2.00335565310539));
#27297=CARTESIAN_POINT('Ctrl Pts',(-0.152484883621452,1.,2.00917680318426));
#27298=CARTESIAN_POINT('Ctrl Pts',(-0.150696157673084,1.,2.01500291940243));
#27299=CARTESIAN_POINT('Ctrl Pts',(-0.148856124775343,1.,2.02083464969897));
#27300=CARTESIAN_POINT('Ctrl Pts',(-0.146965557332586,1.,2.02666926182017));
#27301=CARTESIAN_POINT('Ctrl Pts',(-0.145025140186058,1.,2.03250223739941));
#27302=CARTESIAN_POINT('Ctrl Pts',(-0.143035515058208,1.,2.03832911025913));
#27303=CARTESIAN_POINT('Ctrl Pts',(-0.140997332152546,1.,2.04414757947919));
#27304=CARTESIAN_POINT('Ctrl Pts',(-0.138911255368966,1.,2.04995762001333));
#27305=CARTESIAN_POINT('Ctrl Pts',(-0.136777941218044,1.,2.0557604441427));
#27306=CARTESIAN_POINT('Ctrl Pts',(-0.134598026192107,1.,2.06155781517844));
#27307=CARTESIAN_POINT('Ctrl Pts',(-0.13237211154771,1.,2.06735123910319));
#27308=CARTESIAN_POINT('Ctrl Pts',(-0.130100748328401,1.,2.07314114713047));
#27309=CARTESIAN_POINT('Ctrl Pts',(-0.127784445276116,1.,2.07892715110967));
#27310=CARTESIAN_POINT('Ctrl Pts',(-0.125423679412058,1.,2.08470840653628));
#27311=CARTESIAN_POINT('Ctrl Pts',(-0.123018905621083,1.,2.09048392424826));
#27312=CARTESIAN_POINT('Ctrl Pts',(-0.120570567965129,1.,2.09625292867756));
#27313=CARTESIAN_POINT('Ctrl Pts',(-0.118079107988368,1.,2.10201512132945));
#27314=CARTESIAN_POINT('Ctrl Pts',(-0.115544957687941,1.,2.10777050261359));
#27315=CARTESIAN_POINT('Ctrl Pts',(-0.112968534419746,1.,2.11351924490335));
#27316=CARTESIAN_POINT('Ctrl Pts',(-0.11035023613502,1.,2.11926155590849));
#27317=CARTESIAN_POINT('Ctrl Pts',(-0.107690435231068,1.,2.12499752306927));
#27318=CARTESIAN_POINT('Ctrl Pts',(-0.104989479152703,1.,2.1307270488718));
#27319=CARTESIAN_POINT('Ctrl Pts',(-0.102247700556064,1.,2.13644992667052));
#27320=CARTESIAN_POINT('Ctrl Pts',(-0.0994654261990745,1.,2.14216588395974));
#27321=CARTESIAN_POINT('Ctrl Pts',(-0.0966429852305691,1.,2.14787463531864));
#27322=CARTESIAN_POINT('Ctrl Pts',(-0.0937807218868348,1.,2.15357593978377));
#27323=CARTESIAN_POINT('Ctrl Pts',(-0.0908789888108269,1.,2.15926961544808));
#27324=CARTESIAN_POINT('Ctrl Pts',(-0.0879381291387825,1.,2.16495552645275));
#27325=CARTESIAN_POINT('Ctrl Pts',(-0.0849584620835646,1.,2.17063357871031));
#27326=CARTESIAN_POINT('Ctrl Pts',(-0.0819402680871942,1.,2.1763037121106));
#27327=CARTESIAN_POINT('Ctrl Pts',(-0.078883772768323,1.,2.18196589448304));
#27328=CARTESIAN_POINT('Ctrl Pts',(-0.0757891465833414,1.,2.1876201139874));
#27329=CARTESIAN_POINT('Ctrl Pts',(-0.0732830357304279,1.,2.19213712012956));
#27330=CARTESIAN_POINT('Ctrl Pts',(-0.071386377952463,1.,2.19552129483562));
#27331=CARTESIAN_POINT('Ctrl Pts',(-0.0701143536324929,1.,2.19777582085261));
#27332=CARTESIAN_POINT('Ctrl Pts',(-0.0694764450219586,1.,2.19890268624765));
#27333=CARTESIAN_POINT('',(-0.163289472382897,0.,1.74236521665491));
#27334=CARTESIAN_POINT('Origin',(0.,0.,0.));
#27335=CARTESIAN_POINT('',(-0.383122945602004,1.,1.7075470150345));
#27336=CARTESIAN_POINT('Origin',(0.,1.,0.));
#27337=CARTESIAN_POINT('',(-0.383122945602004,0.,1.7075470150345));
#27338=CARTESIAN_POINT('Ctrl Pts',(-0.61342227326009,-1.,2.11275013067528));
#27339=CARTESIAN_POINT('Ctrl Pts',(-0.61342227326009,1.,2.11275013067528));
#27340=CARTESIAN_POINT('Ctrl Pts',(-0.61246736556225,-1.,2.11187554260142));
#27341=CARTESIAN_POINT('Ctrl Pts',(-0.61246736556225,1.,2.11187554260142));
#27342=CARTESIAN_POINT('Ctrl Pts',(-0.610560911691113,-1.,2.11012443807661));
#27343=CARTESIAN_POINT('Ctrl Pts',(-0.610560911691113,1.,2.11012443807661));
#27344=CARTESIAN_POINT('Ctrl Pts',(-0.607711315456826,-1.,2.10749199615859));
#27345=CARTESIAN_POINT('Ctrl Pts',(-0.607711315456826,1.,2.10749199615859));
#27346=CARTESIAN_POINT('Ctrl Pts',(-0.603932030738212,-1.,2.10397049887709));
#27347=CARTESIAN_POINT('Ctrl Pts',(-0.603932030738212,1.,2.10397049887709));
#27348=CARTESIAN_POINT('Ctrl Pts',(-0.599241616422144,-1.,2.09954930865331));
#27349=CARTESIAN_POINT('Ctrl Pts',(-0.599241616422144,1.,2.09954930865331));
#27350=CARTESIAN_POINT('Ctrl Pts',(-0.594585006052824,-1.,2.09510876220501));
#27351=CARTESIAN_POINT('Ctrl Pts',(-0.594585006052824,1.,2.09510876220501));
#27352=CARTESIAN_POINT('Ctrl Pts',(-0.589962365403189,-1.,2.09064881812053));
#27353=CARTESIAN_POINT('Ctrl Pts',(-0.589962365403189,1.,2.09064881812053));
#27354=CARTESIAN_POINT('Ctrl Pts',(-0.585373918990895,-1.,2.086169437277));
#27355=CARTESIAN_POINT('Ctrl Pts',(-0.585373918990895,1.,2.086169437277));
#27356=CARTESIAN_POINT('Ctrl Pts',(-0.580819952107257,-1.,2.08167059018138));
#27357=CARTESIAN_POINT('Ctrl Pts',(-0.580819952107257,1.,2.08167059018138));
#27358=CARTESIAN_POINT('Ctrl Pts',(-0.576300797416275,-1.,2.07715226767361));
#27359=CARTESIAN_POINT('Ctrl Pts',(-0.576300797416275,1.,2.07715226767361));
#27360=CARTESIAN_POINT('Ctrl Pts',(-0.571816823242411,-1.,2.07261449292757));
#27361=CARTESIAN_POINT('Ctrl Pts',(-0.571816823242411,1.,2.07261449292757));
#27362=CARTESIAN_POINT('Ctrl Pts',(-0.567368421181229,-1.,2.06805732997383));
#27363=CARTESIAN_POINT('Ctrl Pts',(-0.567368421181229,1.,2.06805732997383));
#27364=CARTESIAN_POINT('Ctrl Pts',(-0.562955993082574,-1.,2.06348090160697));
#27365=CARTESIAN_POINT('Ctrl Pts',(-0.562955993082574,1.,2.06348090160697));
#27366=CARTESIAN_POINT('Ctrl Pts',(-0.558579940185467,-1.,2.05888537756571));
#27367=CARTESIAN_POINT('Ctrl Pts',(-0.558579940185467,1.,2.05888537756571));
#27368=CARTESIAN_POINT('Ctrl Pts',(-0.55424065746411,-1.,2.05427091604482));
#27369=CARTESIAN_POINT('Ctrl Pts',(-0.55424065746411,1.,2.05427091604482));
#27370=CARTESIAN_POINT('Ctrl Pts',(-0.549938525150342,-1.,2.04963761077974));
#27371=CARTESIAN_POINT('Ctrl Pts',(-0.549938525150342,1.,2.04963761077974));
#27372=CARTESIAN_POINT('Ctrl Pts',(-0.545673903817348,-1.,2.0449854471456));
#27373=CARTESIAN_POINT('Ctrl Pts',(-0.545673903817348,1.,2.0449854471456));
#27374=CARTESIAN_POINT('Ctrl Pts',(-0.54144712061552,-1.,2.0403142269048));
#27375=CARTESIAN_POINT('Ctrl Pts',(-0.54144712061552,1.,2.0403142269048));
#27376=CARTESIAN_POINT('Ctrl Pts',(-0.537258489833134,-1.,2.03562362953993));
#27377=CARTESIAN_POINT('Ctrl Pts',(-0.537258489833134,1.,2.03562362953993));
#27378=CARTESIAN_POINT('Ctrl Pts',(-0.533108355132905,-1.,2.03091336214401));
#27379=CARTESIAN_POINT('Ctrl Pts',(-0.533108355132905,1.,2.03091336214401));
#27380=CARTESIAN_POINT('Ctrl Pts',(-0.528997127241911,-1.,2.02618329083289));
#27381=CARTESIAN_POINT('Ctrl Pts',(-0.528997127241911,1.,2.02618329083289));
#27382=CARTESIAN_POINT('Ctrl Pts',(-0.524925318333518,-1.,2.02143356304712));
#27383=CARTESIAN_POINT('Ctrl Pts',(-0.524925318333518,1.,2.02143356304712));
#27384=CARTESIAN_POINT('Ctrl Pts',(-0.520893590399428,-1.,2.01666477917305));
#27385=CARTESIAN_POINT('Ctrl Pts',(-0.520893590399428,1.,2.01666477917305));
#27386=CARTESIAN_POINT('Ctrl Pts',(-0.516902681728733,-1.,2.01187773939257));
#27387=CARTESIAN_POINT('Ctrl Pts',(-0.516902681728733,1.,2.01187773939257));
#27388=CARTESIAN_POINT('Ctrl Pts',(-0.512953306961814,-1.,2.00707309946955));
#27389=CARTESIAN_POINT('Ctrl Pts',(-0.512953306961814,1.,2.00707309946955));
#27390=CARTESIAN_POINT('Ctrl Pts',(-0.509046069886152,-1.,2.00225107134733));
#27391=CARTESIAN_POINT('Ctrl Pts',(-0.509046069886152,1.,2.00225107134733));
#27392=CARTESIAN_POINT('Ctrl Pts',(-0.505181361323011,-1.,1.99741107463567));
#27393=CARTESIAN_POINT('Ctrl Pts',(-0.505181361323011,1.,1.99741107463567));
#27394=CARTESIAN_POINT('Ctrl Pts',(-0.501359287727129,-1.,1.9925514912615));
#27395=CARTESIAN_POINT('Ctrl Pts',(-0.501359287727129,1.,1.9925514912615));
#27396=CARTESIAN_POINT('Ctrl Pts',(-0.497579909545564,-1.,1.98767044752929));
#27397=CARTESIAN_POINT('Ctrl Pts',(-0.497579909545564,1.,1.98767044752929));
#27398=CARTESIAN_POINT('Ctrl Pts',(-0.493843476541492,-1.,1.9827665876182));
#27399=CARTESIAN_POINT('Ctrl Pts',(-0.493843476541492,1.,1.9827665876182));
#27400=CARTESIAN_POINT('Ctrl Pts',(-0.490150627860955,-1.,1.97783973019229));
#27401=CARTESIAN_POINT('Ctrl Pts',(-0.490150627860955,1.,1.97783973019229));
#27402=CARTESIAN_POINT('Ctrl Pts',(-0.486502692907661,-1.,1.97289186263272));
#27403=CARTESIAN_POINT('Ctrl Pts',(-0.486502692907661,1.,1.97289186263272));
#27404=CARTESIAN_POINT('Ctrl Pts',(-0.482901662120687,-1.,1.96792703422358));
#27405=CARTESIAN_POINT('Ctrl Pts',(-0.482901662120687,1.,1.96792703422358));
#27406=CARTESIAN_POINT('Ctrl Pts',(-0.479349583074846,-1.,1.96294933055938));
#27407=CARTESIAN_POINT('Ctrl Pts',(-0.479349583074846,1.,1.96294933055938));
#27408=CARTESIAN_POINT('Ctrl Pts',(-0.475848034683172,-1.,1.95796111148175));
#27409=CARTESIAN_POINT('Ctrl Pts',(-0.475848034683172,1.,1.95796111148175));
#27410=CARTESIAN_POINT('Ctrl Pts',(-0.47239767226408,-1.,1.95296148278136));
#27411=CARTESIAN_POINT('Ctrl Pts',(-0.47239767226408,1.,1.95296148278136));
#27412=CARTESIAN_POINT('Ctrl Pts',(-0.468997482913158,-1.,1.94794381136524));
#27413=CARTESIAN_POINT('Ctrl Pts',(-0.468997482913158,1.,1.94794381136524));
#27414=CARTESIAN_POINT('Ctrl Pts',(-0.465645462026065,-1.,1.94289794196205));
#27415=CARTESIAN_POINT('Ctrl Pts',(-0.465645462026065,1.,1.94289794196205));
#27416=CARTESIAN_POINT('Ctrl Pts',(-0.462340031009087,-1.,1.93781486640834));
#27417=CARTESIAN_POINT('Ctrl Pts',(-0.462340031009087,1.,1.93781486640834));
#27418=CARTESIAN_POINT('Ctrl Pts',(-0.459081234547931,-1.,1.93269066517936));
#27419=CARTESIAN_POINT('Ctrl Pts',(-0.459081234547931,1.,1.93269066517936));
#27420=CARTESIAN_POINT('Ctrl Pts',(-0.455872005174335,-1.,1.92753067150461));
#27421=CARTESIAN_POINT('Ctrl Pts',(-0.455872005174335,1.,1.92753067150461));
#27422=CARTESIAN_POINT('Ctrl Pts',(-0.452719478359356,-1.,1.9223538064847));
#27423=CARTESIAN_POINT('Ctrl Pts',(-0.452719478359356,1.,1.9223538064847));
#27424=CARTESIAN_POINT('Ctrl Pts',(-0.449632260106572,-1.,1.91718342555717));
#27425=CARTESIAN_POINT('Ctrl Pts',(-0.449632260106572,1.,1.91718342555717));
#27426=CARTESIAN_POINT('Ctrl Pts',(-0.446617343485651,-1.,1.91203699981095));
#27427=CARTESIAN_POINT('Ctrl Pts',(-0.446617343485651,1.,1.91203699981095));
#27428=CARTESIAN_POINT('Ctrl Pts',(-0.44367755684917,-1.,1.90691756144906));
#27429=CARTESIAN_POINT('Ctrl Pts',(-0.44367755684917,1.,1.90691756144906));
#27430=CARTESIAN_POINT('Ctrl Pts',(-0.440807833704161,-1.,1.90180124389137));
#27431=CARTESIAN_POINT('Ctrl Pts',(-0.440807833704161,1.,1.90180124389137));
#27432=CARTESIAN_POINT('Ctrl Pts',(-0.437995003948443,-1.,1.89663648956549));
#27433=CARTESIAN_POINT('Ctrl Pts',(-0.437995003948443,1.,1.89663648956549));
#27434=CARTESIAN_POINT('Ctrl Pts',(-0.43522566096358,-1.,1.89136993975585));
#27435=CARTESIAN_POINT('Ctrl Pts',(-0.43522566096358,1.,1.89136993975585));
#27436=CARTESIAN_POINT('Ctrl Pts',(-0.432493038548833,-1.,1.88596913666828));
#27437=CARTESIAN_POINT('Ctrl Pts',(-0.432493038548833,1.,1.88596913666828));
#27438=CARTESIAN_POINT('Ctrl Pts',(-0.429803062482217,-1.,1.88044229001778));
#27439=CARTESIAN_POINT('Ctrl Pts',(-0.429803062482217,1.,1.88044229001778));
#27440=CARTESIAN_POINT('Ctrl Pts',(-0.427183828518743,-1.,1.87486989291333));
#27441=CARTESIAN_POINT('Ctrl Pts',(-0.427183828518743,1.,1.87486989291333));
#27442=CARTESIAN_POINT('Ctrl Pts',(-0.424678177290876,-1.,1.8693780394412));
#27443=CARTESIAN_POINT('Ctrl Pts',(-0.424678177290876,1.,1.8693780394412));
#27444=CARTESIAN_POINT('Ctrl Pts',(-0.422327307417885,-1.,1.86408083333863));
#27445=CARTESIAN_POINT('Ctrl Pts',(-0.422327307417885,1.,1.86408083333863));
#27446=CARTESIAN_POINT('Ctrl Pts',(-0.420157287975583,-1.,1.8590328109667));
#27447=CARTESIAN_POINT('Ctrl Pts',(-0.420157287975583,1.,1.8590328109667));
#27448=CARTESIAN_POINT('Ctrl Pts',(-0.418164129144045,-1.,1.8541763285645));
#27449=CARTESIAN_POINT('Ctrl Pts',(-0.418164129144045,1.,1.8541763285645));
#27450=CARTESIAN_POINT('Ctrl Pts',(-0.416300022039885,-1.,1.84929312930314));
#27451=CARTESIAN_POINT('Ctrl Pts',(-0.416300022039885,1.,1.84929312930314));
#27452=CARTESIAN_POINT('Ctrl Pts',(-0.414487438255542,-1.,1.84405757074218));
#27453=CARTESIAN_POINT('Ctrl Pts',(-0.414487438255542,1.,1.84405757074218));
#27454=CARTESIAN_POINT('Ctrl Pts',(-0.412633125322945,-1.,1.8380895347617));
#27455=CARTESIAN_POINT('Ctrl Pts',(-0.412633125322945,1.,1.8380895347617));
#27456=CARTESIAN_POINT('Ctrl Pts',(-0.410641256301276,-1.,1.83100408895047));
#27457=CARTESIAN_POINT('Ctrl Pts',(-0.410641256301276,1.,1.83100408895047));
#27458=CARTESIAN_POINT('Ctrl Pts',(-0.408428948106227,-1.,1.82247022677562));
#27459=CARTESIAN_POINT('Ctrl Pts',(-0.408428948106227,1.,1.82247022677562));
#27460=CARTESIAN_POINT('Ctrl Pts',(-0.405933518407175,-1.,1.81223801812013));
#27461=CARTESIAN_POINT('Ctrl Pts',(-0.405933518407175,1.,1.81223801812013));
#27462=CARTESIAN_POINT('Ctrl Pts',(-0.403107976163396,-1.,1.80012077173238));
#27463=CARTESIAN_POINT('Ctrl Pts',(-0.403107976163396,1.,1.80012077173238));
#27464=CARTESIAN_POINT('Ctrl Pts',(-0.399919403774155,-1.,1.78598826343754));
#27465=CARTESIAN_POINT('Ctrl Pts',(-0.399919403774155,1.,1.78598826343754));
#27466=CARTESIAN_POINT('Ctrl Pts',(-0.396346196110688,-1.,1.76975560043442));
#27467=CARTESIAN_POINT('Ctrl Pts',(-0.396346196110688,1.,1.76975560043442));
#27468=CARTESIAN_POINT('Ctrl Pts',(-0.392375812285395,-1.,1.75137405310193));
#27469=CARTESIAN_POINT('Ctrl Pts',(-0.392375812285395,1.,1.75137405310193));
#27470=CARTESIAN_POINT('Ctrl Pts',(-0.388877023502615,-1.,1.73493170972829));
#27471=CARTESIAN_POINT('Ctrl Pts',(-0.388877023502615,1.,1.73493170972829));
#27472=CARTESIAN_POINT('Ctrl Pts',(-0.386070790323281,-1.,1.72162022244582));
#27473=CARTESIAN_POINT('Ctrl Pts',(-0.386070790323281,1.,1.72162022244582));
#27474=CARTESIAN_POINT('Ctrl Pts',(-0.384119047314215,-1.,1.71231062891398));
#27475=CARTESIAN_POINT('Ctrl Pts',(-0.384119047314215,1.,1.71231062891398));
#27476=CARTESIAN_POINT('Ctrl Pts',(-0.383122945602004,-1.,1.7075470150345));
#27477=CARTESIAN_POINT('Ctrl Pts',(-0.383122945602004,1.,1.7075470150345));
#27478=CARTESIAN_POINT('',(-0.61342227326009,1.,2.11275013067528));
#27479=CARTESIAN_POINT('Ctrl Pts',(-0.61342227326009,1.,2.11275013067528));
#27480=CARTESIAN_POINT('Ctrl Pts',(-0.61246736556225,1.,2.11187554260142));
#27481=CARTESIAN_POINT('Ctrl Pts',(-0.610560911691113,1.,2.11012443807661));
#27482=CARTESIAN_POINT('Ctrl Pts',(-0.607711315456826,1.,2.10749199615859));
#27483=CARTESIAN_POINT('Ctrl Pts',(-0.603932030738212,1.,2.10397049887709));
#27484=CARTESIAN_POINT('Ctrl Pts',(-0.599241616422144,1.,2.09954930865331));
#27485=CARTESIAN_POINT('Ctrl Pts',(-0.594585006052824,1.,2.09510876220501));
#27486=CARTESIAN_POINT('Ctrl Pts',(-0.589962365403189,1.,2.09064881812053));
#27487=CARTESIAN_POINT('Ctrl Pts',(-0.585373918990895,1.,2.086169437277));
#27488=CARTESIAN_POINT('Ctrl Pts',(-0.580819952107257,1.,2.08167059018138));
#27489=CARTESIAN_POINT('Ctrl Pts',(-0.576300797416275,1.,2.07715226767361));
#27490=CARTESIAN_POINT('Ctrl Pts',(-0.571816823242411,1.,2.07261449292757));
#27491=CARTESIAN_POINT('Ctrl Pts',(-0.567368421181229,1.,2.06805732997383));
#27492=CARTESIAN_POINT('Ctrl Pts',(-0.562955993082574,1.,2.06348090160697));
#27493=CARTESIAN_POINT('Ctrl Pts',(-0.558579940185467,1.,2.05888537756571));
#27494=CARTESIAN_POINT('Ctrl Pts',(-0.55424065746411,1.,2.05427091604482));
#27495=CARTESIAN_POINT('Ctrl Pts',(-0.549938525150342,1.,2.04963761077974));
#27496=CARTESIAN_POINT('Ctrl Pts',(-0.545673903817348,1.,2.0449854471456));
#27497=CARTESIAN_POINT('Ctrl Pts',(-0.54144712061552,1.,2.0403142269048));
#27498=CARTESIAN_POINT('Ctrl Pts',(-0.537258489833134,1.,2.03562362953993));
#27499=CARTESIAN_POINT('Ctrl Pts',(-0.533108355132905,1.,2.03091336214401));
#27500=CARTESIAN_POINT('Ctrl Pts',(-0.528997127241911,1.,2.02618329083289));
#27501=CARTESIAN_POINT('Ctrl Pts',(-0.524925318333518,1.,2.02143356304712));
#27502=CARTESIAN_POINT('Ctrl Pts',(-0.520893590399428,1.,2.01666477917305));
#27503=CARTESIAN_POINT('Ctrl Pts',(-0.516902681728733,1.,2.01187773939257));
#27504=CARTESIAN_POINT('Ctrl Pts',(-0.512953306961814,1.,2.00707309946955));
#27505=CARTESIAN_POINT('Ctrl Pts',(-0.509046069886152,1.,2.00225107134733));
#27506=CARTESIAN_POINT('Ctrl Pts',(-0.505181361323011,1.,1.99741107463567));
#27507=CARTESIAN_POINT('Ctrl Pts',(-0.501359287727129,1.,1.9925514912615));
#27508=CARTESIAN_POINT('Ctrl Pts',(-0.497579909545564,1.,1.98767044752929));
#27509=CARTESIAN_POINT('Ctrl Pts',(-0.493843476541492,1.,1.9827665876182));
#27510=CARTESIAN_POINT('Ctrl Pts',(-0.490150627860955,1.,1.97783973019229));
#27511=CARTESIAN_POINT('Ctrl Pts',(-0.486502692907661,1.,1.97289186263272));
#27512=CARTESIAN_POINT('Ctrl Pts',(-0.482901662120687,1.,1.96792703422358));
#27513=CARTESIAN_POINT('Ctrl Pts',(-0.479349583074846,1.,1.96294933055938));
#27514=CARTESIAN_POINT('Ctrl Pts',(-0.475848034683172,1.,1.95796111148175));
#27515=CARTESIAN_POINT('Ctrl Pts',(-0.47239767226408,1.,1.95296148278136));
#27516=CARTESIAN_POINT('Ctrl Pts',(-0.468997482913158,1.,1.94794381136524));
#27517=CARTESIAN_POINT('Ctrl Pts',(-0.465645462026065,1.,1.94289794196205));
#27518=CARTESIAN_POINT('Ctrl Pts',(-0.462340031009087,1.,1.93781486640834));
#27519=CARTESIAN_POINT('Ctrl Pts',(-0.459081234547931,1.,1.93269066517936));
#27520=CARTESIAN_POINT('Ctrl Pts',(-0.455872005174335,1.,1.92753067150461));
#27521=CARTESIAN_POINT('Ctrl Pts',(-0.452719478359356,1.,1.9223538064847));
#27522=CARTESIAN_POINT('Ctrl Pts',(-0.449632260106572,1.,1.91718342555717));
#27523=CARTESIAN_POINT('Ctrl Pts',(-0.446617343485651,1.,1.91203699981095));
#27524=CARTESIAN_POINT('Ctrl Pts',(-0.44367755684917,1.,1.90691756144906));
#27525=CARTESIAN_POINT('Ctrl Pts',(-0.440807833704161,1.,1.90180124389137));
#27526=CARTESIAN_POINT('Ctrl Pts',(-0.437995003948443,1.,1.89663648956549));
#27527=CARTESIAN_POINT('Ctrl Pts',(-0.43522566096358,1.,1.89136993975585));
#27528=CARTESIAN_POINT('Ctrl Pts',(-0.432493038548833,1.,1.88596913666828));
#27529=CARTESIAN_POINT('Ctrl Pts',(-0.429803062482217,1.,1.88044229001778));
#27530=CARTESIAN_POINT('Ctrl Pts',(-0.427183828518743,1.,1.87486989291333));
#27531=CARTESIAN_POINT('Ctrl Pts',(-0.424678177290876,1.,1.8693780394412));
#27532=CARTESIAN_POINT('Ctrl Pts',(-0.422327307417885,1.,1.86408083333863));
#27533=CARTESIAN_POINT('Ctrl Pts',(-0.420157287975583,1.,1.8590328109667));
#27534=CARTESIAN_POINT('Ctrl Pts',(-0.418164129144045,1.,1.8541763285645));
#27535=CARTESIAN_POINT('Ctrl Pts',(-0.416300022039885,1.,1.84929312930314));
#27536=CARTESIAN_POINT('Ctrl Pts',(-0.414487438255542,1.,1.84405757074218));
#27537=CARTESIAN_POINT('Ctrl Pts',(-0.412633125322945,1.,1.8380895347617));
#27538=CARTESIAN_POINT('Ctrl Pts',(-0.410641256301276,1.,1.83100408895047));
#27539=CARTESIAN_POINT('Ctrl Pts',(-0.408428948106227,1.,1.82247022677562));
#27540=CARTESIAN_POINT('Ctrl Pts',(-0.405933518407175,1.,1.81223801812013));
#27541=CARTESIAN_POINT('Ctrl Pts',(-0.403107976163396,1.,1.80012077173238));
#27542=CARTESIAN_POINT('Ctrl Pts',(-0.399919403774155,1.,1.78598826343754));
#27543=CARTESIAN_POINT('Ctrl Pts',(-0.396346196110688,1.,1.76975560043442));
#27544=CARTESIAN_POINT('Ctrl Pts',(-0.392375812285395,1.,1.75137405310193));
#27545=CARTESIAN_POINT('Ctrl Pts',(-0.388877023502615,1.,1.73493170972829));
#27546=CARTESIAN_POINT('Ctrl Pts',(-0.386070790323281,1.,1.72162022244582));
#27547=CARTESIAN_POINT('Ctrl Pts',(-0.384119047314215,1.,1.71231062891398));
#27548=CARTESIAN_POINT('Ctrl Pts',(-0.383122945602004,1.,1.7075470150345));
#27549=CARTESIAN_POINT('',(-0.61342227326009,0.,2.11275013067528));
#27550=CARTESIAN_POINT('Origin',(-0.745574324794401,0.,2.0698113262342));
#27551=CARTESIAN_POINT('',(-0.745574324794401,1.,2.0698113262342));
#27552=CARTESIAN_POINT('',(-0.61342227326009,1.,2.11275013067528));
#27553=CARTESIAN_POINT('',(-0.745574324794401,0.,2.0698113262342));
#27554=CARTESIAN_POINT('Ctrl Pts',(-0.693717979106306,-1.,1.60662857109684));
#27555=CARTESIAN_POINT('Ctrl Pts',(-0.693717979106306,1.,1.60662857109684));
#27556=CARTESIAN_POINT('Ctrl Pts',(-0.695712097881194,-1.,1.61106790958151));
#27557=CARTESIAN_POINT('Ctrl Pts',(-0.695712097881194,1.,1.61106790958151));
#27558=CARTESIAN_POINT('Ctrl Pts',(-0.699605146405088,-1.,1.61974673472612));
#27559=CARTESIAN_POINT('Ctrl Pts',(-0.699605146405088,1.,1.61974673472612));
#27560=CARTESIAN_POINT('Ctrl Pts',(-0.705159151988319,-1.,1.63216541664676));
#27561=CARTESIAN_POINT('Ctrl Pts',(-0.705159151988319,1.,1.63216541664676));
#27562=CARTESIAN_POINT('Ctrl Pts',(-0.711993139355394,-1.,1.64752408832016));
#27563=CARTESIAN_POINT('Ctrl Pts',(-0.711993139355394,1.,1.64752408832016));
#27564=CARTESIAN_POINT('Ctrl Pts',(-0.719585433804282,-1.,1.6647288055568));
#27565=CARTESIAN_POINT('Ctrl Pts',(-0.719585433804282,1.,1.6647288055568));
#27566=CARTESIAN_POINT('Ctrl Pts',(-0.726235967997433,-1.,1.67996158455503));
#27567=CARTESIAN_POINT('Ctrl Pts',(-0.726235967997433,1.,1.67996158455503));
#27568=CARTESIAN_POINT('Ctrl Pts',(-0.731963238697195,-1.,1.69326921975743));
#27569=CARTESIAN_POINT('Ctrl Pts',(-0.731963238697195,1.,1.69326921975743));
#27570=CARTESIAN_POINT('Ctrl Pts',(-0.736799665724771,-1.,1.70473309006121));
#27571=CARTESIAN_POINT('Ctrl Pts',(-0.736799665724771,1.,1.70473309006121));
#27572=CARTESIAN_POINT('Ctrl Pts',(-0.740795162032088,-1.,1.71447789751927));
#27573=CARTESIAN_POINT('Ctrl Pts',(-0.740795162032088,1.,1.71447789751927));
#27574=CARTESIAN_POINT('Ctrl Pts',(-0.744021445433764,-1.,1.7226822991693));
#27575=CARTESIAN_POINT('Ctrl Pts',(-0.744021445433764,1.,1.7226822991693));
#27576=CARTESIAN_POINT('Ctrl Pts',(-0.746574710096436,-1.,1.72958533647399));
#27577=CARTESIAN_POINT('Ctrl Pts',(-0.746574710096436,1.,1.72958533647399));
#27578=CARTESIAN_POINT('Ctrl Pts',(-0.748582462954855,-1.,1.73550351679848));
#27579=CARTESIAN_POINT('Ctrl Pts',(-0.748582462954855,1.,1.73550351679848));
#27580=CARTESIAN_POINT('Ctrl Pts',(-0.75019343597954,-1.,1.74080458266705));
#27581=CARTESIAN_POINT('Ctrl Pts',(-0.75019343597954,1.,1.74080458266705));
#27582=CARTESIAN_POINT('Ctrl Pts',(-0.751555614163629,-1.,1.74585086852298));
#27583=CARTESIAN_POINT('Ctrl Pts',(-0.751555614163629,1.,1.74585086852298));
#27584=CARTESIAN_POINT('Ctrl Pts',(-0.752797683531377,-1.,1.75095139468809));
#27585=CARTESIAN_POINT('Ctrl Pts',(-0.752797683531377,1.,1.75095139468809));
#27586=CARTESIAN_POINT('Ctrl Pts',(-0.75400925402848,-1.,1.75631083600175));
#27587=CARTESIAN_POINT('Ctrl Pts',(-0.75400925402848,1.,1.75631083600175));
#27588=CARTESIAN_POINT('Ctrl Pts',(-0.755220979975262,-1.,1.7619781724032));
#27589=CARTESIAN_POINT('Ctrl Pts',(-0.755220979975262,1.,1.7619781724032));
#27590=CARTESIAN_POINT('Ctrl Pts',(-0.756421896028403,-1.,1.76789396003141));
#27591=CARTESIAN_POINT('Ctrl Pts',(-0.756421896028403,1.,1.76789396003141));
#27592=CARTESIAN_POINT('Ctrl Pts',(-0.757578264077238,-1.,1.77394167108342));
#27593=CARTESIAN_POINT('Ctrl Pts',(-0.757578264077238,1.,1.77394167108342));
#27594=CARTESIAN_POINT('Ctrl Pts',(-0.75865062667738,-1.,1.77999411220912));
#27595=CARTESIAN_POINT('Ctrl Pts',(-0.75865062667738,1.,1.77999411220912));
#27596=CARTESIAN_POINT('Ctrl Pts',(-0.759614401109868,-1.,1.78596964884526));
#27597=CARTESIAN_POINT('Ctrl Pts',(-0.759614401109868,1.,1.78596964884526));
#27598=CARTESIAN_POINT('Ctrl Pts',(-0.760469555880425,-1.,1.79185815610802));
#27599=CARTESIAN_POINT('Ctrl Pts',(-0.760469555880425,1.,1.79185815610802));
#27600=CARTESIAN_POINT('Ctrl Pts',(-0.761229695230359,-1.,1.79768986997735));
#27601=CARTESIAN_POINT('Ctrl Pts',(-0.761229695230359,1.,1.79768986997735));
#27602=CARTESIAN_POINT('Ctrl Pts',(-0.761915336443516,-1.,1.80351583877334));
#27603=CARTESIAN_POINT('Ctrl Pts',(-0.761915336443516,1.,1.80351583877334));
#27604=CARTESIAN_POINT('Ctrl Pts',(-0.762546129464036,-1.,1.80938551463989));
#27605=CARTESIAN_POINT('Ctrl Pts',(-0.762546129464036,1.,1.80938551463989));
#27606=CARTESIAN_POINT('Ctrl Pts',(-0.763132003836783,-1.,1.81532118405566));
#27607=CARTESIAN_POINT('Ctrl Pts',(-0.763132003836783,1.,1.81532118405566));
#27608=CARTESIAN_POINT('Ctrl Pts',(-0.763673465462854,-1.,1.82131873145297));
#27609=CARTESIAN_POINT('Ctrl Pts',(-0.763673465462854,1.,1.82131873145297));
#27610=CARTESIAN_POINT('Ctrl Pts',(-0.764165902606055,-1.,1.8273599120008));
#27611=CARTESIAN_POINT('Ctrl Pts',(-0.764165902606055,1.,1.8273599120008));
#27612=CARTESIAN_POINT('Ctrl Pts',(-0.764602549687845,-1.,1.8334207722714));
#27613=CARTESIAN_POINT('Ctrl Pts',(-0.764602549687845,1.,1.8334207722714));
#27614=CARTESIAN_POINT('Ctrl Pts',(-0.764978057881687,-1.,1.83948181064823));
#27615=CARTESIAN_POINT('Ctrl Pts',(-0.764978057881687,1.,1.83948181064823));
#27616=CARTESIAN_POINT('Ctrl Pts',(-0.765291664861971,-1.,1.8455369887591));
#27617=CARTESIAN_POINT('Ctrl Pts',(-0.765291664861971,1.,1.8455369887591));
#27618=CARTESIAN_POINT('Ctrl Pts',(-0.765545710619023,-1.,1.85158945130054));
#27619=CARTESIAN_POINT('Ctrl Pts',(-0.765545710619023,1.,1.85158945130054));
#27620=CARTESIAN_POINT('Ctrl Pts',(-0.765744212909305,-1.,1.85764741390391));
#27621=CARTESIAN_POINT('Ctrl Pts',(-0.765744212909305,1.,1.85764741390391));
#27622=CARTESIAN_POINT('Ctrl Pts',(-0.765891519092557,-1.,1.86372027063314));
#27623=CARTESIAN_POINT('Ctrl Pts',(-0.765891519092557,1.,1.86372027063314));
#27624=CARTESIAN_POINT('Ctrl Pts',(-0.765990708546111,-1.,1.86981398314345));
#27625=CARTESIAN_POINT('Ctrl Pts',(-0.765990708546111,1.,1.86981398314345));
#27626=CARTESIAN_POINT('Ctrl Pts',(-0.766042837036759,-1.,1.87592888967886));
#27627=CARTESIAN_POINT('Ctrl Pts',(-0.766042837036759,1.,1.87592888967886));
#27628=CARTESIAN_POINT('Ctrl Pts',(-0.766047794851869,-1.,1.88206215302561));
#27629=CARTESIAN_POINT('Ctrl Pts',(-0.766047794851869,1.,1.88206215302561));
#27630=CARTESIAN_POINT('Ctrl Pts',(-0.76600483706209,-1.,1.88820926433409));
#27631=CARTESIAN_POINT('Ctrl Pts',(-0.76600483706209,1.,1.88820926433409));
#27632=CARTESIAN_POINT('Ctrl Pts',(-0.765913193856979,-1.,1.89436577771389));
#27633=CARTESIAN_POINT('Ctrl Pts',(-0.765913193856979,1.,1.89436577771389));
#27634=CARTESIAN_POINT('Ctrl Pts',(-0.765772772593395,-1.,1.90052930393599));
#27635=CARTESIAN_POINT('Ctrl Pts',(-0.765772772593395,1.,1.90052930393599));
#27636=CARTESIAN_POINT('Ctrl Pts',(-0.765584196937936,-1.,1.90669961402362));
#27637=CARTESIAN_POINT('Ctrl Pts',(-0.765584196937936,1.,1.90669961402362));
#27638=CARTESIAN_POINT('Ctrl Pts',(-0.765348465884739,-1.,1.91287765805174));
#27639=CARTESIAN_POINT('Ctrl Pts',(-0.765348465884739,1.,1.91287765805174));
#27640=CARTESIAN_POINT('Ctrl Pts',(-0.765066729667095,-1.,1.91906491634197));
#27641=CARTESIAN_POINT('Ctrl Pts',(-0.765066729667095,1.,1.91906491634197));
#27642=CARTESIAN_POINT('Ctrl Pts',(-0.764740025488189,-1.,1.92526263537041));
#27643=CARTESIAN_POINT('Ctrl Pts',(-0.764740025488189,1.,1.92526263537041));
#27644=CARTESIAN_POINT('Ctrl Pts',(-0.764369010673889,-1.,1.93147105496367));
#27645=CARTESIAN_POINT('Ctrl Pts',(-0.764369010673889,1.,1.93147105496367));
#27646=CARTESIAN_POINT('Ctrl Pts',(-0.763954049121393,-1.,1.93768964875867));
#27647=CARTESIAN_POINT('Ctrl Pts',(-0.763954049121393,1.,1.93768964875867));
#27648=CARTESIAN_POINT('Ctrl Pts',(-0.76349533353858,-1.,1.94391746617626));
#27649=CARTESIAN_POINT('Ctrl Pts',(-0.76349533353858,1.,1.94391746617626));
#27650=CARTESIAN_POINT('Ctrl Pts',(-0.762992990878774,-1.,1.95015342590025));
#27651=CARTESIAN_POINT('Ctrl Pts',(-0.762992990878774,1.,1.95015342590025));
#27652=CARTESIAN_POINT('Ctrl Pts',(-0.762447203806263,-1.,1.95639665309893));
#27653=CARTESIAN_POINT('Ctrl Pts',(-0.762447203806263,1.,1.95639665309893));
#27654=CARTESIAN_POINT('Ctrl Pts',(-0.761858300014575,-1.,1.96264672744229));
#27655=CARTESIAN_POINT('Ctrl Pts',(-0.761858300014575,1.,1.96264672744229));
#27656=CARTESIAN_POINT('Ctrl Pts',(-0.761226690483986,-1.,1.96890351582545));
#27657=CARTESIAN_POINT('Ctrl Pts',(-0.761226690483986,1.,1.96890351582545));
#27658=CARTESIAN_POINT('Ctrl Pts',(-0.760552825409855,-1.,1.97516705321521));
#27659=CARTESIAN_POINT('Ctrl Pts',(-0.760552825409855,1.,1.97516705321521));
#27660=CARTESIAN_POINT('Ctrl Pts',(-0.759837147452135,-1.,1.98143741418156));
#27661=CARTESIAN_POINT('Ctrl Pts',(-0.759837147452135,1.,1.98143741418156));
#27662=CARTESIAN_POINT('Ctrl Pts',(-0.759080037802243,-1.,1.98771456680806));
#27663=CARTESIAN_POINT('Ctrl Pts',(-0.759080037802243,1.,1.98771456680806));
#27664=CARTESIAN_POINT('Ctrl Pts',(-0.758281796766377,-1.,1.9939983109871));
#27665=CARTESIAN_POINT('Ctrl Pts',(-0.758281796766377,1.,1.9939983109871));
#27666=CARTESIAN_POINT('Ctrl Pts',(-0.757442676862341,-1.,2.00028834739072));
#27667=CARTESIAN_POINT('Ctrl Pts',(-0.757442676862341,1.,2.00028834739072));
#27668=CARTESIAN_POINT('Ctrl Pts',(-0.756562904646496,-1.,2.00658431587682));
#27669=CARTESIAN_POINT('Ctrl Pts',(-0.756562904646496,1.,2.00658431587682));
#27670=CARTESIAN_POINT('Ctrl Pts',(-0.7556427049581,-1.,2.01288584328149));
#27671=CARTESIAN_POINT('Ctrl Pts',(-0.7556427049581,1.,2.01288584328149));
#27672=CARTESIAN_POINT('Ctrl Pts',(-0.75468233072352,-1.,2.01919259406003));
#27673=CARTESIAN_POINT('Ctrl Pts',(-0.75468233072352,1.,2.01919259406003));
#27674=CARTESIAN_POINT('Ctrl Pts',(-0.753682061113766,-1.,2.02550428623587));
#27675=CARTESIAN_POINT('Ctrl Pts',(-0.753682061113766,1.,2.02550428623587));
#27676=CARTESIAN_POINT('Ctrl Pts',(-0.752642180488104,-1.,2.03182068456467));
#27677=CARTESIAN_POINT('Ctrl Pts',(-0.752642180488104,1.,2.03182068456467));
#27678=CARTESIAN_POINT('Ctrl Pts',(-0.751562963361384,-1.,2.03814160092173));
#27679=CARTESIAN_POINT('Ctrl Pts',(-0.751562963361384,1.,2.03814160092173));
#27680=CARTESIAN_POINT('Ctrl Pts',(-0.750444657874758,-1.,2.04446689147754));
#27681=CARTESIAN_POINT('Ctrl Pts',(-0.750444657874758,1.,2.04446689147754));
#27682=CARTESIAN_POINT('Ctrl Pts',(-0.749287468663053,-1.,2.05079645591606));
#27683=CARTESIAN_POINT('Ctrl Pts',(-0.749287468663053,1.,2.05079645591606));
#27684=CARTESIAN_POINT('Ctrl Pts',(-0.748091554181101,-1.,2.05713023030263));
#27685=CARTESIAN_POINT('Ctrl Pts',(-0.748091554181101,1.,2.05713023030263));
#27686=CARTESIAN_POINT('Ctrl Pts',(-0.747103932785504,-1.,2.06220058927162));
#27687=CARTESIAN_POINT('Ctrl Pts',(-0.747103932785504,1.,2.06220058927162));
#27688=CARTESIAN_POINT('Ctrl Pts',(-0.746345871542696,-1.,2.06600523016401));
#27689=CARTESIAN_POINT('Ctrl Pts',(-0.746345871542696,1.,2.06600523016401));
#27690=CARTESIAN_POINT('Ctrl Pts',(-0.74583279137781,-1.,2.06854248895575));
#27691=CARTESIAN_POINT('Ctrl Pts',(-0.74583279137781,1.,2.06854248895575));
#27692=CARTESIAN_POINT('Ctrl Pts',(-0.745574324794401,-1.,2.0698113262342));
#27693=CARTESIAN_POINT('Ctrl Pts',(-0.745574324794401,1.,2.0698113262342));
#27694=CARTESIAN_POINT('',(-0.693717979106306,1.,1.60662857109684));
#27695=CARTESIAN_POINT('Ctrl Pts',(-0.693717979106306,1.,1.60662857109684));
#27696=CARTESIAN_POINT('Ctrl Pts',(-0.695712097881194,1.,1.61106790958151));
#27697=CARTESIAN_POINT('Ctrl Pts',(-0.699605146405088,1.,1.61974673472612));
#27698=CARTESIAN_POINT('Ctrl Pts',(-0.705159151988319,1.,1.63216541664676));
#27699=CARTESIAN_POINT('Ctrl Pts',(-0.711993139355394,1.,1.64752408832016));
#27700=CARTESIAN_POINT('Ctrl Pts',(-0.719585433804282,1.,1.6647288055568));
#27701=CARTESIAN_POINT('Ctrl Pts',(-0.726235967997433,1.,1.67996158455503));
#27702=CARTESIAN_POINT('Ctrl Pts',(-0.731963238697195,1.,1.69326921975743));
#27703=CARTESIAN_POINT('Ctrl Pts',(-0.736799665724771,1.,1.70473309006121));
#27704=CARTESIAN_POINT('Ctrl Pts',(-0.740795162032088,1.,1.71447789751927));
#27705=CARTESIAN_POINT('Ctrl Pts',(-0.744021445433764,1.,1.7226822991693));
#27706=CARTESIAN_POINT('Ctrl Pts',(-0.746574710096436,1.,1.72958533647399));
#27707=CARTESIAN_POINT('Ctrl Pts',(-0.748582462954855,1.,1.73550351679848));
#27708=CARTESIAN_POINT('Ctrl Pts',(-0.75019343597954,1.,1.74080458266705));
#27709=CARTESIAN_POINT('Ctrl Pts',(-0.751555614163629,1.,1.74585086852298));
#27710=CARTESIAN_POINT('Ctrl Pts',(-0.752797683531377,1.,1.75095139468809));
#27711=CARTESIAN_POINT('Ctrl Pts',(-0.75400925402848,1.,1.75631083600175));
#27712=CARTESIAN_POINT('Ctrl Pts',(-0.755220979975262,1.,1.7619781724032));
#27713=CARTESIAN_POINT('Ctrl Pts',(-0.756421896028403,1.,1.76789396003141));
#27714=CARTESIAN_POINT('Ctrl Pts',(-0.757578264077238,1.,1.77394167108342));
#27715=CARTESIAN_POINT('Ctrl Pts',(-0.75865062667738,1.,1.77999411220912));
#27716=CARTESIAN_POINT('Ctrl Pts',(-0.759614401109868,1.,1.78596964884526));
#27717=CARTESIAN_POINT('Ctrl Pts',(-0.760469555880425,1.,1.79185815610802));
#27718=CARTESIAN_POINT('Ctrl Pts',(-0.761229695230359,1.,1.79768986997735));
#27719=CARTESIAN_POINT('Ctrl Pts',(-0.761915336443516,1.,1.80351583877334));
#27720=CARTESIAN_POINT('Ctrl Pts',(-0.762546129464036,1.,1.80938551463989));
#27721=CARTESIAN_POINT('Ctrl Pts',(-0.763132003836783,1.,1.81532118405566));
#27722=CARTESIAN_POINT('Ctrl Pts',(-0.763673465462854,1.,1.82131873145297));
#27723=CARTESIAN_POINT('Ctrl Pts',(-0.764165902606055,1.,1.8273599120008));
#27724=CARTESIAN_POINT('Ctrl Pts',(-0.764602549687845,1.,1.8334207722714));
#27725=CARTESIAN_POINT('Ctrl Pts',(-0.764978057881687,1.,1.83948181064823));
#27726=CARTESIAN_POINT('Ctrl Pts',(-0.765291664861971,1.,1.8455369887591));
#27727=CARTESIAN_POINT('Ctrl Pts',(-0.765545710619023,1.,1.85158945130054));
#27728=CARTESIAN_POINT('Ctrl Pts',(-0.765744212909305,1.,1.85764741390391));
#27729=CARTESIAN_POINT('Ctrl Pts',(-0.765891519092557,1.,1.86372027063314));
#27730=CARTESIAN_POINT('Ctrl Pts',(-0.765990708546111,1.,1.86981398314345));
#27731=CARTESIAN_POINT('Ctrl Pts',(-0.766042837036759,1.,1.87592888967886));
#27732=CARTESIAN_POINT('Ctrl Pts',(-0.766047794851869,1.,1.88206215302561));
#27733=CARTESIAN_POINT('Ctrl Pts',(-0.76600483706209,1.,1.88820926433409));
#27734=CARTESIAN_POINT('Ctrl Pts',(-0.765913193856979,1.,1.89436577771389));
#27735=CARTESIAN_POINT('Ctrl Pts',(-0.765772772593395,1.,1.90052930393599));
#27736=CARTESIAN_POINT('Ctrl Pts',(-0.765584196937936,1.,1.90669961402362));
#27737=CARTESIAN_POINT('Ctrl Pts',(-0.765348465884739,1.,1.91287765805174));
#27738=CARTESIAN_POINT('Ctrl Pts',(-0.765066729667095,1.,1.91906491634197));
#27739=CARTESIAN_POINT('Ctrl Pts',(-0.764740025488189,1.,1.92526263537041));
#27740=CARTESIAN_POINT('Ctrl Pts',(-0.764369010673889,1.,1.93147105496367));
#27741=CARTESIAN_POINT('Ctrl Pts',(-0.763954049121393,1.,1.93768964875867));
#27742=CARTESIAN_POINT('Ctrl Pts',(-0.76349533353858,1.,1.94391746617626));
#27743=CARTESIAN_POINT('Ctrl Pts',(-0.762992990878774,1.,1.95015342590025));
#27744=CARTESIAN_POINT('Ctrl Pts',(-0.762447203806263,1.,1.95639665309893));
#27745=CARTESIAN_POINT('Ctrl Pts',(-0.761858300014575,1.,1.96264672744229));
#27746=CARTESIAN_POINT('Ctrl Pts',(-0.761226690483986,1.,1.96890351582545));
#27747=CARTESIAN_POINT('Ctrl Pts',(-0.760552825409855,1.,1.97516705321521));
#27748=CARTESIAN_POINT('Ctrl Pts',(-0.759837147452135,1.,1.98143741418156));
#27749=CARTESIAN_POINT('Ctrl Pts',(-0.759080037802243,1.,1.98771456680806));
#27750=CARTESIAN_POINT('Ctrl Pts',(-0.758281796766377,1.,1.9939983109871));
#27751=CARTESIAN_POINT('Ctrl Pts',(-0.757442676862341,1.,2.00028834739072));
#27752=CARTESIAN_POINT('Ctrl Pts',(-0.756562904646496,1.,2.00658431587682));
#27753=CARTESIAN_POINT('Ctrl Pts',(-0.7556427049581,1.,2.01288584328149));
#27754=CARTESIAN_POINT('Ctrl Pts',(-0.75468233072352,1.,2.01919259406003));
#27755=CARTESIAN_POINT('Ctrl Pts',(-0.753682061113766,1.,2.02550428623587));
#27756=CARTESIAN_POINT('Ctrl Pts',(-0.752642180488104,1.,2.03182068456467));
#27757=CARTESIAN_POINT('Ctrl Pts',(-0.751562963361384,1.,2.03814160092173));
#27758=CARTESIAN_POINT('Ctrl Pts',(-0.750444657874758,1.,2.04446689147754));
#27759=CARTESIAN_POINT('Ctrl Pts',(-0.749287468663053,1.,2.05079645591606));
#27760=CARTESIAN_POINT('Ctrl Pts',(-0.748091554181101,1.,2.05713023030263));
#27761=CARTESIAN_POINT('Ctrl Pts',(-0.747103932785504,1.,2.06220058927162));
#27762=CARTESIAN_POINT('Ctrl Pts',(-0.746345871542696,1.,2.06600523016401));
#27763=CARTESIAN_POINT('Ctrl Pts',(-0.74583279137781,1.,2.06854248895575));
#27764=CARTESIAN_POINT('Ctrl Pts',(-0.745574324794401,1.,2.0698113262342));
#27765=CARTESIAN_POINT('',(-0.693717979106306,0.,1.60662857109684));
#27766=CARTESIAN_POINT('Origin',(0.,0.,0.));
#27767=CARTESIAN_POINT('',(-0.892032620296855,1.,1.5055822144029));
#27768=CARTESIAN_POINT('Origin',(0.,1.,0.));
#27769=CARTESIAN_POINT('',(-0.892032620296855,0.,1.5055822144029));
#27770=CARTESIAN_POINT('Ctrl Pts',(-1.23627494547115,-1.,1.81978687191668));
#27771=CARTESIAN_POINT('Ctrl Pts',(-1.23627494547115,1.,1.81978687191668));
#27772=CARTESIAN_POINT('Ctrl Pts',(-1.23509651170476,-1.,1.81925017193666));
#27773=CARTESIAN_POINT('Ctrl Pts',(-1.23509651170476,1.,1.81925017193666));
#27774=CARTESIAN_POINT('Ctrl Pts',(-1.2327422452705,-1.,1.81817389921279));
#27775=CARTESIAN_POINT('Ctrl Pts',(-1.2327422452705,1.,1.81817389921279));
#27776=CARTESIAN_POINT('Ctrl Pts',(-1.2292186489137,-1.,1.8165508718364));
#27777=CARTESIAN_POINT('Ctrl Pts',(-1.2292186489137,1.,1.8165508718364));
#27778=CARTESIAN_POINT('Ctrl Pts',(-1.2245361330495,-1.,1.81436959210434));
#27779=CARTESIAN_POINT('Ctrl Pts',(-1.2245361330495,1.,1.81436959210434));
#27780=CARTESIAN_POINT('Ctrl Pts',(-1.21870906103557,-1.,1.81161420806656));
#27781=CARTESIAN_POINT('Ctrl Pts',(-1.21870906103557,1.,1.81161420806656));
#27782=CARTESIAN_POINT('Ctrl Pts',(-1.21290815708314,-1.,1.80882996917129));
#27783=CARTESIAN_POINT('Ctrl Pts',(-1.21290815708314,1.,1.80882996917129));
#27784=CARTESIAN_POINT('Ctrl Pts',(-1.20713356605475,-1.,1.80601678480707));
#27785=CARTESIAN_POINT('Ctrl Pts',(-1.20713356605475,1.,1.80601678480707));
#27786=CARTESIAN_POINT('Ctrl Pts',(-1.20138548938974,-1.,1.80317454838603));
#27787=CARTESIAN_POINT('Ctrl Pts',(-1.20138548938974,1.,1.80317454838603));
#27788=CARTESIAN_POINT('Ctrl Pts',(-1.19566418930242,-1.,1.80030314369879));
#27789=CARTESIAN_POINT('Ctrl Pts',(-1.19566418930242,1.,1.80030314369879));
#27790=CARTESIAN_POINT('Ctrl Pts',(-1.18996997934445,-1.,1.79740245923478));
#27791=CARTESIAN_POINT('Ctrl Pts',(-1.18996997934445,1.,1.79740245923478));
#27792=CARTESIAN_POINT('Ctrl Pts',(-1.18430321697432,-1.,1.79447240321515));
#27793=CARTESIAN_POINT('Ctrl Pts',(-1.18430321697432,1.,1.79447240321515));
#27794=CARTESIAN_POINT('Ctrl Pts',(-1.17866429440809,-1.,1.79151291552689));
#27795=CARTESIAN_POINT('Ctrl Pts',(-1.17866429440809,1.,1.79151291552689));
#27796=CARTESIAN_POINT('Ctrl Pts',(-1.17305363177328,-1.,1.78852398877616));
#27797=CARTESIAN_POINT('Ctrl Pts',(-1.17305363177328,1.,1.78852398877616));
#27798=CARTESIAN_POINT('Ctrl Pts',(-1.16747166312303,-1.,1.78550566040443));
#27799=CARTESIAN_POINT('Ctrl Pts',(-1.16747166312303,1.,1.78550566040443));
#27800=CARTESIAN_POINT('Ctrl Pts',(-1.16191881298499,-1.,1.78245795881009));
#27801=CARTESIAN_POINT('Ctrl Pts',(-1.16191881298499,1.,1.78245795881009));
#27802=CARTESIAN_POINT('Ctrl Pts',(-1.15639547194698,-1.,1.77938085564275));
#27803=CARTESIAN_POINT('Ctrl Pts',(-1.15639547194698,1.,1.77938085564275));
#27804=CARTESIAN_POINT('Ctrl Pts',(-1.15090197841515,-1.,1.7762742255701));
#27805=CARTESIAN_POINT('Ctrl Pts',(-1.15090197841515,1.,1.7762742255701));
#27806=CARTESIAN_POINT('Ctrl Pts',(-1.1454385822692,-1.,1.77313777896194));
#27807=CARTESIAN_POINT('Ctrl Pts',(-1.1454385822692,1.,1.77313777896194));
#27808=CARTESIAN_POINT('Ctrl Pts',(-1.14000548336975,-1.,1.76997111386769));
#27809=CARTESIAN_POINT('Ctrl Pts',(-1.14000548336975,1.,1.76997111386769));
#27810=CARTESIAN_POINT('Ctrl Pts',(-1.1346029180462,-1.,1.76677384551862));
#27811=CARTESIAN_POINT('Ctrl Pts',(-1.1346029180462,1.,1.76677384551862));
#27812=CARTESIAN_POINT('Ctrl Pts',(-1.12923123555075,-1.,1.7635457196617));
#27813=CARTESIAN_POINT('Ctrl Pts',(-1.12923123555075,1.,1.7635457196617));
#27814=CARTESIAN_POINT('Ctrl Pts',(-1.12389096855086,-1.,1.76028671825096));
#27815=CARTESIAN_POINT('Ctrl Pts',(-1.12389096855086,1.,1.76028671825096));
#27816=CARTESIAN_POINT('Ctrl Pts',(-1.11858293216763,-1.,1.75699720772105));
#27817=CARTESIAN_POINT('Ctrl Pts',(-1.11858293216763,1.,1.75699720772105));
#27818=CARTESIAN_POINT('Ctrl Pts',(-1.11330807582551,-1.,1.7536777209463));
#27819=CARTESIAN_POINT('Ctrl Pts',(-1.11330807582551,1.,1.7536777209463));
#27820=CARTESIAN_POINT('Ctrl Pts',(-1.10806728183007,-1.,1.7503286607592));
#27821=CARTESIAN_POINT('Ctrl Pts',(-1.10806728183007,1.,1.7503286607592));
#27822=CARTESIAN_POINT('Ctrl Pts',(-1.10286118991143,-1.,1.74695004214923));
#27823=CARTESIAN_POINT('Ctrl Pts',(-1.10286118991143,1.,1.74695004214923));
#27824=CARTESIAN_POINT('Ctrl Pts',(-1.09768999241225,-1.,1.74354119236208));
#27825=CARTESIAN_POINT('Ctrl Pts',(-1.09768999241225,1.,1.74354119236208));
#27826=CARTESIAN_POINT('Ctrl Pts',(-1.09255329056493,-1.,1.74010053962247));
#27827=CARTESIAN_POINT('Ctrl Pts',(-1.09255329056493,1.,1.74010053962247));
#27828=CARTESIAN_POINT('Ctrl Pts',(-1.08745056285427,-1.,1.73662628326091));
#27829=CARTESIAN_POINT('Ctrl Pts',(-1.08745056285427,1.,1.73662628326091));
#27830=CARTESIAN_POINT('Ctrl Pts',(-1.08238162784749,-1.,1.73311705663407));
#27831=CARTESIAN_POINT('Ctrl Pts',(-1.08238162784749,1.,1.73311705663407));
#27832=CARTESIAN_POINT('Ctrl Pts',(-1.0773470373727,-1.,1.72957248977424));
#27833=CARTESIAN_POINT('Ctrl Pts',(-1.0773470373727,1.,1.72957248977424));
#27834=CARTESIAN_POINT('Ctrl Pts',(-1.07234866990252,-1.,1.72599406198488));
#27835=CARTESIAN_POINT('Ctrl Pts',(-1.07234866990252,1.,1.72599406198488));
#27836=CARTESIAN_POINT('Ctrl Pts',(-1.06738966975462,-1.,1.72238500928453));
#27837=CARTESIAN_POINT('Ctrl Pts',(-1.06738966975462,1.,1.72238500928453));
#27838=CARTESIAN_POINT('Ctrl Pts',(-1.06247324680647,-1.,1.71874858456904));
#27839=CARTESIAN_POINT('Ctrl Pts',(-1.06247324680647,1.,1.71874858456904));
#27840=CARTESIAN_POINT('Ctrl Pts',(-1.05760163192479,-1.,1.7150865442702));
#27841=CARTESIAN_POINT('Ctrl Pts',(-1.05760163192479,1.,1.7150865442702));
#27842=CARTESIAN_POINT('Ctrl Pts',(-1.05277517202855,-1.,1.71139783543989));
#27843=CARTESIAN_POINT('Ctrl Pts',(-1.05277517202855,1.,1.71139783543989));
#27844=CARTESIAN_POINT('Ctrl Pts',(-1.04799085404995,-1.,1.70767646263649));
#27845=CARTESIAN_POINT('Ctrl Pts',(-1.04799085404995,1.,1.70767646263649));
#27846=CARTESIAN_POINT('Ctrl Pts',(-1.04324363334554,-1.,1.70391338707982));
#27847=CARTESIAN_POINT('Ctrl Pts',(-1.04324363334554,1.,1.70391338707982));
#27848=CARTESIAN_POINT('Ctrl Pts',(-1.03852922490789,-1.,1.70010052930962));
#27849=CARTESIAN_POINT('Ctrl Pts',(-1.03852922490789,1.,1.70010052930962));
#27850=CARTESIAN_POINT('Ctrl Pts',(-1.03384646003588,-1.,1.69623414782771));
#27851=CARTESIAN_POINT('Ctrl Pts',(-1.03384646003588,1.,1.69623414782771));
#27852=CARTESIAN_POINT('Ctrl Pts',(-1.02919977579147,-1.,1.69231840863458));
#27853=CARTESIAN_POINT('Ctrl Pts',(-1.02919977579147,1.,1.69231840863458));
#27854=CARTESIAN_POINT('Ctrl Pts',(-1.02460180535255,-1.,1.68836910178447));
#27855=CARTESIAN_POINT('Ctrl Pts',(-1.02460180535255,1.,1.68836910178447));
#27856=CARTESIAN_POINT('Ctrl Pts',(-1.02006795074201,-1.,1.68440578021706));
#27857=CARTESIAN_POINT('Ctrl Pts',(-1.02006795074201,1.,1.68440578021706));
#27858=CARTESIAN_POINT('Ctrl Pts',(-1.01561026162773,-1.,1.68044289894798));
#27859=CARTESIAN_POINT('Ctrl Pts',(-1.01561026162773,1.,1.68044289894798));
#27860=CARTESIAN_POINT('Ctrl Pts',(-1.01123236493511,-1.,1.67648246776464));
#27861=CARTESIAN_POINT('Ctrl Pts',(-1.01123236493511,1.,1.67648246776464));
#27862=CARTESIAN_POINT('Ctrl Pts',(-1.00692206696414,-1.,1.67250335383293));
#27863=CARTESIAN_POINT('Ctrl Pts',(-1.00692206696414,1.,1.67250335383293));
#27864=CARTESIAN_POINT('Ctrl Pts',(-1.00265091003727,-1.,1.66846059277303));
#27865=CARTESIAN_POINT('Ctrl Pts',(-1.00265091003727,1.,1.66846059277303));
#27866=CARTESIAN_POINT('Ctrl Pts',(-0.998389654952758,-1.,1.66430758030376));
#27867=CARTESIAN_POINT('Ctrl Pts',(-0.998389654952758,1.,1.66430758030376));
#27868=CARTESIAN_POINT('Ctrl Pts',(-0.994121836661306,-1.,1.66001553809947));
#27869=CARTESIAN_POINT('Ctrl Pts',(-0.994121836661306,1.,1.66001553809947));
#27870=CARTESIAN_POINT('Ctrl Pts',(-0.989855627854165,-1.,1.65559044289699));
#27871=CARTESIAN_POINT('Ctrl Pts',(-0.989855627854165,1.,1.65559044289699));
#27872=CARTESIAN_POINT('Ctrl Pts',(-0.985642622920821,-1.,1.65110016612638));
#27873=CARTESIAN_POINT('Ctrl Pts',(-0.985642622920821,1.,1.65110016612638));
#27874=CARTESIAN_POINT('Ctrl Pts',(-0.981562530939489,-1.,1.64665139190656));
#27875=CARTESIAN_POINT('Ctrl Pts',(-0.981562530939489,1.,1.64665139190656));
#27876=CARTESIAN_POINT('Ctrl Pts',(-0.977689794119416,-1.,1.64233990826687));
#27877=CARTESIAN_POINT('Ctrl Pts',(-0.977689794119416,1.,1.64233990826687));
#27878=CARTESIAN_POINT('Ctrl Pts',(-0.974066058287418,-1.,1.63820952658144));
#27879=CARTESIAN_POINT('Ctrl Pts',(-0.974066058287418,1.,1.63820952658144));
#27880=CARTESIAN_POINT('Ctrl Pts',(-0.970669715997509,-1.,1.63420665729798));
#27881=CARTESIAN_POINT('Ctrl Pts',(-0.970669715997509,1.,1.63420665729798));
#27882=CARTESIAN_POINT('Ctrl Pts',(-0.967387853230345,-1.,1.63013849959461));
#27883=CARTESIAN_POINT('Ctrl Pts',(-0.967387853230345,1.,1.63013849959461));
#27884=CARTESIAN_POINT('Ctrl Pts',(-0.964046107040536,-1.,1.62571930670187));
#27885=CARTESIAN_POINT('Ctrl Pts',(-0.964046107040536,1.,1.62571930670187));
#27886=CARTESIAN_POINT('Ctrl Pts',(-0.960438326101729,-1.,1.62061638140221));
#27887=CARTESIAN_POINT('Ctrl Pts',(-0.960438326101729,1.,1.62061638140221));
#27888=CARTESIAN_POINT('Ctrl Pts',(-0.956354422920671,-1.,1.61449324337085));
#27889=CARTESIAN_POINT('Ctrl Pts',(-0.956354422920671,1.,1.61449324337085));
#27890=CARTESIAN_POINT('Ctrl Pts',(-0.951613284356035,-1.,1.60706069896936));
#27891=CARTESIAN_POINT('Ctrl Pts',(-0.951613284356035,1.,1.60706069896936));
#27892=CARTESIAN_POINT('Ctrl Pts',(-0.946078063315257,-1.,1.59810042043673));
#27893=CARTESIAN_POINT('Ctrl Pts',(-0.946078063315257,1.,1.59810042043673));
#27894=CARTESIAN_POINT('Ctrl Pts',(-0.939646377893399,-1.,1.58744937487176));
#27895=CARTESIAN_POINT('Ctrl Pts',(-0.939646377893399,1.,1.58744937487176));
#27896=CARTESIAN_POINT('Ctrl Pts',(-0.932246680108685,-1.,1.57499388382243));
#27897=CARTESIAN_POINT('Ctrl Pts',(-0.932246680108685,1.,1.57499388382243));
#27898=CARTESIAN_POINT('Ctrl Pts',(-0.923832188944341,-1.,1.56065988578893));
#27899=CARTESIAN_POINT('Ctrl Pts',(-0.923832188944341,1.,1.56065988578893));
#27900=CARTESIAN_POINT('Ctrl Pts',(-0.914375919026456,-1.,1.54440491149498));
#27901=CARTESIAN_POINT('Ctrl Pts',(-0.914375919026456,1.,1.54440491149498));
#27902=CARTESIAN_POINT('Ctrl Pts',(-0.905967409625651,-1.,1.52984849887993));
#27903=CARTESIAN_POINT('Ctrl Pts',(-0.905967409625651,1.,1.52984849887993));
#27904=CARTESIAN_POINT('Ctrl Pts',(-0.899185047483511,-1.,1.51805569590094));
#27905=CARTESIAN_POINT('Ctrl Pts',(-0.899185047483511,1.,1.51805569590094));
#27906=CARTESIAN_POINT('Ctrl Pts',(-0.894452006964543,-1.,1.50980486806688));
#27907=CARTESIAN_POINT('Ctrl Pts',(-0.894452006964543,1.,1.50980486806688));
#27908=CARTESIAN_POINT('Ctrl Pts',(-0.892032620296855,-1.,1.5055822144029));
#27909=CARTESIAN_POINT('Ctrl Pts',(-0.892032620296855,1.,1.5055822144029));
#27910=CARTESIAN_POINT('',(-1.23627494547115,1.,1.81978687191668));
#27911=CARTESIAN_POINT('Ctrl Pts',(-1.23627494547115,1.,1.81978687191668));
#27912=CARTESIAN_POINT('Ctrl Pts',(-1.23509651170476,1.,1.81925017193666));
#27913=CARTESIAN_POINT('Ctrl Pts',(-1.2327422452705,1.,1.81817389921279));
#27914=CARTESIAN_POINT('Ctrl Pts',(-1.2292186489137,1.,1.8165508718364));
#27915=CARTESIAN_POINT('Ctrl Pts',(-1.2245361330495,1.,1.81436959210434));
#27916=CARTESIAN_POINT('Ctrl Pts',(-1.21870906103557,1.,1.81161420806656));
#27917=CARTESIAN_POINT('Ctrl Pts',(-1.21290815708314,1.,1.80882996917129));
#27918=CARTESIAN_POINT('Ctrl Pts',(-1.20713356605475,1.,1.80601678480707));
#27919=CARTESIAN_POINT('Ctrl Pts',(-1.20138548938974,1.,1.80317454838603));
#27920=CARTESIAN_POINT('Ctrl Pts',(-1.19566418930242,1.,1.80030314369879));
#27921=CARTESIAN_POINT('Ctrl Pts',(-1.18996997934445,1.,1.79740245923478));
#27922=CARTESIAN_POINT('Ctrl Pts',(-1.18430321697432,1.,1.79447240321515));
#27923=CARTESIAN_POINT('Ctrl Pts',(-1.17866429440809,1.,1.79151291552689));
#27924=CARTESIAN_POINT('Ctrl Pts',(-1.17305363177328,1.,1.78852398877616));
#27925=CARTESIAN_POINT('Ctrl Pts',(-1.16747166312303,1.,1.78550566040443));
#27926=CARTESIAN_POINT('Ctrl Pts',(-1.16191881298499,1.,1.78245795881009));
#27927=CARTESIAN_POINT('Ctrl Pts',(-1.15639547194698,1.,1.77938085564275));
#27928=CARTESIAN_POINT('Ctrl Pts',(-1.15090197841515,1.,1.7762742255701));
#27929=CARTESIAN_POINT('Ctrl Pts',(-1.1454385822692,1.,1.77313777896194));
#27930=CARTESIAN_POINT('Ctrl Pts',(-1.14000548336975,1.,1.76997111386769));
#27931=CARTESIAN_POINT('Ctrl Pts',(-1.1346029180462,1.,1.76677384551862));
#27932=CARTESIAN_POINT('Ctrl Pts',(-1.12923123555075,1.,1.7635457196617));
#27933=CARTESIAN_POINT('Ctrl Pts',(-1.12389096855086,1.,1.76028671825096));
#27934=CARTESIAN_POINT('Ctrl Pts',(-1.11858293216763,1.,1.75699720772105));
#27935=CARTESIAN_POINT('Ctrl Pts',(-1.11330807582551,1.,1.7536777209463));
#27936=CARTESIAN_POINT('Ctrl Pts',(-1.10806728183007,1.,1.7503286607592));
#27937=CARTESIAN_POINT('Ctrl Pts',(-1.10286118991143,1.,1.74695004214923));
#27938=CARTESIAN_POINT('Ctrl Pts',(-1.09768999241225,1.,1.74354119236208));
#27939=CARTESIAN_POINT('Ctrl Pts',(-1.09255329056493,1.,1.74010053962247));
#27940=CARTESIAN_POINT('Ctrl Pts',(-1.08745056285427,1.,1.73662628326091));
#27941=CARTESIAN_POINT('Ctrl Pts',(-1.08238162784749,1.,1.73311705663407));
#27942=CARTESIAN_POINT('Ctrl Pts',(-1.0773470373727,1.,1.72957248977424));
#27943=CARTESIAN_POINT('Ctrl Pts',(-1.07234866990252,1.,1.72599406198488));
#27944=CARTESIAN_POINT('Ctrl Pts',(-1.06738966975462,1.,1.72238500928453));
#27945=CARTESIAN_POINT('Ctrl Pts',(-1.06247324680647,1.,1.71874858456904));
#27946=CARTESIAN_POINT('Ctrl Pts',(-1.05760163192479,1.,1.7150865442702));
#27947=CARTESIAN_POINT('Ctrl Pts',(-1.05277517202855,1.,1.71139783543989));
#27948=CARTESIAN_POINT('Ctrl Pts',(-1.04799085404995,1.,1.70767646263649));
#27949=CARTESIAN_POINT('Ctrl Pts',(-1.04324363334554,1.,1.70391338707982));
#27950=CARTESIAN_POINT('Ctrl Pts',(-1.03852922490789,1.,1.70010052930962));
#27951=CARTESIAN_POINT('Ctrl Pts',(-1.03384646003588,1.,1.69623414782771));
#27952=CARTESIAN_POINT('Ctrl Pts',(-1.02919977579147,1.,1.69231840863458));
#27953=CARTESIAN_POINT('Ctrl Pts',(-1.02460180535255,1.,1.68836910178447));
#27954=CARTESIAN_POINT('Ctrl Pts',(-1.02006795074201,1.,1.68440578021706));
#27955=CARTESIAN_POINT('Ctrl Pts',(-1.01561026162773,1.,1.68044289894798));
#27956=CARTESIAN_POINT('Ctrl Pts',(-1.01123236493511,1.,1.67648246776464));
#27957=CARTESIAN_POINT('Ctrl Pts',(-1.00692206696414,1.,1.67250335383293));
#27958=CARTESIAN_POINT('Ctrl Pts',(-1.00265091003727,1.,1.66846059277303));
#27959=CARTESIAN_POINT('Ctrl Pts',(-0.998389654952758,1.,1.66430758030376));
#27960=CARTESIAN_POINT('Ctrl Pts',(-0.994121836661306,1.,1.66001553809947));
#27961=CARTESIAN_POINT('Ctrl Pts',(-0.989855627854165,1.,1.65559044289699));
#27962=CARTESIAN_POINT('Ctrl Pts',(-0.985642622920821,1.,1.65110016612638));
#27963=CARTESIAN_POINT('Ctrl Pts',(-0.981562530939489,1.,1.64665139190656));
#27964=CARTESIAN_POINT('Ctrl Pts',(-0.977689794119416,1.,1.64233990826687));
#27965=CARTESIAN_POINT('Ctrl Pts',(-0.974066058287418,1.,1.63820952658144));
#27966=CARTESIAN_POINT('Ctrl Pts',(-0.970669715997509,1.,1.63420665729798));
#27967=CARTESIAN_POINT('Ctrl Pts',(-0.967387853230345,1.,1.63013849959461));
#27968=CARTESIAN_POINT('Ctrl Pts',(-0.964046107040536,1.,1.62571930670187));
#27969=CARTESIAN_POINT('Ctrl Pts',(-0.960438326101729,1.,1.62061638140221));
#27970=CARTESIAN_POINT('Ctrl Pts',(-0.956354422920671,1.,1.61449324337085));
#27971=CARTESIAN_POINT('Ctrl Pts',(-0.951613284356035,1.,1.60706069896936));
#27972=CARTESIAN_POINT('Ctrl Pts',(-0.946078063315257,1.,1.59810042043673));
#27973=CARTESIAN_POINT('Ctrl Pts',(-0.939646377893399,1.,1.58744937487176));
#27974=CARTESIAN_POINT('Ctrl Pts',(-0.932246680108685,1.,1.57499388382243));
#27975=CARTESIAN_POINT('Ctrl Pts',(-0.923832188944341,1.,1.56065988578893));
#27976=CARTESIAN_POINT('Ctrl Pts',(-0.914375919026456,1.,1.54440491149498));
#27977=CARTESIAN_POINT('Ctrl Pts',(-0.905967409625651,1.,1.52984849887993));
#27978=CARTESIAN_POINT('Ctrl Pts',(-0.899185047483511,1.,1.51805569590094));
#27979=CARTESIAN_POINT('Ctrl Pts',(-0.894452006964543,1.,1.50980486806688));
#27980=CARTESIAN_POINT('Ctrl Pts',(-0.892032620296855,1.,1.5055822144029));
#27981=CARTESIAN_POINT('',(-1.23627494547115,0.,1.81978687191668));
#27982=CARTESIAN_POINT('Origin',(-1.34869019493419,0.,1.73811241238545));
#27983=CARTESIAN_POINT('',(-1.34869019493419,1.,1.73811241238545));
#27984=CARTESIAN_POINT('',(-1.23627494547115,1.,1.81978687191668));
#27985=CARTESIAN_POINT('',(-1.34869019493419,0.,1.73811241238545));
#27986=CARTESIAN_POINT('Ctrl Pts',(-1.15624053661742,-1.,1.31362392696032));
#27987=CARTESIAN_POINT('Ctrl Pts',(-1.15624053661742,1.,1.31362392696032));
#27988=CARTESIAN_POINT('Ctrl Pts',(-1.15950888730809,-1.,1.31722977216397));
#27989=CARTESIAN_POINT('Ctrl Pts',(-1.15950888730809,1.,1.31722977216397));
#27990=CARTESIAN_POINT('Ctrl Pts',(-1.16589330093588,-1.,1.32428080721772));
#27991=CARTESIAN_POINT('Ctrl Pts',(-1.16589330093588,1.,1.32428080721772));
#27992=CARTESIAN_POINT('Ctrl Pts',(-1.17501305789857,-1.,1.33437539347008));
#27993=CARTESIAN_POINT('Ctrl Pts',(-1.17501305789857,1.,1.33437539347008));
#27994=CARTESIAN_POINT('Ctrl Pts',(-1.18625865667441,-1.,1.34687054001093));
#27995=CARTESIAN_POINT('Ctrl Pts',(-1.18625865667441,1.,1.34687054001093));
#27996=CARTESIAN_POINT('Ctrl Pts',(-1.1987959077932,-1.,1.36088705043885));
#27997=CARTESIAN_POINT('Ctrl Pts',(-1.1987959077932,1.,1.36088705043885));
#27998=CARTESIAN_POINT('Ctrl Pts',(-1.20982812925645,-1.,1.37331915607905));
#27999=CARTESIAN_POINT('Ctrl Pts',(-1.20982812925645,1.,1.37331915607905));
#28000=CARTESIAN_POINT('Ctrl Pts',(-1.21938737280852,-1.,1.38420564527715));
#28001=CARTESIAN_POINT('Ctrl Pts',(-1.21938737280852,1.,1.38420564527715));
#28002=CARTESIAN_POINT('Ctrl Pts',(-1.22752961899387,-1.,1.39361389568796));
#28003=CARTESIAN_POINT('Ctrl Pts',(-1.22752961899387,1.,1.39361389568796));
#28004=CARTESIAN_POINT('Ctrl Pts',(-1.23434087290423,-1.,1.40164708206106));
#28005=CARTESIAN_POINT('Ctrl Pts',(-1.23434087290423,1.,1.40164708206106));
#28006=CARTESIAN_POINT('Ctrl Pts',(-1.23994455029534,-1.,1.40845295531283));
#28007=CARTESIAN_POINT('Ctrl Pts',(-1.23994455029534,1.,1.40845295531283));
#28008=CARTESIAN_POINT('Ctrl Pts',(-1.24450600513056,-1.,1.41422913175179));
#28009=CARTESIAN_POINT('Ctrl Pts',(-1.24450600513056,1.,1.41422913175179));
#28010=CARTESIAN_POINT('Ctrl Pts',(-1.24824430986571,-1.,1.41923722596025));
#28011=CARTESIAN_POINT('Ctrl Pts',(-1.24824430986571,1.,1.41923722596025));
#28012=CARTESIAN_POINT('Ctrl Pts',(-1.2514145557001,-1.,1.42378102115575));
#28013=CARTESIAN_POINT('Ctrl Pts',(-1.2514145557001,1.,1.42378102115575));
#28014=CARTESIAN_POINT('Ctrl Pts',(-1.25426945222639,-1.,1.42815938799387));
#28015=CARTESIAN_POINT('Ctrl Pts',(-1.25426945222639,1.,1.42815938799387));
#28016=CARTESIAN_POINT('Ctrl Pts',(-1.25702687965755,-1.,1.43262645609691));
#28017=CARTESIAN_POINT('Ctrl Pts',(-1.25702687965755,1.,1.43262645609691));
#28018=CARTESIAN_POINT('Ctrl Pts',(-1.25983531012005,-1.,1.43734919180848));
#28019=CARTESIAN_POINT('Ctrl Pts',(-1.25983531012005,1.,1.43734919180848));
#28020=CARTESIAN_POINT('Ctrl Pts',(-1.26273903323859,-1.,1.44236470511303));
#28021=CARTESIAN_POINT('Ctrl Pts',(-1.26273903323859,1.,1.44236470511303));
#28022=CARTESIAN_POINT('Ctrl Pts',(-1.26570925118868,-1.,1.44761985001662));
#28023=CARTESIAN_POINT('Ctrl Pts',(-1.26570925118868,1.,1.44761985001662));
#28024=CARTESIAN_POINT('Ctrl Pts',(-1.2686778680489,-1.,1.45301422764247));
#28025=CARTESIAN_POINT('Ctrl Pts',(-1.2686778680489,1.,1.45301422764247));
#28026=CARTESIAN_POINT('Ctrl Pts',(-1.27156805265289,-1.,1.45843906294697));
#28027=CARTESIAN_POINT('Ctrl Pts',(-1.27156805265289,1.,1.45843906294697));
#28028=CARTESIAN_POINT('Ctrl Pts',(-1.27433119897822,-1.,1.46382431332476));
#28029=CARTESIAN_POINT('Ctrl Pts',(-1.27433119897822,1.,1.46382431332476));
#28030=CARTESIAN_POINT('Ctrl Pts',(-1.27696414831089,-1.,1.46916035917133));
#28031=CARTESIAN_POINT('Ctrl Pts',(-1.27696414831089,1.,1.46916035917133));
#28032=CARTESIAN_POINT('Ctrl Pts',(-1.2794891824849,-1.,1.4744717526707));
#28033=CARTESIAN_POINT('Ctrl Pts',(-1.2794891824849,1.,1.4744717526707));
#28034=CARTESIAN_POINT('Ctrl Pts',(-1.28194158939517,-1.,1.47980070347095));
#28035=CARTESIAN_POINT('Ctrl Pts',(-1.28194158939517,1.,1.47980070347095));
#28036=CARTESIAN_POINT('Ctrl Pts',(-1.28435533880201,-1.,1.4851881711891));
#28037=CARTESIAN_POINT('Ctrl Pts',(-1.28435533880201,1.,1.4851881711891));
#28038=CARTESIAN_POINT('Ctrl Pts',(-1.2867467611644,-1.,1.4906522831278));
#28039=CARTESIAN_POINT('Ctrl Pts',(-1.2867467611644,1.,1.4906522831278));
#28040=CARTESIAN_POINT('Ctrl Pts',(-1.28911506584254,-1.,1.49618896881754));
#28041=CARTESIAN_POINT('Ctrl Pts',(-1.28911506584254,1.,1.49618896881754));
#28042=CARTESIAN_POINT('Ctrl Pts',(-1.29145022885181,-1.,1.50178230149776));
#28043=CARTESIAN_POINT('Ctrl Pts',(-1.29145022885181,1.,1.50178230149776));
#28044=CARTESIAN_POINT('Ctrl Pts',(-1.29373841372842,-1.,1.50741159078365));
#28045=CARTESIAN_POINT('Ctrl Pts',(-1.29373841372842,1.,1.50741159078365));
#28046=CARTESIAN_POINT('Ctrl Pts',(-1.29596850710509,-1.,1.51305994241402));
#28047=CARTESIAN_POINT('Ctrl Pts',(-1.29596850710509,1.,1.51305994241402));
#28048=CARTESIAN_POINT('Ctrl Pts',(-1.29813791800747,-1.,1.51872184912724));
#28049=CARTESIAN_POINT('Ctrl Pts',(-1.29813791800747,1.,1.51872184912724));
#28050=CARTESIAN_POINT('Ctrl Pts',(-1.30024984366328,-1.,1.52439957861062));
#28051=CARTESIAN_POINT('Ctrl Pts',(-1.30024984366328,1.,1.52439957861062));
#28052=CARTESIAN_POINT('Ctrl Pts',(-1.30231064395568,-1.,1.53009970283891));
#28053=CARTESIAN_POINT('Ctrl Pts',(-1.30231064395568,1.,1.53009970283891));
#28054=CARTESIAN_POINT('Ctrl Pts',(-1.30432735639489,-1.,1.53582981268977));
#28055=CARTESIAN_POINT('Ctrl Pts',(-1.30432735639489,1.,1.53582981268977));
#28056=CARTESIAN_POINT('Ctrl Pts',(-1.30630475189556,-1.,1.54159462645432));
#28057=CARTESIAN_POINT('Ctrl Pts',(-1.30630475189556,1.,1.54159462645432));
#28058=CARTESIAN_POINT('Ctrl Pts',(-1.30824393907473,-1.,1.54739413957185));
#28059=CARTESIAN_POINT('Ctrl Pts',(-1.30824393907473,1.,1.54739413957185));
#28060=CARTESIAN_POINT('Ctrl Pts',(-1.31014393684222,-1.,1.55322568759481));
#28061=CARTESIAN_POINT('Ctrl Pts',(-1.31014393684222,1.,1.55322568759481));
#28062=CARTESIAN_POINT('Ctrl Pts',(-1.31200264341696,-1.,1.55908521254821));
#28063=CARTESIAN_POINT('Ctrl Pts',(-1.31200264341696,1.,1.55908521254821));
#28064=CARTESIAN_POINT('Ctrl Pts',(-1.31381795281002,-1.,1.56496872402353));
#28065=CARTESIAN_POINT('Ctrl Pts',(-1.31381795281002,1.,1.56496872402353));
#28066=CARTESIAN_POINT('Ctrl Pts',(-1.31558903860016,-1.,1.57087397835723));
#28067=CARTESIAN_POINT('Ctrl Pts',(-1.31558903860016,1.,1.57087397835723));
#28068=CARTESIAN_POINT('Ctrl Pts',(-1.31731642317187,-1.,1.5768005650559));
#28069=CARTESIAN_POINT('Ctrl Pts',(-1.31731642317187,1.,1.5768005650559));
#28070=CARTESIAN_POINT('Ctrl Pts',(-1.31900135021432,-1.,1.58274907898834));
#28071=CARTESIAN_POINT('Ctrl Pts',(-1.31900135021432,1.,1.58274907898834));
#28072=CARTESIAN_POINT('Ctrl Pts',(-1.32064537110892,-1.,1.58872057258245));
#28073=CARTESIAN_POINT('Ctrl Pts',(-1.32064537110892,1.,1.58872057258245));
#28074=CARTESIAN_POINT('Ctrl Pts',(-1.32224985747682,-1.,1.59471591079403));
#28075=CARTESIAN_POINT('Ctrl Pts',(-1.32224985747682,1.,1.59471591079403));
#28076=CARTESIAN_POINT('Ctrl Pts',(-1.32381550858256,-1.,1.60073511858687));
#28077=CARTESIAN_POINT('Ctrl Pts',(-1.32381550858256,1.,1.60073511858687));
#28078=CARTESIAN_POINT('Ctrl Pts',(-1.32534250785782,-1.,1.60677758290954));
#28079=CARTESIAN_POINT('Ctrl Pts',(-1.32534250785782,1.,1.60677758290954));
#28080=CARTESIAN_POINT('Ctrl Pts',(-1.32683074483356,-1.,1.6128423401575));
#28081=CARTESIAN_POINT('Ctrl Pts',(-1.32683074483356,1.,1.6128423401575));
#28082=CARTESIAN_POINT('Ctrl Pts',(-1.32828000610449,-1.,1.61892832270724));
#28083=CARTESIAN_POINT('Ctrl Pts',(-1.32828000610449,1.,1.61892832270724));
#28084=CARTESIAN_POINT('Ctrl Pts',(-1.3296901950568,-1.,1.62503464209797));
#28085=CARTESIAN_POINT('Ctrl Pts',(-1.3296901950568,1.,1.62503464209797));
#28086=CARTESIAN_POINT('Ctrl Pts',(-1.33106149345645,-1.,1.63116079730923));
#28087=CARTESIAN_POINT('Ctrl Pts',(-1.33106149345645,1.,1.63116079730923));
#28088=CARTESIAN_POINT('Ctrl Pts',(-1.33239425103724,-1.,1.63730653475089));
#28089=CARTESIAN_POINT('Ctrl Pts',(-1.33239425103724,1.,1.63730653475089));
#28090=CARTESIAN_POINT('Ctrl Pts',(-1.33368890676572,-1.,1.6434717485603));
#28091=CARTESIAN_POINT('Ctrl Pts',(-1.33368890676572,1.,1.6434717485603));
#28092=CARTESIAN_POINT('Ctrl Pts',(-1.33494590467993,-1.,1.6496563728683));
#28093=CARTESIAN_POINT('Ctrl Pts',(-1.33494590467993,1.,1.6496563728683));
#28094=CARTESIAN_POINT('Ctrl Pts',(-1.33616559745172,-1.,1.65586025952593));
#28095=CARTESIAN_POINT('Ctrl Pts',(-1.33616559745172,1.,1.65586025952593));
#28096=CARTESIAN_POINT('Ctrl Pts',(-1.33734820885262,-1.,1.66208312541983));
#28097=CARTESIAN_POINT('Ctrl Pts',(-1.33734820885262,1.,1.66208312541983));
#28098=CARTESIAN_POINT('Ctrl Pts',(-1.33849388654388,-1.,1.66832460783989));
#28099=CARTESIAN_POINT('Ctrl Pts',(-1.33849388654388,1.,1.66832460783989));
#28100=CARTESIAN_POINT('Ctrl Pts',(-1.3396027347034,-1.,1.67458429426086));
#28101=CARTESIAN_POINT('Ctrl Pts',(-1.3396027347034,1.,1.67458429426086));
#28102=CARTESIAN_POINT('Ctrl Pts',(-1.34067485185203,-1.,1.68086176030362));
#28103=CARTESIAN_POINT('Ctrl Pts',(-1.34067485185203,1.,1.68086176030362));
#28104=CARTESIAN_POINT('Ctrl Pts',(-1.341710374848,-1.,1.68715660868764));
#28105=CARTESIAN_POINT('Ctrl Pts',(-1.341710374848,1.,1.68715660868764));
#28106=CARTESIAN_POINT('Ctrl Pts',(-1.34270948206319,-1.,1.6934684849687));
#28107=CARTESIAN_POINT('Ctrl Pts',(-1.34270948206319,1.,1.6934684849687));
#28108=CARTESIAN_POINT('Ctrl Pts',(-1.34367237124483,-1.,1.69979707754427));
#28109=CARTESIAN_POINT('Ctrl Pts',(-1.34367237124483,1.,1.69979707754427));
#28110=CARTESIAN_POINT('Ctrl Pts',(-1.34459924533831,-1.,1.70614212266738));
#28111=CARTESIAN_POINT('Ctrl Pts',(-1.34459924533831,1.,1.70614212266738));
#28112=CARTESIAN_POINT('Ctrl Pts',(-1.34549029589416,-1.,1.71250340686822));
#28113=CARTESIAN_POINT('Ctrl Pts',(-1.34549029589416,1.,1.71250340686822));
#28114=CARTESIAN_POINT('Ctrl Pts',(-1.34634568653227,-1.,1.7188807715049));
#28115=CARTESIAN_POINT('Ctrl Pts',(-1.34634568653227,1.,1.7188807715049));
#28116=CARTESIAN_POINT('Ctrl Pts',(-1.34716554819527,-1.,1.72527410680674));
#28117=CARTESIAN_POINT('Ctrl Pts',(-1.34716554819527,1.,1.72527410680674));
#28118=CARTESIAN_POINT('Ctrl Pts',(-1.34779309152035,-1.,1.7304014965394));
#28119=CARTESIAN_POINT('Ctrl Pts',(-1.34779309152035,1.,1.7304014965394));
#28120=CARTESIAN_POINT('Ctrl Pts',(-1.34824783112887,-1.,1.73425417885907));
#28121=CARTESIAN_POINT('Ctrl Pts',(-1.34824783112887,1.,1.73425417885907));
#28122=CARTESIAN_POINT('Ctrl Pts',(-1.34854391898045,-1.,1.73682580585691));
#28123=CARTESIAN_POINT('Ctrl Pts',(-1.34854391898045,1.,1.73682580585691));
#28124=CARTESIAN_POINT('Ctrl Pts',(-1.34869019493419,-1.,1.73811241238545));
#28125=CARTESIAN_POINT('Ctrl Pts',(-1.34869019493419,1.,1.73811241238545));
#28126=CARTESIAN_POINT('',(-1.15624053661742,1.,1.31362392696032));
#28127=CARTESIAN_POINT('Ctrl Pts',(-1.15624053661742,1.,1.31362392696032));
#28128=CARTESIAN_POINT('Ctrl Pts',(-1.15950888730809,1.,1.31722977216397));
#28129=CARTESIAN_POINT('Ctrl Pts',(-1.16589330093588,1.,1.32428080721772));
#28130=CARTESIAN_POINT('Ctrl Pts',(-1.17501305789857,1.,1.33437539347008));
#28131=CARTESIAN_POINT('Ctrl Pts',(-1.18625865667441,1.,1.34687054001093));
#28132=CARTESIAN_POINT('Ctrl Pts',(-1.1987959077932,1.,1.36088705043885));
#28133=CARTESIAN_POINT('Ctrl Pts',(-1.20982812925645,1.,1.37331915607905));
#28134=CARTESIAN_POINT('Ctrl Pts',(-1.21938737280852,1.,1.38420564527715));
#28135=CARTESIAN_POINT('Ctrl Pts',(-1.22752961899387,1.,1.39361389568796));
#28136=CARTESIAN_POINT('Ctrl Pts',(-1.23434087290423,1.,1.40164708206106));
#28137=CARTESIAN_POINT('Ctrl Pts',(-1.23994455029534,1.,1.40845295531283));
#28138=CARTESIAN_POINT('Ctrl Pts',(-1.24450600513056,1.,1.41422913175179));
#28139=CARTESIAN_POINT('Ctrl Pts',(-1.24824430986571,1.,1.41923722596025));
#28140=CARTESIAN_POINT('Ctrl Pts',(-1.2514145557001,1.,1.42378102115575));
#28141=CARTESIAN_POINT('Ctrl Pts',(-1.25426945222639,1.,1.42815938799387));
#28142=CARTESIAN_POINT('Ctrl Pts',(-1.25702687965755,1.,1.43262645609691));
#28143=CARTESIAN_POINT('Ctrl Pts',(-1.25983531012005,1.,1.43734919180848));
#28144=CARTESIAN_POINT('Ctrl Pts',(-1.26273903323859,1.,1.44236470511303));
#28145=CARTESIAN_POINT('Ctrl Pts',(-1.26570925118868,1.,1.44761985001662));
#28146=CARTESIAN_POINT('Ctrl Pts',(-1.2686778680489,1.,1.45301422764247));
#28147=CARTESIAN_POINT('Ctrl Pts',(-1.27156805265289,1.,1.45843906294697));
#28148=CARTESIAN_POINT('Ctrl Pts',(-1.27433119897822,1.,1.46382431332476));
#28149=CARTESIAN_POINT('Ctrl Pts',(-1.27696414831089,1.,1.46916035917133));
#28150=CARTESIAN_POINT('Ctrl Pts',(-1.2794891824849,1.,1.4744717526707));
#28151=CARTESIAN_POINT('Ctrl Pts',(-1.28194158939517,1.,1.47980070347095));
#28152=CARTESIAN_POINT('Ctrl Pts',(-1.28435533880201,1.,1.4851881711891));
#28153=CARTESIAN_POINT('Ctrl Pts',(-1.2867467611644,1.,1.4906522831278));
#28154=CARTESIAN_POINT('Ctrl Pts',(-1.28911506584254,1.,1.49618896881754));
#28155=CARTESIAN_POINT('Ctrl Pts',(-1.29145022885181,1.,1.50178230149776));
#28156=CARTESIAN_POINT('Ctrl Pts',(-1.29373841372842,1.,1.50741159078365));
#28157=CARTESIAN_POINT('Ctrl Pts',(-1.29596850710509,1.,1.51305994241402));
#28158=CARTESIAN_POINT('Ctrl Pts',(-1.29813791800747,1.,1.51872184912724));
#28159=CARTESIAN_POINT('Ctrl Pts',(-1.30024984366328,1.,1.52439957861062));
#28160=CARTESIAN_POINT('Ctrl Pts',(-1.30231064395568,1.,1.53009970283891));
#28161=CARTESIAN_POINT('Ctrl Pts',(-1.30432735639489,1.,1.53582981268977));
#28162=CARTESIAN_POINT('Ctrl Pts',(-1.30630475189556,1.,1.54159462645432));
#28163=CARTESIAN_POINT('Ctrl Pts',(-1.30824393907473,1.,1.54739413957185));
#28164=CARTESIAN_POINT('Ctrl Pts',(-1.31014393684222,1.,1.55322568759481));
#28165=CARTESIAN_POINT('Ctrl Pts',(-1.31200264341696,1.,1.55908521254821));
#28166=CARTESIAN_POINT('Ctrl Pts',(-1.31381795281002,1.,1.56496872402353));
#28167=CARTESIAN_POINT('Ctrl Pts',(-1.31558903860016,1.,1.57087397835723));
#28168=CARTESIAN_POINT('Ctrl Pts',(-1.31731642317187,1.,1.5768005650559));
#28169=CARTESIAN_POINT('Ctrl Pts',(-1.31900135021432,1.,1.58274907898834));
#28170=CARTESIAN_POINT('Ctrl Pts',(-1.32064537110892,1.,1.58872057258245));
#28171=CARTESIAN_POINT('Ctrl Pts',(-1.32224985747682,1.,1.59471591079403));
#28172=CARTESIAN_POINT('Ctrl Pts',(-1.32381550858256,1.,1.60073511858687));
#28173=CARTESIAN_POINT('Ctrl Pts',(-1.32534250785782,1.,1.60677758290954));
#28174=CARTESIAN_POINT('Ctrl Pts',(-1.32683074483356,1.,1.6128423401575));
#28175=CARTESIAN_POINT('Ctrl Pts',(-1.32828000610449,1.,1.61892832270724));
#28176=CARTESIAN_POINT('Ctrl Pts',(-1.3296901950568,1.,1.62503464209797));
#28177=CARTESIAN_POINT('Ctrl Pts',(-1.33106149345645,1.,1.63116079730923));
#28178=CARTESIAN_POINT('Ctrl Pts',(-1.33239425103724,1.,1.63730653475089));
#28179=CARTESIAN_POINT('Ctrl Pts',(-1.33368890676572,1.,1.6434717485603));
#28180=CARTESIAN_POINT('Ctrl Pts',(-1.33494590467993,1.,1.6496563728683));
#28181=CARTESIAN_POINT('Ctrl Pts',(-1.33616559745172,1.,1.65586025952593));
#28182=CARTESIAN_POINT('Ctrl Pts',(-1.33734820885262,1.,1.66208312541983));
#28183=CARTESIAN_POINT('Ctrl Pts',(-1.33849388654388,1.,1.66832460783989));
#28184=CARTESIAN_POINT('Ctrl Pts',(-1.3396027347034,1.,1.67458429426086));
#28185=CARTESIAN_POINT('Ctrl Pts',(-1.34067485185203,1.,1.68086176030362));
#28186=CARTESIAN_POINT('Ctrl Pts',(-1.341710374848,1.,1.68715660868764));
#28187=CARTESIAN_POINT('Ctrl Pts',(-1.34270948206319,1.,1.6934684849687));
#28188=CARTESIAN_POINT('Ctrl Pts',(-1.34367237124483,1.,1.69979707754427));
#28189=CARTESIAN_POINT('Ctrl Pts',(-1.34459924533831,1.,1.70614212266738));
#28190=CARTESIAN_POINT('Ctrl Pts',(-1.34549029589416,1.,1.71250340686822));
#28191=CARTESIAN_POINT('Ctrl Pts',(-1.34634568653227,1.,1.7188807715049));
#28192=CARTESIAN_POINT('Ctrl Pts',(-1.34716554819527,1.,1.72527410680674));
#28193=CARTESIAN_POINT('Ctrl Pts',(-1.34779309152035,1.,1.7304014965394));
#28194=CARTESIAN_POINT('Ctrl Pts',(-1.34824783112887,1.,1.73425417885907));
#28195=CARTESIAN_POINT('Ctrl Pts',(-1.34854391898045,1.,1.73682580585691));
#28196=CARTESIAN_POINT('Ctrl Pts',(-1.34869019493419,1.,1.73811241238545));
#28197=CARTESIAN_POINT('',(-1.15624053661742,0.,1.31362392696032));
#28198=CARTESIAN_POINT('Origin',(0.,0.,0.));
#28199=CARTESIAN_POINT('',(-1.31362392696033,1.,1.15624053661742));
#28200=CARTESIAN_POINT('Origin',(0.,1.,0.));
#28201=CARTESIAN_POINT('',(-1.31362392696033,0.,1.15624053661742));
#28202=CARTESIAN_POINT('Ctrl Pts',(-1.73811241238545,-1.,1.34869019493419));
#28203=CARTESIAN_POINT('Ctrl Pts',(-1.73811241238545,1.,1.34869019493419));
#28204=CARTESIAN_POINT('Ctrl Pts',(-1.73682580585819,-1.,1.34854391898145));
#28205=CARTESIAN_POINT('Ctrl Pts',(-1.73682580585819,1.,1.34854391898145));
#28206=CARTESIAN_POINT('Ctrl Pts',(-1.73425417886255,-1.,1.34824783113158));
#28207=CARTESIAN_POINT('Ctrl Pts',(-1.73425417886255,1.,1.34824783113158));
#28208=CARTESIAN_POINT('Ctrl Pts',(-1.73040149654497,-1.,1.3477930915247));
#28209=CARTESIAN_POINT('Ctrl Pts',(-1.73040149654497,1.,1.3477930915247));
#28210=CARTESIAN_POINT('Ctrl Pts',(-1.72527410681298,-1.,1.34716554820013));
#28211=CARTESIAN_POINT('Ctrl Pts',(-1.72527410681298,1.,1.34716554820013));
#28212=CARTESIAN_POINT('Ctrl Pts',(-1.7188807715095,-1.,1.34634568653586));
#28213=CARTESIAN_POINT('Ctrl Pts',(-1.7188807715095,1.,1.34634568653586));
#28214=CARTESIAN_POINT('Ctrl Pts',(-1.71250340687011,-1.,1.34549029589563));
#28215=CARTESIAN_POINT('Ctrl Pts',(-1.71250340687011,1.,1.34549029589563));
#28216=CARTESIAN_POINT('Ctrl Pts',(-1.70614212266676,-1.,1.34459924533783));
#28217=CARTESIAN_POINT('Ctrl Pts',(-1.70614212266676,1.,1.34459924533783));
#28218=CARTESIAN_POINT('Ctrl Pts',(-1.69979707754221,-1.,1.34367237124322));
#28219=CARTESIAN_POINT('Ctrl Pts',(-1.69979707754221,1.,1.34367237124322));
#28220=CARTESIAN_POINT('Ctrl Pts',(-1.6934684849664,-1.,1.34270948206139));
#28221=CARTESIAN_POINT('Ctrl Pts',(-1.6934684849664,1.,1.34270948206139));
#28222=CARTESIAN_POINT('Ctrl Pts',(-1.68715660868602,-1.,1.34171037484673));
#28223=CARTESIAN_POINT('Ctrl Pts',(-1.68715660868602,1.,1.34171037484673));
#28224=CARTESIAN_POINT('Ctrl Pts',(-1.68086176030308,-1.,1.3406748518516));
#28225=CARTESIAN_POINT('Ctrl Pts',(-1.68086176030308,1.,1.3406748518516));
#28226=CARTESIAN_POINT('Ctrl Pts',(-1.67458429426126,-1.,1.33960273470372));
#28227=CARTESIAN_POINT('Ctrl Pts',(-1.67458429426126,1.,1.33960273470372));
#28228=CARTESIAN_POINT('Ctrl Pts',(-1.66832460784078,-1.,1.33849388654458));
#28229=CARTESIAN_POINT('Ctrl Pts',(-1.66832460784078,1.,1.33849388654458));
#28230=CARTESIAN_POINT('Ctrl Pts',(-1.66208312542073,-1.,1.33734820885331));
#28231=CARTESIAN_POINT('Ctrl Pts',(-1.66208312542073,1.,1.33734820885331));
#28232=CARTESIAN_POINT('Ctrl Pts',(-1.65586025952651,-1.,1.33616559745217));
#28233=CARTESIAN_POINT('Ctrl Pts',(-1.65586025952651,1.,1.33616559745217));
#28234=CARTESIAN_POINT('Ctrl Pts',(-1.64965637286843,-1.,1.33494590468003));
#28235=CARTESIAN_POINT('Ctrl Pts',(-1.64965637286843,1.,1.33494590468003));
#28236=CARTESIAN_POINT('Ctrl Pts',(-1.64347174856007,-1.,1.33368890676554));
#28237=CARTESIAN_POINT('Ctrl Pts',(-1.64347174856007,1.,1.33368890676554));
#28238=CARTESIAN_POINT('Ctrl Pts',(-1.6373065347505,-1.,1.33239425103694));
#28239=CARTESIAN_POINT('Ctrl Pts',(-1.6373065347505,1.,1.33239425103694));
#28240=CARTESIAN_POINT('Ctrl Pts',(-1.63116079730887,-1.,1.33106149345618));
#28241=CARTESIAN_POINT('Ctrl Pts',(-1.63116079730887,1.,1.33106149345618));
#28242=CARTESIAN_POINT('Ctrl Pts',(-1.62503464209777,-1.,1.32969019505665));
#28243=CARTESIAN_POINT('Ctrl Pts',(-1.62503464209777,1.,1.32969019505665));
#28244=CARTESIAN_POINT('Ctrl Pts',(-1.61892832270723,-1.,1.32828000610448));
#28245=CARTESIAN_POINT('Ctrl Pts',(-1.61892832270723,1.,1.32828000610448));
#28246=CARTESIAN_POINT('Ctrl Pts',(-1.61284234015762,-1.,1.32683074483365));
#28247=CARTESIAN_POINT('Ctrl Pts',(-1.61284234015762,1.,1.32683074483365));
#28248=CARTESIAN_POINT('Ctrl Pts',(-1.6067775829097,-1.,1.32534250785794));
#28249=CARTESIAN_POINT('Ctrl Pts',(-1.6067775829097,1.,1.32534250785794));
#28250=CARTESIAN_POINT('Ctrl Pts',(-1.600735118587,-1.,1.32381550858266));
#28251=CARTESIAN_POINT('Ctrl Pts',(-1.600735118587,1.,1.32381550858266));
#28252=CARTESIAN_POINT('Ctrl Pts',(-1.59471591079408,-1.,1.32224985747686));
#28253=CARTESIAN_POINT('Ctrl Pts',(-1.59471591079408,1.,1.32224985747686));
#28254=CARTESIAN_POINT('Ctrl Pts',(-1.58872057258244,-1.,1.32064537110891));
#28255=CARTESIAN_POINT('Ctrl Pts',(-1.58872057258244,1.,1.32064537110891));
#28256=CARTESIAN_POINT('Ctrl Pts',(-1.58274907898829,-1.,1.31900135021428));
#28257=CARTESIAN_POINT('Ctrl Pts',(-1.58274907898829,1.,1.31900135021428));
#28258=CARTESIAN_POINT('Ctrl Pts',(-1.57680056505585,-1.,1.31731642317183));
#28259=CARTESIAN_POINT('Ctrl Pts',(-1.57680056505585,1.,1.31731642317183));
#28260=CARTESIAN_POINT('Ctrl Pts',(-1.57087397835721,-1.,1.31558903860015));
#28261=CARTESIAN_POINT('Ctrl Pts',(-1.57087397835721,1.,1.31558903860015));
#28262=CARTESIAN_POINT('Ctrl Pts',(-1.56496872402352,-1.,1.31381795281002));
#28263=CARTESIAN_POINT('Ctrl Pts',(-1.56496872402352,1.,1.31381795281002));
#28264=CARTESIAN_POINT('Ctrl Pts',(-1.55908521254822,-1.,1.31200264341696));
#28265=CARTESIAN_POINT('Ctrl Pts',(-1.55908521254822,1.,1.31200264341696));
#28266=CARTESIAN_POINT('Ctrl Pts',(-1.55322568759481,-1.,1.31014393684221));
#28267=CARTESIAN_POINT('Ctrl Pts',(-1.55322568759481,1.,1.31014393684221));
#28268=CARTESIAN_POINT('Ctrl Pts',(-1.54739413957183,-1.,1.30824393907471));
#28269=CARTESIAN_POINT('Ctrl Pts',(-1.54739413957183,1.,1.30824393907471));
#28270=CARTESIAN_POINT('Ctrl Pts',(-1.54159462645428,-1.,1.30630475189553));
#28271=CARTESIAN_POINT('Ctrl Pts',(-1.54159462645428,1.,1.30630475189553));
#28272=CARTESIAN_POINT('Ctrl Pts',(-1.53582981268976,-1.,1.30432735639487));
#28273=CARTESIAN_POINT('Ctrl Pts',(-1.53582981268976,1.,1.30432735639487));
#28274=CARTESIAN_POINT('Ctrl Pts',(-1.53009970283893,-1.,1.3023106439557));
#28275=CARTESIAN_POINT('Ctrl Pts',(-1.53009970283893,1.,1.3023106439557));
#28276=CARTESIAN_POINT('Ctrl Pts',(-1.5243995786107,-1.,1.30024984366334));
#28277=CARTESIAN_POINT('Ctrl Pts',(-1.5243995786107,1.,1.30024984366334));
#28278=CARTESIAN_POINT('Ctrl Pts',(-1.51872184912735,-1.,1.29813791800757));
#28279=CARTESIAN_POINT('Ctrl Pts',(-1.51872184912735,1.,1.29813791800757));
#28280=CARTESIAN_POINT('Ctrl Pts',(-1.51305994241412,-1.,1.29596850710518));
#28281=CARTESIAN_POINT('Ctrl Pts',(-1.51305994241412,1.,1.29596850710518));
#28282=CARTESIAN_POINT('Ctrl Pts',(-1.50741159078367,-1.,1.29373841372843));
#28283=CARTESIAN_POINT('Ctrl Pts',(-1.50741159078367,1.,1.29373841372843));
#28284=CARTESIAN_POINT('Ctrl Pts',(-1.50178230149764,-1.,1.29145022885171));
#28285=CARTESIAN_POINT('Ctrl Pts',(-1.50178230149764,1.,1.29145022885171));
#28286=CARTESIAN_POINT('Ctrl Pts',(-1.49618896881729,-1.,1.28911506584232));
#28287=CARTESIAN_POINT('Ctrl Pts',(-1.49618896881729,1.,1.28911506584232));
#28288=CARTESIAN_POINT('Ctrl Pts',(-1.4906522831275,-1.,1.28674676116415));
#28289=CARTESIAN_POINT('Ctrl Pts',(-1.4906522831275,1.,1.28674676116415));
#28290=CARTESIAN_POINT('Ctrl Pts',(-1.48518817118891,-1.,1.28435533880184));
#28291=CARTESIAN_POINT('Ctrl Pts',(-1.48518817118891,1.,1.28435533880184));
#28292=CARTESIAN_POINT('Ctrl Pts',(-1.47980070347102,-1.,1.28194158939522));
#28293=CARTESIAN_POINT('Ctrl Pts',(-1.47980070347102,1.,1.28194158939522));
#28294=CARTESIAN_POINT('Ctrl Pts',(-1.4744717526711,-1.,1.27948918248524));
#28295=CARTESIAN_POINT('Ctrl Pts',(-1.4744717526711,1.,1.27948918248524));
#28296=CARTESIAN_POINT('Ctrl Pts',(-1.46916035917197,-1.,1.27696414831144));
#28297=CARTESIAN_POINT('Ctrl Pts',(-1.46916035917197,1.,1.27696414831144));
#28298=CARTESIAN_POINT('Ctrl Pts',(-1.4638243133254,-1.,1.27433119897877));
#28299=CARTESIAN_POINT('Ctrl Pts',(-1.4638243133254,1.,1.27433119897877));
#28300=CARTESIAN_POINT('Ctrl Pts',(-1.45843906294725,-1.,1.27156805265312));
#28301=CARTESIAN_POINT('Ctrl Pts',(-1.45843906294725,1.,1.27156805265312));
#28302=CARTESIAN_POINT('Ctrl Pts',(-1.45301422764205,-1.,1.26867786804854));
#28303=CARTESIAN_POINT('Ctrl Pts',(-1.45301422764205,1.,1.26867786804854));
#28304=CARTESIAN_POINT('Ctrl Pts',(-1.44761985001544,-1.,1.26570925118767));
#28305=CARTESIAN_POINT('Ctrl Pts',(-1.44761985001544,1.,1.26570925118767));
#28306=CARTESIAN_POINT('Ctrl Pts',(-1.44236470511145,-1.,1.26273903323723));
#28307=CARTESIAN_POINT('Ctrl Pts',(-1.44236470511145,1.,1.26273903323723));
#28308=CARTESIAN_POINT('Ctrl Pts',(-1.43734919180719,-1.,1.25983531011894));
#28309=CARTESIAN_POINT('Ctrl Pts',(-1.43734919180719,1.,1.25983531011894));
#28310=CARTESIAN_POINT('Ctrl Pts',(-1.43262645609679,-1.,1.25702687965744));
#28311=CARTESIAN_POINT('Ctrl Pts',(-1.43262645609679,1.,1.25702687965744));
#28312=CARTESIAN_POINT('Ctrl Pts',(-1.42815938799555,-1.,1.25426945222783));
#28313=CARTESIAN_POINT('Ctrl Pts',(-1.42815938799555,1.,1.25426945222783));
#28314=CARTESIAN_POINT('Ctrl Pts',(-1.42378102115911,-1.,1.25141455570299));
#28315=CARTESIAN_POINT('Ctrl Pts',(-1.42378102115911,1.,1.25141455570299));
#28316=CARTESIAN_POINT('Ctrl Pts',(-1.41923722596421,-1.,1.24824430986911));
#28317=CARTESIAN_POINT('Ctrl Pts',(-1.41923722596421,1.,1.24824430986911));
#28318=CARTESIAN_POINT('Ctrl Pts',(-1.41422913175437,-1.,1.24450600513278));
#28319=CARTESIAN_POINT('Ctrl Pts',(-1.41422913175437,1.,1.24450600513278));
#28320=CARTESIAN_POINT('Ctrl Pts',(-1.40845295531151,-1.,1.23994455029421));
#28321=CARTESIAN_POINT('Ctrl Pts',(-1.40845295531151,1.,1.23994455029421));
#28322=CARTESIAN_POINT('Ctrl Pts',(-1.40164708205345,-1.,1.23434087289768));
#28323=CARTESIAN_POINT('Ctrl Pts',(-1.40164708205345,1.,1.23434087289768));
#28324=CARTESIAN_POINT('Ctrl Pts',(-1.39361389567257,-1.,1.22752961898063));
#28325=CARTESIAN_POINT('Ctrl Pts',(-1.39361389567257,1.,1.22752961898063));
#28326=CARTESIAN_POINT('Ctrl Pts',(-1.38420564525391,-1.,1.21938737278853));
#28327=CARTESIAN_POINT('Ctrl Pts',(-1.38420564525391,1.,1.21938737278853));
#28328=CARTESIAN_POINT('Ctrl Pts',(-1.37331915604962,-1.,1.20982812923113));
#28329=CARTESIAN_POINT('Ctrl Pts',(-1.37331915604962,1.,1.20982812923113));
#28330=CARTESIAN_POINT('Ctrl Pts',(-1.36088705040677,-1.,1.1987959077656));
#28331=CARTESIAN_POINT('Ctrl Pts',(-1.36088705040677,1.,1.1987959077656));
#28332=CARTESIAN_POINT('Ctrl Pts',(-1.34687053998157,-1.,1.18625865664915));
#28333=CARTESIAN_POINT('Ctrl Pts',(-1.34687053998157,1.,1.18625865664915));
#28334=CARTESIAN_POINT('Ctrl Pts',(-1.33437539344842,-1.,1.17501305787994));
#28335=CARTESIAN_POINT('Ctrl Pts',(-1.33437539344842,1.,1.17501305787994));
#28336=CARTESIAN_POINT('Ctrl Pts',(-1.32428080720544,-1.,1.16589330092532));
#28337=CARTESIAN_POINT('Ctrl Pts',(-1.32428080720544,1.,1.16589330092532));
#28338=CARTESIAN_POINT('Ctrl Pts',(-1.3172297721596,-1.,1.15950888730433));
#28339=CARTESIAN_POINT('Ctrl Pts',(-1.3172297721596,1.,1.15950888730433));
#28340=CARTESIAN_POINT('Ctrl Pts',(-1.31362392696033,-1.,1.15624053661742));
#28341=CARTESIAN_POINT('Ctrl Pts',(-1.31362392696033,1.,1.15624053661742));
#28342=CARTESIAN_POINT('',(-1.73811241238545,1.,1.34869019493419));
#28343=CARTESIAN_POINT('Ctrl Pts',(-1.73811241238545,1.,1.34869019493419));
#28344=CARTESIAN_POINT('Ctrl Pts',(-1.73682580585819,1.,1.34854391898145));
#28345=CARTESIAN_POINT('Ctrl Pts',(-1.73425417886255,1.,1.34824783113158));
#28346=CARTESIAN_POINT('Ctrl Pts',(-1.73040149654497,1.,1.3477930915247));
#28347=CARTESIAN_POINT('Ctrl Pts',(-1.72527410681298,1.,1.34716554820013));
#28348=CARTESIAN_POINT('Ctrl Pts',(-1.7188807715095,1.,1.34634568653586));
#28349=CARTESIAN_POINT('Ctrl Pts',(-1.71250340687011,1.,1.34549029589563));
#28350=CARTESIAN_POINT('Ctrl Pts',(-1.70614212266676,1.,1.34459924533783));
#28351=CARTESIAN_POINT('Ctrl Pts',(-1.69979707754221,1.,1.34367237124322));
#28352=CARTESIAN_POINT('Ctrl Pts',(-1.6934684849664,1.,1.34270948206139));
#28353=CARTESIAN_POINT('Ctrl Pts',(-1.68715660868602,1.,1.34171037484673));
#28354=CARTESIAN_POINT('Ctrl Pts',(-1.68086176030308,1.,1.3406748518516));
#28355=CARTESIAN_POINT('Ctrl Pts',(-1.67458429426126,1.,1.33960273470372));
#28356=CARTESIAN_POINT('Ctrl Pts',(-1.66832460784078,1.,1.33849388654458));
#28357=CARTESIAN_POINT('Ctrl Pts',(-1.66208312542073,1.,1.33734820885331));
#28358=CARTESIAN_POINT('Ctrl Pts',(-1.65586025952651,1.,1.33616559745217));
#28359=CARTESIAN_POINT('Ctrl Pts',(-1.64965637286843,1.,1.33494590468003));
#28360=CARTESIAN_POINT('Ctrl Pts',(-1.64347174856007,1.,1.33368890676554));
#28361=CARTESIAN_POINT('Ctrl Pts',(-1.6373065347505,1.,1.33239425103694));
#28362=CARTESIAN_POINT('Ctrl Pts',(-1.63116079730887,1.,1.33106149345618));
#28363=CARTESIAN_POINT('Ctrl Pts',(-1.62503464209777,1.,1.32969019505665));
#28364=CARTESIAN_POINT('Ctrl Pts',(-1.61892832270723,1.,1.32828000610448));
#28365=CARTESIAN_POINT('Ctrl Pts',(-1.61284234015762,1.,1.32683074483365));
#28366=CARTESIAN_POINT('Ctrl Pts',(-1.6067775829097,1.,1.32534250785794));
#28367=CARTESIAN_POINT('Ctrl Pts',(-1.600735118587,1.,1.32381550858266));
#28368=CARTESIAN_POINT('Ctrl Pts',(-1.59471591079408,1.,1.32224985747686));
#28369=CARTESIAN_POINT('Ctrl Pts',(-1.58872057258244,1.,1.32064537110891));
#28370=CARTESIAN_POINT('Ctrl Pts',(-1.58274907898829,1.,1.31900135021428));
#28371=CARTESIAN_POINT('Ctrl Pts',(-1.57680056505585,1.,1.31731642317183));
#28372=CARTESIAN_POINT('Ctrl Pts',(-1.57087397835721,1.,1.31558903860015));
#28373=CARTESIAN_POINT('Ctrl Pts',(-1.56496872402352,1.,1.31381795281002));
#28374=CARTESIAN_POINT('Ctrl Pts',(-1.55908521254822,1.,1.31200264341696));
#28375=CARTESIAN_POINT('Ctrl Pts',(-1.55322568759481,1.,1.31014393684221));
#28376=CARTESIAN_POINT('Ctrl Pts',(-1.54739413957183,1.,1.30824393907471));
#28377=CARTESIAN_POINT('Ctrl Pts',(-1.54159462645428,1.,1.30630475189553));
#28378=CARTESIAN_POINT('Ctrl Pts',(-1.53582981268976,1.,1.30432735639487));
#28379=CARTESIAN_POINT('Ctrl Pts',(-1.53009970283893,1.,1.3023106439557));
#28380=CARTESIAN_POINT('Ctrl Pts',(-1.5243995786107,1.,1.30024984366334));
#28381=CARTESIAN_POINT('Ctrl Pts',(-1.51872184912735,1.,1.29813791800757));
#28382=CARTESIAN_POINT('Ctrl Pts',(-1.51305994241412,1.,1.29596850710518));
#28383=CARTESIAN_POINT('Ctrl Pts',(-1.50741159078367,1.,1.29373841372843));
#28384=CARTESIAN_POINT('Ctrl Pts',(-1.50178230149764,1.,1.29145022885171));
#28385=CARTESIAN_POINT('Ctrl Pts',(-1.49618896881729,1.,1.28911506584232));
#28386=CARTESIAN_POINT('Ctrl Pts',(-1.4906522831275,1.,1.28674676116415));
#28387=CARTESIAN_POINT('Ctrl Pts',(-1.48518817118891,1.,1.28435533880184));
#28388=CARTESIAN_POINT('Ctrl Pts',(-1.47980070347102,1.,1.28194158939522));
#28389=CARTESIAN_POINT('Ctrl Pts',(-1.4744717526711,1.,1.27948918248524));
#28390=CARTESIAN_POINT('Ctrl Pts',(-1.46916035917197,1.,1.27696414831144));
#28391=CARTESIAN_POINT('Ctrl Pts',(-1.4638243133254,1.,1.27433119897877));
#28392=CARTESIAN_POINT('Ctrl Pts',(-1.45843906294725,1.,1.27156805265312));
#28393=CARTESIAN_POINT('Ctrl Pts',(-1.45301422764205,1.,1.26867786804854));
#28394=CARTESIAN_POINT('Ctrl Pts',(-1.44761985001544,1.,1.26570925118767));
#28395=CARTESIAN_POINT('Ctrl Pts',(-1.44236470511145,1.,1.26273903323723));
#28396=CARTESIAN_POINT('Ctrl Pts',(-1.43734919180719,1.,1.25983531011894));
#28397=CARTESIAN_POINT('Ctrl Pts',(-1.43262645609679,1.,1.25702687965744));
#28398=CARTESIAN_POINT('Ctrl Pts',(-1.42815938799555,1.,1.25426945222783));
#28399=CARTESIAN_POINT('Ctrl Pts',(-1.42378102115911,1.,1.25141455570299));
#28400=CARTESIAN_POINT('Ctrl Pts',(-1.41923722596421,1.,1.24824430986911));
#28401=CARTESIAN_POINT('Ctrl Pts',(-1.41422913175437,1.,1.24450600513278));
#28402=CARTESIAN_POINT('Ctrl Pts',(-1.40845295531151,1.,1.23994455029421));
#28403=CARTESIAN_POINT('Ctrl Pts',(-1.40164708205345,1.,1.23434087289768));
#28404=CARTESIAN_POINT('Ctrl Pts',(-1.39361389567257,1.,1.22752961898063));
#28405=CARTESIAN_POINT('Ctrl Pts',(-1.38420564525391,1.,1.21938737278853));
#28406=CARTESIAN_POINT('Ctrl Pts',(-1.37331915604962,1.,1.20982812923113));
#28407=CARTESIAN_POINT('Ctrl Pts',(-1.36088705040677,1.,1.1987959077656));
#28408=CARTESIAN_POINT('Ctrl Pts',(-1.34687053998157,1.,1.18625865664915));
#28409=CARTESIAN_POINT('Ctrl Pts',(-1.33437539344842,1.,1.17501305787994));
#28410=CARTESIAN_POINT('Ctrl Pts',(-1.32428080720544,1.,1.16589330092532));
#28411=CARTESIAN_POINT('Ctrl Pts',(-1.3172297721596,1.,1.15950888730433));
#28412=CARTESIAN_POINT('Ctrl Pts',(-1.31362392696033,1.,1.15624053661742));
#28413=CARTESIAN_POINT('',(-1.73811241238545,0.,1.34869019493419));
#28414=CARTESIAN_POINT('Origin',(-1.81978687191668,0.,1.23627494547115));
#28415=CARTESIAN_POINT('',(-1.81978687191668,1.,1.23627494547115));
#28416=CARTESIAN_POINT('',(-1.73811241238545,1.,1.34869019493419));
#28417=CARTESIAN_POINT('',(-1.81978687191668,0.,1.23627494547115));
#28418=CARTESIAN_POINT('Ctrl Pts',(-1.5055822144029,-1.,0.892032620296855));
#28419=CARTESIAN_POINT('Ctrl Pts',(-1.5055822144029,1.,0.892032620296855));
#28420=CARTESIAN_POINT('Ctrl Pts',(-1.50980486807181,-1.,0.894452006967538));
#28421=CARTESIAN_POINT('Ctrl Pts',(-1.50980486807181,1.,0.894452006967538));
#28422=CARTESIAN_POINT('Ctrl Pts',(-1.51805569591479,-1.,0.89918504749193));
#28423=CARTESIAN_POINT('Ctrl Pts',(-1.51805569591479,1.,0.89918504749193));
#28424=CARTESIAN_POINT('Ctrl Pts',(-1.52984849890434,-1.,0.905967409640499));
#28425=CARTESIAN_POINT('Ctrl Pts',(-1.52984849890434,1.,0.905967409640499));
#28426=CARTESIAN_POINT('Ctrl Pts',(-1.54440491152808,-1.,0.91437591904658));
#28427=CARTESIAN_POINT('Ctrl Pts',(-1.54440491152808,1.,0.91437591904658));
#28428=CARTESIAN_POINT('Ctrl Pts',(-1.56065988582509,-1.,0.923832188966322));
#28429=CARTESIAN_POINT('Ctrl Pts',(-1.56065988582509,1.,0.923832188966322));
#28430=CARTESIAN_POINT('Ctrl Pts',(-1.57499388385561,-1.,0.932246680128849));
#28431=CARTESIAN_POINT('Ctrl Pts',(-1.57499388385561,1.,0.932246680128849));
#28432=CARTESIAN_POINT('Ctrl Pts',(-1.58744937489796,-1.,0.939646377909319));
#28433=CARTESIAN_POINT('Ctrl Pts',(-1.58744937489796,1.,0.939646377909319));
#28434=CARTESIAN_POINT('Ctrl Pts',(-1.59810042045408,-1.,0.946078063325796));
#28435=CARTESIAN_POINT('Ctrl Pts',(-1.59810042045408,1.,0.946078063325796));
#28436=CARTESIAN_POINT('Ctrl Pts',(-1.60706069897794,-1.,0.951613284361248));
#28437=CARTESIAN_POINT('Ctrl Pts',(-1.60706069897794,1.,0.951613284361248));
#28438=CARTESIAN_POINT('Ctrl Pts',(-1.61449324337233,-1.,0.956354422921573));
#28439=CARTESIAN_POINT('Ctrl Pts',(-1.61449324337233,1.,0.956354422921573));
#28440=CARTESIAN_POINT('Ctrl Pts',(-1.62061638139929,-1.,0.960438326099958));
#28441=CARTESIAN_POINT('Ctrl Pts',(-1.62061638139929,1.,0.960438326099958));
#28442=CARTESIAN_POINT('Ctrl Pts',(-1.6257193066974,-1.,0.964046107037821));
#28443=CARTESIAN_POINT('Ctrl Pts',(-1.6257193066974,1.,0.964046107037821));
#28444=CARTESIAN_POINT('Ctrl Pts',(-1.63013849959083,-1.,0.967387853228041));
#28445=CARTESIAN_POINT('Ctrl Pts',(-1.63013849959083,1.,0.967387853228041));
#28446=CARTESIAN_POINT('Ctrl Pts',(-1.63420665729609,-1.,0.970669715996356));
#28447=CARTESIAN_POINT('Ctrl Pts',(-1.63420665729609,1.,0.970669715996356));
#28448=CARTESIAN_POINT('Ctrl Pts',(-1.63820952658157,-1.,0.974066058287501));
#28449=CARTESIAN_POINT('Ctrl Pts',(-1.63820952658157,1.,0.974066058287501));
#28450=CARTESIAN_POINT('Ctrl Pts',(-1.64233990826831,-1.,0.977689794120297));
#28451=CARTESIAN_POINT('Ctrl Pts',(-1.64233990826831,1.,0.977689794120297));
#28452=CARTESIAN_POINT('Ctrl Pts',(-1.64665139190834,-1.,0.981562530940574));
#28453=CARTESIAN_POINT('Ctrl Pts',(-1.64665139190834,1.,0.981562530940574));
#28454=CARTESIAN_POINT('Ctrl Pts',(-1.6511001661277,-1.,0.985642622921626));
#28455=CARTESIAN_POINT('Ctrl Pts',(-1.6511001661277,1.,0.985642622921626));
#28456=CARTESIAN_POINT('Ctrl Pts',(-1.65559044289746,-1.,0.98985562785445));
#28457=CARTESIAN_POINT('Ctrl Pts',(-1.65559044289746,1.,0.98985562785445));
#28458=CARTESIAN_POINT('Ctrl Pts',(-1.66001553809916,-1.,0.994121836661116));
#28459=CARTESIAN_POINT('Ctrl Pts',(-1.66001553809916,1.,0.994121836661116));
#28460=CARTESIAN_POINT('Ctrl Pts',(-1.66430758030304,-1.,0.998389654952317));
#28461=CARTESIAN_POINT('Ctrl Pts',(-1.66430758030304,1.,0.998389654952317));
#28462=CARTESIAN_POINT('Ctrl Pts',(-1.66846059277231,-1.,1.00265091003682));
#28463=CARTESIAN_POINT('Ctrl Pts',(-1.66846059277231,1.,1.00265091003682));
#28464=CARTESIAN_POINT('Ctrl Pts',(-1.67250335383248,-1.,1.00692206696387));
#28465=CARTESIAN_POINT('Ctrl Pts',(-1.67250335383248,1.,1.00692206696387));
#28466=CARTESIAN_POINT('Ctrl Pts',(-1.67648246776457,-1.,1.01123236493507));
#28467=CARTESIAN_POINT('Ctrl Pts',(-1.67648246776457,1.,1.01123236493507));
#28468=CARTESIAN_POINT('Ctrl Pts',(-1.6804428989482,-1.,1.01561026162787));
#28469=CARTESIAN_POINT('Ctrl Pts',(-1.6804428989482,1.,1.01561026162787));
#28470=CARTESIAN_POINT('Ctrl Pts',(-1.68440578021739,-1.,1.02006795074222));
#28471=CARTESIAN_POINT('Ctrl Pts',(-1.68440578021739,1.,1.02006795074222));
#28472=CARTESIAN_POINT('Ctrl Pts',(-1.68836910178475,-1.,1.02460180535272));
#28473=CARTESIAN_POINT('Ctrl Pts',(-1.68836910178475,1.,1.02460180535272));
#28474=CARTESIAN_POINT('Ctrl Pts',(-1.69231840863471,-1.,1.02919977579155));
#28475=CARTESIAN_POINT('Ctrl Pts',(-1.69231840863471,1.,1.02919977579155));
#28476=CARTESIAN_POINT('Ctrl Pts',(-1.69623414782769,-1.,1.03384646003587));
#28477=CARTESIAN_POINT('Ctrl Pts',(-1.69623414782769,1.,1.03384646003587));
#28478=CARTESIAN_POINT('Ctrl Pts',(-1.70010052930951,-1.,1.03852922490782));
#28479=CARTESIAN_POINT('Ctrl Pts',(-1.70010052930951,1.,1.03852922490782));
#28480=CARTESIAN_POINT('Ctrl Pts',(-1.70391338707969,-1.,1.04324363334546));
#28481=CARTESIAN_POINT('Ctrl Pts',(-1.70391338707969,1.,1.04324363334546));
#28482=CARTESIAN_POINT('Ctrl Pts',(-1.70767646263641,-1.,1.0479908540499));
#28483=CARTESIAN_POINT('Ctrl Pts',(-1.70767646263641,1.,1.0479908540499));
#28484=CARTESIAN_POINT('Ctrl Pts',(-1.71139783543986,-1.,1.05277517202854));
#28485=CARTESIAN_POINT('Ctrl Pts',(-1.71139783543986,1.,1.05277517202854));
#28486=CARTESIAN_POINT('Ctrl Pts',(-1.71508654427022,-1.,1.05760163192481));
#28487=CARTESIAN_POINT('Ctrl Pts',(-1.71508654427022,1.,1.05760163192481));
#28488=CARTESIAN_POINT('Ctrl Pts',(-1.71874858456908,-1.,1.0624732468065));
#28489=CARTESIAN_POINT('Ctrl Pts',(-1.71874858456908,1.,1.0624732468065));
#28490=CARTESIAN_POINT('Ctrl Pts',(-1.72238500928456,-1.,1.06738966975463));
#28491=CARTESIAN_POINT('Ctrl Pts',(-1.72238500928456,1.,1.06738966975463));
#28492=CARTESIAN_POINT('Ctrl Pts',(-1.72599406198489,-1.,1.07234866990252));
#28493=CARTESIAN_POINT('Ctrl Pts',(-1.72599406198489,1.,1.07234866990252));
#28494=CARTESIAN_POINT('Ctrl Pts',(-1.72957248977424,-1.,1.0773470373727));
#28495=CARTESIAN_POINT('Ctrl Pts',(-1.72957248977424,1.,1.0773470373727));
#28496=CARTESIAN_POINT('Ctrl Pts',(-1.73311705663407,-1.,1.08238162784749));
#28497=CARTESIAN_POINT('Ctrl Pts',(-1.73311705663407,1.,1.08238162784749));
#28498=CARTESIAN_POINT('Ctrl Pts',(-1.73662628326093,-1.,1.08745056285429));
#28499=CARTESIAN_POINT('Ctrl Pts',(-1.73662628326093,1.,1.08745056285429));
#28500=CARTESIAN_POINT('Ctrl Pts',(-1.74010053962252,-1.,1.09255329056496));
#28501=CARTESIAN_POINT('Ctrl Pts',(-1.74010053962252,1.,1.09255329056496));
#28502=CARTESIAN_POINT('Ctrl Pts',(-1.74354119236212,-1.,1.09768999241229));
#28503=CARTESIAN_POINT('Ctrl Pts',(-1.74354119236212,1.,1.09768999241229));
#28504=CARTESIAN_POINT('Ctrl Pts',(-1.74695004214924,-1.,1.10286118991144));
#28505=CARTESIAN_POINT('Ctrl Pts',(-1.74695004214924,1.,1.10286118991144));
#28506=CARTESIAN_POINT('Ctrl Pts',(-1.75032866075914,-1.,1.10806728183003));
#28507=CARTESIAN_POINT('Ctrl Pts',(-1.75032866075914,1.,1.10806728183003));
#28508=CARTESIAN_POINT('Ctrl Pts',(-1.75367772094617,-1.,1.11330807582542));
#28509=CARTESIAN_POINT('Ctrl Pts',(-1.75367772094617,1.,1.11330807582542));
#28510=CARTESIAN_POINT('Ctrl Pts',(-1.75699720772089,-1.,1.11858293216752));
#28511=CARTESIAN_POINT('Ctrl Pts',(-1.75699720772089,1.,1.11858293216752));
#28512=CARTESIAN_POINT('Ctrl Pts',(-1.76028671825084,-1.,1.12389096855078));
#28513=CARTESIAN_POINT('Ctrl Pts',(-1.76028671825084,1.,1.12389096855078));
#28514=CARTESIAN_POINT('Ctrl Pts',(-1.76354571966171,-1.,1.12923123555076));
#28515=CARTESIAN_POINT('Ctrl Pts',(-1.76354571966171,1.,1.12923123555076));
#28516=CARTESIAN_POINT('Ctrl Pts',(-1.76677384551883,-1.,1.13460291804635));
#28517=CARTESIAN_POINT('Ctrl Pts',(-1.76677384551883,1.,1.13460291804635));
#28518=CARTESIAN_POINT('Ctrl Pts',(-1.76997111386806,-1.,1.14000548337));
#28519=CARTESIAN_POINT('Ctrl Pts',(-1.76997111386806,1.,1.14000548337));
#28520=CARTESIAN_POINT('Ctrl Pts',(-1.77313777896234,-1.,1.14543858226948));
#28521=CARTESIAN_POINT('Ctrl Pts',(-1.77313777896234,1.,1.14543858226948));
#28522=CARTESIAN_POINT('Ctrl Pts',(-1.77627422557034,-1.,1.15090197841531));
#28523=CARTESIAN_POINT('Ctrl Pts',(-1.77627422557034,1.,1.15090197841531));
#28524=CARTESIAN_POINT('Ctrl Pts',(-1.77938085564261,-1.,1.15639547194689));
#28525=CARTESIAN_POINT('Ctrl Pts',(-1.77938085564261,1.,1.15639547194689));
#28526=CARTESIAN_POINT('Ctrl Pts',(-1.78245795880949,-1.,1.16191881298458));
#28527=CARTESIAN_POINT('Ctrl Pts',(-1.78245795880949,1.,1.16191881298458));
#28528=CARTESIAN_POINT('Ctrl Pts',(-1.78550566040349,-1.,1.16747166312239));
#28529=CARTESIAN_POINT('Ctrl Pts',(-1.78550566040349,1.,1.16747166312239));
#28530=CARTESIAN_POINT('Ctrl Pts',(-1.78852398877523,-1.,1.17305363177265));
#28531=CARTESIAN_POINT('Ctrl Pts',(-1.78852398877523,1.,1.17305363177265));
#28532=CARTESIAN_POINT('Ctrl Pts',(-1.79151291552646,-1.,1.17866429440781));
#28533=CARTESIAN_POINT('Ctrl Pts',(-1.79151291552646,1.,1.17866429440781));
#28534=CARTESIAN_POINT('Ctrl Pts',(-1.79447240321572,-1.,1.18430321697471));
#28535=CARTESIAN_POINT('Ctrl Pts',(-1.79447240321572,1.,1.18430321697471));
#28536=CARTESIAN_POINT('Ctrl Pts',(-1.79740245923649,-1.,1.1899699793456));
#28537=CARTESIAN_POINT('Ctrl Pts',(-1.79740245923649,1.,1.1899699793456));
#28538=CARTESIAN_POINT('Ctrl Pts',(-1.80030314370121,-1.,1.19566418930405));
#28539=CARTESIAN_POINT('Ctrl Pts',(-1.80030314370121,1.,1.19566418930405));
#28540=CARTESIAN_POINT('Ctrl Pts',(-1.8031745483882,-1.,1.2013854893912));
#28541=CARTESIAN_POINT('Ctrl Pts',(-1.8031745483882,1.,1.2013854893912));
#28542=CARTESIAN_POINT('Ctrl Pts',(-1.80601678480772,-1.,1.20713356605519));
#28543=CARTESIAN_POINT('Ctrl Pts',(-1.80601678480772,1.,1.20713356605519));
#28544=CARTESIAN_POINT('Ctrl Pts',(-1.80882996916931,-1.,1.2129081570818));
#28545=CARTESIAN_POINT('Ctrl Pts',(-1.80882996916931,1.,1.2129081570818));
#28546=CARTESIAN_POINT('Ctrl Pts',(-1.81161420806172,-1.,1.2187090610323));
#28547=CARTESIAN_POINT('Ctrl Pts',(-1.81161420806172,1.,1.2187090610323));
#28548=CARTESIAN_POINT('Ctrl Pts',(-1.81436959209778,-1.,1.22453613304507));
#28549=CARTESIAN_POINT('Ctrl Pts',(-1.81436959209778,1.,1.22453613304507));
#28550=CARTESIAN_POINT('Ctrl Pts',(-1.81655087183054,-1.,1.22921864890975));
#28551=CARTESIAN_POINT('Ctrl Pts',(-1.81655087183054,1.,1.22921864890975));
#28552=CARTESIAN_POINT('Ctrl Pts',(-1.81817389920914,-1.,1.23274224526804));
#28553=CARTESIAN_POINT('Ctrl Pts',(-1.81817389920914,1.,1.23274224526804));
#28554=CARTESIAN_POINT('Ctrl Pts',(-1.81925017193531,-1.,1.23509651170384));
#28555=CARTESIAN_POINT('Ctrl Pts',(-1.81925017193531,1.,1.23509651170384));
#28556=CARTESIAN_POINT('Ctrl Pts',(-1.81978687191668,-1.,1.23627494547115));
#28557=CARTESIAN_POINT('Ctrl Pts',(-1.81978687191668,1.,1.23627494547115));
#28558=CARTESIAN_POINT('',(-1.5055822144029,1.,0.892032620296855));
#28559=CARTESIAN_POINT('Ctrl Pts',(-1.5055822144029,1.,0.892032620296855));
#28560=CARTESIAN_POINT('Ctrl Pts',(-1.50980486807181,1.,0.894452006967538));
#28561=CARTESIAN_POINT('Ctrl Pts',(-1.51805569591479,1.,0.89918504749193));
#28562=CARTESIAN_POINT('Ctrl Pts',(-1.52984849890434,1.,0.905967409640499));
#28563=CARTESIAN_POINT('Ctrl Pts',(-1.54440491152808,1.,0.91437591904658));
#28564=CARTESIAN_POINT('Ctrl Pts',(-1.56065988582509,1.,0.923832188966322));
#28565=CARTESIAN_POINT('Ctrl Pts',(-1.57499388385561,1.,0.932246680128849));
#28566=CARTESIAN_POINT('Ctrl Pts',(-1.58744937489796,1.,0.939646377909319));
#28567=CARTESIAN_POINT('Ctrl Pts',(-1.59810042045408,1.,0.946078063325796));
#28568=CARTESIAN_POINT('Ctrl Pts',(-1.60706069897794,1.,0.951613284361248));
#28569=CARTESIAN_POINT('Ctrl Pts',(-1.61449324337233,1.,0.956354422921573));
#28570=CARTESIAN_POINT('Ctrl Pts',(-1.62061638139929,1.,0.960438326099958));
#28571=CARTESIAN_POINT('Ctrl Pts',(-1.6257193066974,1.,0.964046107037821));
#28572=CARTESIAN_POINT('Ctrl Pts',(-1.63013849959083,1.,0.967387853228041));
#28573=CARTESIAN_POINT('Ctrl Pts',(-1.63420665729609,1.,0.970669715996356));
#28574=CARTESIAN_POINT('Ctrl Pts',(-1.63820952658157,1.,0.974066058287501));
#28575=CARTESIAN_POINT('Ctrl Pts',(-1.64233990826831,1.,0.977689794120297));
#28576=CARTESIAN_POINT('Ctrl Pts',(-1.64665139190834,1.,0.981562530940574));
#28577=CARTESIAN_POINT('Ctrl Pts',(-1.6511001661277,1.,0.985642622921626));
#28578=CARTESIAN_POINT('Ctrl Pts',(-1.65559044289746,1.,0.98985562785445));
#28579=CARTESIAN_POINT('Ctrl Pts',(-1.66001553809916,1.,0.994121836661116));
#28580=CARTESIAN_POINT('Ctrl Pts',(-1.66430758030304,1.,0.998389654952317));
#28581=CARTESIAN_POINT('Ctrl Pts',(-1.66846059277231,1.,1.00265091003682));
#28582=CARTESIAN_POINT('Ctrl Pts',(-1.67250335383248,1.,1.00692206696387));
#28583=CARTESIAN_POINT('Ctrl Pts',(-1.67648246776457,1.,1.01123236493507));
#28584=CARTESIAN_POINT('Ctrl Pts',(-1.6804428989482,1.,1.01561026162787));
#28585=CARTESIAN_POINT('Ctrl Pts',(-1.68440578021739,1.,1.02006795074222));
#28586=CARTESIAN_POINT('Ctrl Pts',(-1.68836910178475,1.,1.02460180535272));
#28587=CARTESIAN_POINT('Ctrl Pts',(-1.69231840863471,1.,1.02919977579155));
#28588=CARTESIAN_POINT('Ctrl Pts',(-1.69623414782769,1.,1.03384646003587));
#28589=CARTESIAN_POINT('Ctrl Pts',(-1.70010052930951,1.,1.03852922490782));
#28590=CARTESIAN_POINT('Ctrl Pts',(-1.70391338707969,1.,1.04324363334546));
#28591=CARTESIAN_POINT('Ctrl Pts',(-1.70767646263641,1.,1.0479908540499));
#28592=CARTESIAN_POINT('Ctrl Pts',(-1.71139783543986,1.,1.05277517202854));
#28593=CARTESIAN_POINT('Ctrl Pts',(-1.71508654427022,1.,1.05760163192481));
#28594=CARTESIAN_POINT('Ctrl Pts',(-1.71874858456908,1.,1.0624732468065));
#28595=CARTESIAN_POINT('Ctrl Pts',(-1.72238500928456,1.,1.06738966975463));
#28596=CARTESIAN_POINT('Ctrl Pts',(-1.72599406198489,1.,1.07234866990252));
#28597=CARTESIAN_POINT('Ctrl Pts',(-1.72957248977424,1.,1.0773470373727));
#28598=CARTESIAN_POINT('Ctrl Pts',(-1.73311705663407,1.,1.08238162784749));
#28599=CARTESIAN_POINT('Ctrl Pts',(-1.73662628326093,1.,1.08745056285429));
#28600=CARTESIAN_POINT('Ctrl Pts',(-1.74010053962252,1.,1.09255329056496));
#28601=CARTESIAN_POINT('Ctrl Pts',(-1.74354119236212,1.,1.09768999241229));
#28602=CARTESIAN_POINT('Ctrl Pts',(-1.74695004214924,1.,1.10286118991144));
#28603=CARTESIAN_POINT('Ctrl Pts',(-1.75032866075914,1.,1.10806728183003));
#28604=CARTESIAN_POINT('Ctrl Pts',(-1.75367772094617,1.,1.11330807582542));
#28605=CARTESIAN_POINT('Ctrl Pts',(-1.75699720772089,1.,1.11858293216752));
#28606=CARTESIAN_POINT('Ctrl Pts',(-1.76028671825084,1.,1.12389096855078));
#28607=CARTESIAN_POINT('Ctrl Pts',(-1.76354571966171,1.,1.12923123555076));
#28608=CARTESIAN_POINT('Ctrl Pts',(-1.76677384551883,1.,1.13460291804635));
#28609=CARTESIAN_POINT('Ctrl Pts',(-1.76997111386806,1.,1.14000548337));
#28610=CARTESIAN_POINT('Ctrl Pts',(-1.77313777896234,1.,1.14543858226948));
#28611=CARTESIAN_POINT('Ctrl Pts',(-1.77627422557034,1.,1.15090197841531));
#28612=CARTESIAN_POINT('Ctrl Pts',(-1.77938085564261,1.,1.15639547194689));
#28613=CARTESIAN_POINT('Ctrl Pts',(-1.78245795880949,1.,1.16191881298458));
#28614=CARTESIAN_POINT('Ctrl Pts',(-1.78550566040349,1.,1.16747166312239));
#28615=CARTESIAN_POINT('Ctrl Pts',(-1.78852398877523,1.,1.17305363177265));
#28616=CARTESIAN_POINT('Ctrl Pts',(-1.79151291552646,1.,1.17866429440781));
#28617=CARTESIAN_POINT('Ctrl Pts',(-1.79447240321572,1.,1.18430321697471));
#28618=CARTESIAN_POINT('Ctrl Pts',(-1.79740245923649,1.,1.1899699793456));
#28619=CARTESIAN_POINT('Ctrl Pts',(-1.80030314370121,1.,1.19566418930405));
#28620=CARTESIAN_POINT('Ctrl Pts',(-1.8031745483882,1.,1.2013854893912));
#28621=CARTESIAN_POINT('Ctrl Pts',(-1.80601678480772,1.,1.20713356605519));
#28622=CARTESIAN_POINT('Ctrl Pts',(-1.80882996916931,1.,1.2129081570818));
#28623=CARTESIAN_POINT('Ctrl Pts',(-1.81161420806172,1.,1.2187090610323));
#28624=CARTESIAN_POINT('Ctrl Pts',(-1.81436959209778,1.,1.22453613304507));
#28625=CARTESIAN_POINT('Ctrl Pts',(-1.81655087183054,1.,1.22921864890975));
#28626=CARTESIAN_POINT('Ctrl Pts',(-1.81817389920914,1.,1.23274224526804));
#28627=CARTESIAN_POINT('Ctrl Pts',(-1.81925017193531,1.,1.23509651170384));
#28628=CARTESIAN_POINT('Ctrl Pts',(-1.81978687191668,1.,1.23627494547115));
#28629=CARTESIAN_POINT('',(-1.5055822144029,0.,0.892032620296856));
#28630=CARTESIAN_POINT('Origin',(0.,0.,0.));
#28631=CARTESIAN_POINT('',(-1.60662857109684,1.,0.693717979106305));
#28632=CARTESIAN_POINT('Origin',(0.,1.,0.));
#28633=CARTESIAN_POINT('',(-1.60662857109684,0.,0.693717979106306));
#28634=CARTESIAN_POINT('Ctrl Pts',(-2.0698113262342,-1.,0.7455743247944));
#28635=CARTESIAN_POINT('Ctrl Pts',(-2.0698113262342,1.,0.7455743247944));
#28636=CARTESIAN_POINT('Ctrl Pts',(-2.06854248895728,-1.,0.745832791378367));
#28637=CARTESIAN_POINT('Ctrl Pts',(-2.06854248895728,1.,0.745832791378367));
#28638=CARTESIAN_POINT('Ctrl Pts',(-2.06600523016815,-1.,0.7463458715442));
#28639=CARTESIAN_POINT('Ctrl Pts',(-2.06600523016815,1.,0.7463458715442));
#28640=CARTESIAN_POINT('Ctrl Pts',(-2.06220058927826,-1.,0.747103932787919));
#28641=CARTESIAN_POINT('Ctrl Pts',(-2.06220058927826,1.,0.747103932787919));
#28642=CARTESIAN_POINT('Ctrl Pts',(-2.05713023031006,-1.,0.748091554183802));
#28643=CARTESIAN_POINT('Ctrl Pts',(-2.05713023031006,1.,0.748091554183802));
#28644=CARTESIAN_POINT('Ctrl Pts',(-2.05079645592154,-1.,0.749287468665046));
#28645=CARTESIAN_POINT('Ctrl Pts',(-2.05079645592154,1.,0.749287468665046));
#28646=CARTESIAN_POINT('Ctrl Pts',(-2.04446689147979,-1.,0.750444657875576));
#28647=CARTESIAN_POINT('Ctrl Pts',(-2.04446689147979,1.,0.750444657875576));
#28648=CARTESIAN_POINT('Ctrl Pts',(-2.03814160092099,-1.,0.751562963361115));
#28649=CARTESIAN_POINT('Ctrl Pts',(-2.03814160092099,1.,0.751562963361115));
#28650=CARTESIAN_POINT('Ctrl Pts',(-2.03182068456221,-1.,0.752642180487211));
#28651=CARTESIAN_POINT('Ctrl Pts',(-2.03182068456221,1.,0.752642180487211));
#28652=CARTESIAN_POINT('Ctrl Pts',(-2.02550428623313,-1.,0.753682061112768));
#28653=CARTESIAN_POINT('Ctrl Pts',(-2.02550428623313,1.,0.753682061112768));
#28654=CARTESIAN_POINT('Ctrl Pts',(-2.01919259405809,-1.,0.754682330722816));
#28655=CARTESIAN_POINT('Ctrl Pts',(-2.01919259405809,1.,0.754682330722816));
#28656=CARTESIAN_POINT('Ctrl Pts',(-2.01288584328084,-1.,0.755642704957865));
#28657=CARTESIAN_POINT('Ctrl Pts',(-2.01288584328084,1.,0.755642704957865));
#28658=CARTESIAN_POINT('Ctrl Pts',(-2.0065843158773,-1.,0.75656290464667));
#28659=CARTESIAN_POINT('Ctrl Pts',(-2.0065843158773,1.,0.75656290464667));
#28660=CARTESIAN_POINT('Ctrl Pts',(-2.00028834739178,-1.,0.757442676862724));
#28661=CARTESIAN_POINT('Ctrl Pts',(-2.00028834739178,1.,0.757442676862724));
#28662=CARTESIAN_POINT('Ctrl Pts',(-1.99399831098817,-1.,0.758281796766761));
#28663=CARTESIAN_POINT('Ctrl Pts',(-1.99399831098817,1.,0.758281796766761));
#28664=CARTESIAN_POINT('Ctrl Pts',(-1.98771456680874,-1.,0.759080037802488));
#28665=CARTESIAN_POINT('Ctrl Pts',(-1.98771456680874,1.,0.759080037802488));
#28666=CARTESIAN_POINT('Ctrl Pts',(-1.98143741418172,-1.,0.75983714745219));
#28667=CARTESIAN_POINT('Ctrl Pts',(-1.98143741418172,1.,0.75983714745219));
#28668=CARTESIAN_POINT('Ctrl Pts',(-1.97516705321494,-1.,0.760552825409757));
#28669=CARTESIAN_POINT('Ctrl Pts',(-1.97516705321494,1.,0.760552825409757));
#28670=CARTESIAN_POINT('Ctrl Pts',(-1.96890351582499,-1.,0.76122669048382));
#28671=CARTESIAN_POINT('Ctrl Pts',(-1.96890351582499,1.,0.76122669048382));
#28672=CARTESIAN_POINT('Ctrl Pts',(-1.96264672744186,-1.,0.761858300014423));
#28673=CARTESIAN_POINT('Ctrl Pts',(-1.96264672744186,1.,0.761858300014423));
#28674=CARTESIAN_POINT('Ctrl Pts',(-1.95639665309869,-1.,0.762447203806179));
#28675=CARTESIAN_POINT('Ctrl Pts',(-1.95639665309869,1.,0.762447203806179));
#28676=CARTESIAN_POINT('Ctrl Pts',(-1.95015342590024,-1.,0.762992990878769));
#28677=CARTESIAN_POINT('Ctrl Pts',(-1.95015342590024,1.,0.762992990878769));
#28678=CARTESIAN_POINT('Ctrl Pts',(-1.9439174661764,-1.,0.763495333538629));
#28679=CARTESIAN_POINT('Ctrl Pts',(-1.9439174661764,1.,0.763495333538629));
#28680=CARTESIAN_POINT('Ctrl Pts',(-1.93768964875886,-1.,0.763954049121458));
#28681=CARTESIAN_POINT('Ctrl Pts',(-1.93768964875886,1.,0.763954049121458));
#28682=CARTESIAN_POINT('Ctrl Pts',(-1.93147105496382,-1.,0.76436901067394));
#28683=CARTESIAN_POINT('Ctrl Pts',(-1.93147105496382,1.,0.76436901067394));
#28684=CARTESIAN_POINT('Ctrl Pts',(-1.92526263537048,-1.,0.764740025488211));
#28685=CARTESIAN_POINT('Ctrl Pts',(-1.92526263537048,1.,0.764740025488211));
#28686=CARTESIAN_POINT('Ctrl Pts',(-1.91906491634196,-1.,0.765066729667088));
#28687=CARTESIAN_POINT('Ctrl Pts',(-1.91906491634196,1.,0.765066729667088));
#28688=CARTESIAN_POINT('Ctrl Pts',(-1.91287765805169,-1.,0.765348465884722));
#28689=CARTESIAN_POINT('Ctrl Pts',(-1.91287765805169,1.,0.765348465884722));
#28690=CARTESIAN_POINT('Ctrl Pts',(-1.90669961402356,-1.,0.765584196937919));
#28691=CARTESIAN_POINT('Ctrl Pts',(-1.90669961402356,1.,0.765584196937919));
#28692=CARTESIAN_POINT('Ctrl Pts',(-1.90052930393596,-1.,0.765772772593386));
#28693=CARTESIAN_POINT('Ctrl Pts',(-1.90052930393596,1.,0.765772772593386));
#28694=CARTESIAN_POINT('Ctrl Pts',(-1.89436577771388,-1.,0.765913193856978));
#28695=CARTESIAN_POINT('Ctrl Pts',(-1.89436577771388,1.,0.765913193856978));
#28696=CARTESIAN_POINT('Ctrl Pts',(-1.88820926433409,-1.,0.766004837062091));
#28697=CARTESIAN_POINT('Ctrl Pts',(-1.88820926433409,1.,0.766004837062091));
#28698=CARTESIAN_POINT('Ctrl Pts',(-1.88206215302561,-1.,0.766047794851864));
#28699=CARTESIAN_POINT('Ctrl Pts',(-1.88206215302561,1.,0.766047794851864));
#28700=CARTESIAN_POINT('Ctrl Pts',(-1.87592888967883,-1.,0.766042837036744));
#28701=CARTESIAN_POINT('Ctrl Pts',(-1.87592888967883,1.,0.766042837036744));
#28702=CARTESIAN_POINT('Ctrl Pts',(-1.86981398314341,-1.,0.765990708546091));
#28703=CARTESIAN_POINT('Ctrl Pts',(-1.86981398314341,1.,0.765990708546091));
#28704=CARTESIAN_POINT('Ctrl Pts',(-1.86372027063312,-1.,0.765891519092547));
#28705=CARTESIAN_POINT('Ctrl Pts',(-1.86372027063312,1.,0.765891519092547));
#28706=CARTESIAN_POINT('Ctrl Pts',(-1.85764741390394,-1.,0.765744212909318));
#28707=CARTESIAN_POINT('Ctrl Pts',(-1.85764741390394,1.,0.765744212909318));
#28708=CARTESIAN_POINT('Ctrl Pts',(-1.85158945130063,-1.,0.765545710619062));
#28709=CARTESIAN_POINT('Ctrl Pts',(-1.85158945130063,1.,0.765545710619062));
#28710=CARTESIAN_POINT('Ctrl Pts',(-1.84553698875924,-1.,0.765291664862029));
#28711=CARTESIAN_POINT('Ctrl Pts',(-1.84553698875924,1.,0.765291664862029));
#28712=CARTESIAN_POINT('Ctrl Pts',(-1.83948181064835,-1.,0.764978057881737));
#28713=CARTESIAN_POINT('Ctrl Pts',(-1.83948181064835,1.,0.764978057881737));
#28714=CARTESIAN_POINT('Ctrl Pts',(-1.83342077227142,-1.,0.764602549687853));
#28715=CARTESIAN_POINT('Ctrl Pts',(-1.83342077227142,1.,0.764602549687853));
#28716=CARTESIAN_POINT('Ctrl Pts',(-1.82735991200065,-1.,0.764165902605995));
#28717=CARTESIAN_POINT('Ctrl Pts',(-1.82735991200065,1.,0.764165902605995));
#28718=CARTESIAN_POINT('Ctrl Pts',(-1.82131873145266,-1.,0.763673465462726));
#28719=CARTESIAN_POINT('Ctrl Pts',(-1.82131873145266,1.,0.763673465462726));
#28720=CARTESIAN_POINT('Ctrl Pts',(-1.8153211840553,-1.,0.763132003836634));
#28721=CARTESIAN_POINT('Ctrl Pts',(-1.8153211840553,1.,0.763132003836634));
#28722=CARTESIAN_POINT('Ctrl Pts',(-1.80938551463965,-1.,0.762546129463938));
#28723=CARTESIAN_POINT('Ctrl Pts',(-1.80938551463965,1.,0.762546129463938));
#28724=CARTESIAN_POINT('Ctrl Pts',(-1.80351583877342,-1.,0.761915336443547));
#28725=CARTESIAN_POINT('Ctrl Pts',(-1.80351583877342,1.,0.761915336443547));
#28726=CARTESIAN_POINT('Ctrl Pts',(-1.79768986997783,-1.,0.761229695230558));
#28727=CARTESIAN_POINT('Ctrl Pts',(-1.79768986997783,1.,0.761229695230558));
#28728=CARTESIAN_POINT('Ctrl Pts',(-1.7918581561088,-1.,0.760469555880749));
#28729=CARTESIAN_POINT('Ctrl Pts',(-1.7918581561088,1.,0.760469555880749));
#28730=CARTESIAN_POINT('Ctrl Pts',(-1.78596964884604,-1.,0.759614401110189));
#28731=CARTESIAN_POINT('Ctrl Pts',(-1.78596964884604,1.,0.759614401110189));
#28732=CARTESIAN_POINT('Ctrl Pts',(-1.77999411220945,-1.,0.758650626677518));
#28733=CARTESIAN_POINT('Ctrl Pts',(-1.77999411220945,1.,0.758650626677518));
#28734=CARTESIAN_POINT('Ctrl Pts',(-1.77394167108292,-1.,0.757578264077029));
#28735=CARTESIAN_POINT('Ctrl Pts',(-1.77394167108292,1.,0.757578264077029));
#28736=CARTESIAN_POINT('Ctrl Pts',(-1.76789396002998,-1.,0.75642189602781));
#28737=CARTESIAN_POINT('Ctrl Pts',(-1.76789396002998,1.,0.75642189602781));
#28738=CARTESIAN_POINT('Ctrl Pts',(-1.76197817240128,-1.,0.755220979974461));
#28739=CARTESIAN_POINT('Ctrl Pts',(-1.76197817240128,1.,0.755220979974461));
#28740=CARTESIAN_POINT('Ctrl Pts',(-1.75631083600019,-1.,0.754009254027829));
#28741=CARTESIAN_POINT('Ctrl Pts',(-1.75631083600019,1.,0.754009254027829));
#28742=CARTESIAN_POINT('Ctrl Pts',(-1.75095139468794,-1.,0.752797683531314));
#28743=CARTESIAN_POINT('Ctrl Pts',(-1.75095139468794,1.,0.752797683531314));
#28744=CARTESIAN_POINT('Ctrl Pts',(-1.74585086852502,-1.,0.751555614164482));
#28745=CARTESIAN_POINT('Ctrl Pts',(-1.74585086852502,1.,0.751555614164482));
#28746=CARTESIAN_POINT('Ctrl Pts',(-1.74080458267114,-1.,0.750193435981249));
#28747=CARTESIAN_POINT('Ctrl Pts',(-1.74080458267114,1.,0.750193435981249));
#28748=CARTESIAN_POINT('Ctrl Pts',(-1.7355035168033,-1.,0.74858246295687));
#28749=CARTESIAN_POINT('Ctrl Pts',(-1.7355035168033,1.,0.74858246295687));
#28750=CARTESIAN_POINT('Ctrl Pts',(-1.72958533647714,-1.,0.746574710097752));
#28751=CARTESIAN_POINT('Ctrl Pts',(-1.72958533647714,1.,0.746574710097752));
#28752=CARTESIAN_POINT('Ctrl Pts',(-1.72268229916769,-1.,0.744021445433093));
#28753=CARTESIAN_POINT('Ctrl Pts',(-1.72268229916769,1.,0.744021445433093));
#28754=CARTESIAN_POINT('Ctrl Pts',(-1.71447789751001,-1.,0.74079516202821));
#28755=CARTESIAN_POINT('Ctrl Pts',(-1.71447789751001,1.,0.74079516202821));
#28756=CARTESIAN_POINT('Ctrl Pts',(-1.70473309004249,-1.,0.736799665716932));
#28757=CARTESIAN_POINT('Ctrl Pts',(-1.70473309004249,1.,0.736799665716932));
#28758=CARTESIAN_POINT('Ctrl Pts',(-1.69326921972915,-1.,0.731963238685357));
#28759=CARTESIAN_POINT('Ctrl Pts',(-1.69326921972915,1.,0.731963238685357));
#28760=CARTESIAN_POINT('Ctrl Pts',(-1.67996158451922,-1.,0.726235967982445));
#28761=CARTESIAN_POINT('Ctrl Pts',(-1.67996158451922,1.,0.726235967982445));
#28762=CARTESIAN_POINT('Ctrl Pts',(-1.66472880551777,-1.,0.71958543378795));
#28763=CARTESIAN_POINT('Ctrl Pts',(-1.66472880551777,1.,0.71958543378795));
#28764=CARTESIAN_POINT('Ctrl Pts',(-1.64752408828442,-1.,0.711993139340447));
#28765=CARTESIAN_POINT('Ctrl Pts',(-1.64752408828442,1.,0.711993139340447));
#28766=CARTESIAN_POINT('Ctrl Pts',(-1.6321654166204,-1.,0.705159151977294));
#28767=CARTESIAN_POINT('Ctrl Pts',(-1.6321654166204,1.,0.705159151977294));
#28768=CARTESIAN_POINT('Ctrl Pts',(-1.61974673471117,-1.,0.699605146398837));
#28769=CARTESIAN_POINT('Ctrl Pts',(-1.61974673471117,1.,0.699605146398837));
#28770=CARTESIAN_POINT('Ctrl Pts',(-1.61106790957619,-1.,0.69571209787897));
#28771=CARTESIAN_POINT('Ctrl Pts',(-1.61106790957619,1.,0.69571209787897));
#28772=CARTESIAN_POINT('Ctrl Pts',(-1.60662857109684,-1.,0.693717979106305));
#28773=CARTESIAN_POINT('Ctrl Pts',(-1.60662857109684,1.,0.693717979106305));
#28774=CARTESIAN_POINT('',(-2.0698113262342,1.,0.7455743247944));
#28775=CARTESIAN_POINT('Ctrl Pts',(-2.0698113262342,1.,0.7455743247944));
#28776=CARTESIAN_POINT('Ctrl Pts',(-2.06854248895728,1.,0.745832791378367));
#28777=CARTESIAN_POINT('Ctrl Pts',(-2.06600523016815,1.,0.7463458715442));
#28778=CARTESIAN_POINT('Ctrl Pts',(-2.06220058927826,1.,0.747103932787919));
#28779=CARTESIAN_POINT('Ctrl Pts',(-2.05713023031006,1.,0.748091554183802));
#28780=CARTESIAN_POINT('Ctrl Pts',(-2.05079645592154,1.,0.749287468665046));
#28781=CARTESIAN_POINT('Ctrl Pts',(-2.04446689147979,1.,0.750444657875576));
#28782=CARTESIAN_POINT('Ctrl Pts',(-2.03814160092099,1.,0.751562963361115));
#28783=CARTESIAN_POINT('Ctrl Pts',(-2.03182068456221,1.,0.752642180487211));
#28784=CARTESIAN_POINT('Ctrl Pts',(-2.02550428623313,1.,0.753682061112768));
#28785=CARTESIAN_POINT('Ctrl Pts',(-2.01919259405809,1.,0.754682330722816));
#28786=CARTESIAN_POINT('Ctrl Pts',(-2.01288584328084,1.,0.755642704957865));
#28787=CARTESIAN_POINT('Ctrl Pts',(-2.0065843158773,1.,0.75656290464667));
#28788=CARTESIAN_POINT('Ctrl Pts',(-2.00028834739178,1.,0.757442676862724));
#28789=CARTESIAN_POINT('Ctrl Pts',(-1.99399831098817,1.,0.758281796766761));
#28790=CARTESIAN_POINT('Ctrl Pts',(-1.98771456680874,1.,0.759080037802488));
#28791=CARTESIAN_POINT('Ctrl Pts',(-1.98143741418172,1.,0.75983714745219));
#28792=CARTESIAN_POINT('Ctrl Pts',(-1.97516705321494,1.,0.760552825409757));
#28793=CARTESIAN_POINT('Ctrl Pts',(-1.96890351582499,1.,0.76122669048382));
#28794=CARTESIAN_POINT('Ctrl Pts',(-1.96264672744186,1.,0.761858300014423));
#28795=CARTESIAN_POINT('Ctrl Pts',(-1.95639665309869,1.,0.762447203806179));
#28796=CARTESIAN_POINT('Ctrl Pts',(-1.95015342590024,1.,0.762992990878769));
#28797=CARTESIAN_POINT('Ctrl Pts',(-1.9439174661764,1.,0.763495333538629));
#28798=CARTESIAN_POINT('Ctrl Pts',(-1.93768964875886,1.,0.763954049121458));
#28799=CARTESIAN_POINT('Ctrl Pts',(-1.93147105496382,1.,0.76436901067394));
#28800=CARTESIAN_POINT('Ctrl Pts',(-1.92526263537048,1.,0.764740025488211));
#28801=CARTESIAN_POINT('Ctrl Pts',(-1.91906491634196,1.,0.765066729667088));
#28802=CARTESIAN_POINT('Ctrl Pts',(-1.91287765805169,1.,0.765348465884722));
#28803=CARTESIAN_POINT('Ctrl Pts',(-1.90669961402356,1.,0.765584196937919));
#28804=CARTESIAN_POINT('Ctrl Pts',(-1.90052930393596,1.,0.765772772593386));
#28805=CARTESIAN_POINT('Ctrl Pts',(-1.89436577771388,1.,0.765913193856978));
#28806=CARTESIAN_POINT('Ctrl Pts',(-1.88820926433409,1.,0.766004837062091));
#28807=CARTESIAN_POINT('Ctrl Pts',(-1.88206215302561,1.,0.766047794851864));
#28808=CARTESIAN_POINT('Ctrl Pts',(-1.87592888967883,1.,0.766042837036744));
#28809=CARTESIAN_POINT('Ctrl Pts',(-1.86981398314341,1.,0.765990708546091));
#28810=CARTESIAN_POINT('Ctrl Pts',(-1.86372027063312,1.,0.765891519092547));
#28811=CARTESIAN_POINT('Ctrl Pts',(-1.85764741390394,1.,0.765744212909318));
#28812=CARTESIAN_POINT('Ctrl Pts',(-1.85158945130063,1.,0.765545710619062));
#28813=CARTESIAN_POINT('Ctrl Pts',(-1.84553698875924,1.,0.765291664862029));
#28814=CARTESIAN_POINT('Ctrl Pts',(-1.83948181064835,1.,0.764978057881737));
#28815=CARTESIAN_POINT('Ctrl Pts',(-1.83342077227142,1.,0.764602549687853));
#28816=CARTESIAN_POINT('Ctrl Pts',(-1.82735991200065,1.,0.764165902605995));
#28817=CARTESIAN_POINT('Ctrl Pts',(-1.82131873145266,1.,0.763673465462726));
#28818=CARTESIAN_POINT('Ctrl Pts',(-1.8153211840553,1.,0.763132003836634));
#28819=CARTESIAN_POINT('Ctrl Pts',(-1.80938551463965,1.,0.762546129463938));
#28820=CARTESIAN_POINT('Ctrl Pts',(-1.80351583877342,1.,0.761915336443547));
#28821=CARTESIAN_POINT('Ctrl Pts',(-1.79768986997783,1.,0.761229695230558));
#28822=CARTESIAN_POINT('Ctrl Pts',(-1.7918581561088,1.,0.760469555880749));
#28823=CARTESIAN_POINT('Ctrl Pts',(-1.78596964884604,1.,0.759614401110189));
#28824=CARTESIAN_POINT('Ctrl Pts',(-1.77999411220945,1.,0.758650626677518));
#28825=CARTESIAN_POINT('Ctrl Pts',(-1.77394167108292,1.,0.757578264077029));
#28826=CARTESIAN_POINT('Ctrl Pts',(-1.76789396002998,1.,0.75642189602781));
#28827=CARTESIAN_POINT('Ctrl Pts',(-1.76197817240128,1.,0.755220979974461));
#28828=CARTESIAN_POINT('Ctrl Pts',(-1.75631083600019,1.,0.754009254027829));
#28829=CARTESIAN_POINT('Ctrl Pts',(-1.75095139468794,1.,0.752797683531314));
#28830=CARTESIAN_POINT('Ctrl Pts',(-1.74585086852502,1.,0.751555614164482));
#28831=CARTESIAN_POINT('Ctrl Pts',(-1.74080458267114,1.,0.750193435981249));
#28832=CARTESIAN_POINT('Ctrl Pts',(-1.7355035168033,1.,0.74858246295687));
#28833=CARTESIAN_POINT('Ctrl Pts',(-1.72958533647714,1.,0.746574710097752));
#28834=CARTESIAN_POINT('Ctrl Pts',(-1.72268229916769,1.,0.744021445433093));
#28835=CARTESIAN_POINT('Ctrl Pts',(-1.71447789751001,1.,0.74079516202821));
#28836=CARTESIAN_POINT('Ctrl Pts',(-1.70473309004249,1.,0.736799665716932));
#28837=CARTESIAN_POINT('Ctrl Pts',(-1.69326921972915,1.,0.731963238685357));
#28838=CARTESIAN_POINT('Ctrl Pts',(-1.67996158451922,1.,0.726235967982445));
#28839=CARTESIAN_POINT('Ctrl Pts',(-1.66472880551777,1.,0.71958543378795));
#28840=CARTESIAN_POINT('Ctrl Pts',(-1.64752408828442,1.,0.711993139340447));
#28841=CARTESIAN_POINT('Ctrl Pts',(-1.6321654166204,1.,0.705159151977294));
#28842=CARTESIAN_POINT('Ctrl Pts',(-1.61974673471117,1.,0.699605146398837));
#28843=CARTESIAN_POINT('Ctrl Pts',(-1.61106790957619,1.,0.69571209787897));
#28844=CARTESIAN_POINT('Ctrl Pts',(-1.60662857109684,1.,0.693717979106305));
#28845=CARTESIAN_POINT('',(-2.0698113262342,0.,0.7455743247944));
#28846=CARTESIAN_POINT('Origin',(-2.11275013067528,0.,0.61342227326009));
#28847=CARTESIAN_POINT('',(-2.11275013067528,1.,0.61342227326009));
#28848=CARTESIAN_POINT('',(-2.0698113262342,1.,0.7455743247944));
#28849=CARTESIAN_POINT('',(-2.11275013067528,0.,0.61342227326009));
#28850=CARTESIAN_POINT('Ctrl Pts',(-1.7075470150345,-1.,0.383122945602004));
#28851=CARTESIAN_POINT('Ctrl Pts',(-1.7075470150345,1.,0.383122945602004));
#28852=CARTESIAN_POINT('Ctrl Pts',(-1.71231062891958,-1.,0.384119047315542));
#28853=CARTESIAN_POINT('Ctrl Pts',(-1.71231062891958,1.,0.384119047315542));
#28854=CARTESIAN_POINT('Ctrl Pts',(-1.72162022246158,-1.,0.38607079032701));
#28855=CARTESIAN_POINT('Ctrl Pts',(-1.72162022246158,1.,0.38607079032701));
#28856=CARTESIAN_POINT('Ctrl Pts',(-1.7349317097561,-1.,0.388877023509191));
#28857=CARTESIAN_POINT('Ctrl Pts',(-1.7349317097561,1.,0.388877023509191));
#28858=CARTESIAN_POINT('Ctrl Pts',(-1.75137405313962,-1.,0.392375812294307));
#28859=CARTESIAN_POINT('Ctrl Pts',(-1.75137405313962,1.,0.392375812294307));
#28860=CARTESIAN_POINT('Ctrl Pts',(-1.7697556004756,-1.,0.39634619612042));
#28861=CARTESIAN_POINT('Ctrl Pts',(-1.7697556004756,1.,0.39634619612042));
#28862=CARTESIAN_POINT('Ctrl Pts',(-1.78598826347533,-1.,0.39991940378308));
#28863=CARTESIAN_POINT('Ctrl Pts',(-1.78598826347533,1.,0.39991940378308));
#28864=CARTESIAN_POINT('Ctrl Pts',(-1.80012077176221,-1.,0.403107976170441));
#28865=CARTESIAN_POINT('Ctrl Pts',(-1.80012077176221,1.,0.403107976170441));
#28866=CARTESIAN_POINT('Ctrl Pts',(-1.81223801813988,-1.,0.405933518411838));
#28867=CARTESIAN_POINT('Ctrl Pts',(-1.81223801813988,1.,0.405933518411838));
#28868=CARTESIAN_POINT('Ctrl Pts',(-1.8224702267854,-1.,0.408428948108533));
#28869=CARTESIAN_POINT('Ctrl Pts',(-1.8224702267854,1.,0.408428948108533));
#28870=CARTESIAN_POINT('Ctrl Pts',(-1.83100408895216,-1.,0.410641256301675));
#28871=CARTESIAN_POINT('Ctrl Pts',(-1.83100408895216,1.,0.410641256301675));
#28872=CARTESIAN_POINT('Ctrl Pts',(-1.83808953475839,-1.,0.412633125322161));
#28873=CARTESIAN_POINT('Ctrl Pts',(-1.83808953475839,1.,0.412633125322161));
#28874=CARTESIAN_POINT('Ctrl Pts',(-1.8440575707371,-1.,0.41448743825434));
#28875=CARTESIAN_POINT('Ctrl Pts',(-1.8440575707371,1.,0.41448743825434));
#28876=CARTESIAN_POINT('Ctrl Pts',(-1.84929312929882,-1.,0.416300022038864));
#28877=CARTESIAN_POINT('Ctrl Pts',(-1.84929312929882,1.,0.416300022038864));
#28878=CARTESIAN_POINT('Ctrl Pts',(-1.85417632856234,-1.,0.418164129143534));
#28879=CARTESIAN_POINT('Ctrl Pts',(-1.85417632856234,1.,0.418164129143534));
#28880=CARTESIAN_POINT('Ctrl Pts',(-1.85903281096686,-1.,0.420157287975619));
#28881=CARTESIAN_POINT('Ctrl Pts',(-1.85903281096686,1.,0.420157287975619));
#28882=CARTESIAN_POINT('Ctrl Pts',(-1.86408083334028,-1.,0.422327307418275));
#28883=CARTESIAN_POINT('Ctrl Pts',(-1.86408083334028,1.,0.422327307418275));
#28884=CARTESIAN_POINT('Ctrl Pts',(-1.86937803944323,-1.,0.424678177291359));
#28885=CARTESIAN_POINT('Ctrl Pts',(-1.86937803944323,1.,0.424678177291359));
#28886=CARTESIAN_POINT('Ctrl Pts',(-1.87486989291484,-1.,0.427183828519102));
#28887=CARTESIAN_POINT('Ctrl Pts',(-1.87486989291484,1.,0.427183828519102));
#28888=CARTESIAN_POINT('Ctrl Pts',(-1.88044229001832,-1.,0.429803062482344));
#28889=CARTESIAN_POINT('Ctrl Pts',(-1.88044229001832,1.,0.429803062482344));
#28890=CARTESIAN_POINT('Ctrl Pts',(-1.88596913666793,-1.,0.432493038548748));
#28891=CARTESIAN_POINT('Ctrl Pts',(-1.88596913666793,1.,0.432493038548748));
#28892=CARTESIAN_POINT('Ctrl Pts',(-1.89136993975504,-1.,0.435225660963383));
#28893=CARTESIAN_POINT('Ctrl Pts',(-1.89136993975504,1.,0.435225660963383));
#28894=CARTESIAN_POINT('Ctrl Pts',(-1.89663648956466,-1.,0.437995003948244));
#28895=CARTESIAN_POINT('Ctrl Pts',(-1.89663648956466,1.,0.437995003948244));
#28896=CARTESIAN_POINT('Ctrl Pts',(-1.90180124389086,-1.,0.440807833704038));
#28897=CARTESIAN_POINT('Ctrl Pts',(-1.90180124389086,1.,0.440807833704038));
#28898=CARTESIAN_POINT('Ctrl Pts',(-1.90691756144898,-1.,0.44367755684915));
#28899=CARTESIAN_POINT('Ctrl Pts',(-1.90691756144898,1.,0.44367755684915));
#28900=CARTESIAN_POINT('Ctrl Pts',(-1.9120369998112,-1.,0.446617343485711));
#28901=CARTESIAN_POINT('Ctrl Pts',(-1.9120369998112,1.,0.446617343485711));
#28902=CARTESIAN_POINT('Ctrl Pts',(-1.91718342555755,-1.,0.449632260106662));
#28903=CARTESIAN_POINT('Ctrl Pts',(-1.91718342555755,1.,0.449632260106662));
#28904=CARTESIAN_POINT('Ctrl Pts',(-1.92235380648502,-1.,0.452719478359432));
#28905=CARTESIAN_POINT('Ctrl Pts',(-1.92235380648502,1.,0.452719478359432));
#28906=CARTESIAN_POINT('Ctrl Pts',(-1.92753067150476,-1.,0.455872005174371));
#28907=CARTESIAN_POINT('Ctrl Pts',(-1.92753067150476,1.,0.455872005174371));
#28908=CARTESIAN_POINT('Ctrl Pts',(-1.93269066517934,-1.,0.459081234547926));
#28909=CARTESIAN_POINT('Ctrl Pts',(-1.93269066517934,1.,0.459081234547926));
#28910=CARTESIAN_POINT('Ctrl Pts',(-1.93781486640821,-1.,0.462340031009056));
#28911=CARTESIAN_POINT('Ctrl Pts',(-1.93781486640821,1.,0.462340031009056));
#28912=CARTESIAN_POINT('Ctrl Pts',(-1.9428979419619,-1.,0.46564546202603));
#28913=CARTESIAN_POINT('Ctrl Pts',(-1.9428979419619,1.,0.46564546202603));
#28914=CARTESIAN_POINT('Ctrl Pts',(-1.94794381136514,-1.,0.468997482913135));
#28915=CARTESIAN_POINT('Ctrl Pts',(-1.94794381136514,1.,0.468997482913135));
#28916=CARTESIAN_POINT('Ctrl Pts',(-1.95296148278133,-1.,0.472397672264072));
#28917=CARTESIAN_POINT('Ctrl Pts',(-1.95296148278133,1.,0.472397672264072));
#28918=CARTESIAN_POINT('Ctrl Pts',(-1.95796111148177,-1.,0.475848034683176));
#28919=CARTESIAN_POINT('Ctrl Pts',(-1.95796111148177,1.,0.475848034683176));
#28920=CARTESIAN_POINT('Ctrl Pts',(-1.96294933055943,-1.,0.479349583074855));
#28921=CARTESIAN_POINT('Ctrl Pts',(-1.96294933055943,1.,0.479349583074855));
#28922=CARTESIAN_POINT('Ctrl Pts',(-1.96792703422362,-1.,0.48290166212069));
#28923=CARTESIAN_POINT('Ctrl Pts',(-1.96792703422362,1.,0.48290166212069));
#28924=CARTESIAN_POINT('Ctrl Pts',(-1.97289186263272,-1.,0.486502692907659));
#28925=CARTESIAN_POINT('Ctrl Pts',(-1.97289186263272,1.,0.486502692907659));
#28926=CARTESIAN_POINT('Ctrl Pts',(-1.97783973019229,-1.,0.490150627860952));
#28927=CARTESIAN_POINT('Ctrl Pts',(-1.97783973019229,1.,0.490150627860952));
#28928=CARTESIAN_POINT('Ctrl Pts',(-1.98276658761821,-1.,0.493843476541494));
#28929=CARTESIAN_POINT('Ctrl Pts',(-1.98276658761821,1.,0.493843476541494));
#28930=CARTESIAN_POINT('Ctrl Pts',(-1.98767044752932,-1.,0.497579909545574));
#28931=CARTESIAN_POINT('Ctrl Pts',(-1.98767044752932,1.,0.497579909545574));
#28932=CARTESIAN_POINT('Ctrl Pts',(-1.99255149126155,-1.,0.501359287727146));
#28933=CARTESIAN_POINT('Ctrl Pts',(-1.99255149126155,1.,0.501359287727146));
#28934=CARTESIAN_POINT('Ctrl Pts',(-1.99741107463572,-1.,0.505181361323026));
#28935=CARTESIAN_POINT('Ctrl Pts',(-1.99741107463572,1.,0.505181361323026));
#28936=CARTESIAN_POINT('Ctrl Pts',(-2.00225107134734,-1.,0.509046069886157));
#28937=CARTESIAN_POINT('Ctrl Pts',(-2.00225107134734,1.,0.509046069886157));
#28938=CARTESIAN_POINT('Ctrl Pts',(-2.00707309946949,-1.,0.512953306961792));
#28939=CARTESIAN_POINT('Ctrl Pts',(-2.00707309946949,1.,0.512953306961792));
#28940=CARTESIAN_POINT('Ctrl Pts',(-2.01187773939242,-1.,0.516902681728687));
#28941=CARTESIAN_POINT('Ctrl Pts',(-2.01187773939242,1.,0.516902681728687));
#28942=CARTESIAN_POINT('Ctrl Pts',(-2.01666477917286,-1.,0.52089359039937));
#28943=CARTESIAN_POINT('Ctrl Pts',(-2.01666477917286,1.,0.52089359039937));
#28944=CARTESIAN_POINT('Ctrl Pts',(-2.02143356304698,-1.,0.524925318333476));
#28945=CARTESIAN_POINT('Ctrl Pts',(-2.02143356304698,1.,0.524925318333476));
#28946=CARTESIAN_POINT('Ctrl Pts',(-2.0261832908329,-1.,0.528997127241914));
#28947=CARTESIAN_POINT('Ctrl Pts',(-2.0261832908329,1.,0.528997127241914));
#28948=CARTESIAN_POINT('Ctrl Pts',(-2.03091336214426,-1.,0.533108355132976));
#28949=CARTESIAN_POINT('Ctrl Pts',(-2.03091336214426,1.,0.533108355132976));
#28950=CARTESIAN_POINT('Ctrl Pts',(-2.03562362954037,-1.,0.537258489833262));
#28951=CARTESIAN_POINT('Ctrl Pts',(-2.03562362954037,1.,0.537258489833262));
#28952=CARTESIAN_POINT('Ctrl Pts',(-2.04031422690527,-1.,0.541447120615659));
#28953=CARTESIAN_POINT('Ctrl Pts',(-2.04031422690527,1.,0.541447120615659));
#28954=CARTESIAN_POINT('Ctrl Pts',(-2.04498544714588,-1.,0.54567390381743));
#28955=CARTESIAN_POINT('Ctrl Pts',(-2.04498544714588,1.,0.54567390381743));
#28956=CARTESIAN_POINT('Ctrl Pts',(-2.04963761077958,-1.,0.549938525150295));
#28957=CARTESIAN_POINT('Ctrl Pts',(-2.04963761077958,1.,0.549938525150295));
#28958=CARTESIAN_POINT('Ctrl Pts',(-2.05427091604413,-1.,0.554240657463906));
#28959=CARTESIAN_POINT('Ctrl Pts',(-2.05427091604413,1.,0.554240657463906));
#28960=CARTESIAN_POINT('Ctrl Pts',(-2.05888537756462,-1.,0.558579940185151));
#28961=CARTESIAN_POINT('Ctrl Pts',(-2.05888537756462,1.,0.558579940185151));
#28962=CARTESIAN_POINT('Ctrl Pts',(-2.06348090160589,-1.,0.562955993082261));
#28963=CARTESIAN_POINT('Ctrl Pts',(-2.06348090160589,1.,0.562955993082261));
#28964=CARTESIAN_POINT('Ctrl Pts',(-2.06805732997334,-1.,0.567368421181087));
#28965=CARTESIAN_POINT('Ctrl Pts',(-2.06805732997334,1.,0.567368421181087));
#28966=CARTESIAN_POINT('Ctrl Pts',(-2.07261449292824,-1.,0.571816823242603));
#28967=CARTESIAN_POINT('Ctrl Pts',(-2.07261449292824,1.,0.571816823242603));
#28968=CARTESIAN_POINT('Ctrl Pts',(-2.07715226767559,-1.,0.576300797416844));
#28969=CARTESIAN_POINT('Ctrl Pts',(-2.07715226767559,1.,0.576300797416844));
#28970=CARTESIAN_POINT('Ctrl Pts',(-2.08167059018418,-1.,0.580819952108063));
#28971=CARTESIAN_POINT('Ctrl Pts',(-2.08167059018418,1.,0.580819952108063));
#28972=CARTESIAN_POINT('Ctrl Pts',(-2.08616943727951,-1.,0.585373918991617));
#28973=CARTESIAN_POINT('Ctrl Pts',(-2.08616943727951,1.,0.585373918991617));
#28974=CARTESIAN_POINT('Ctrl Pts',(-2.09064881812129,-1.,0.589962365403406));
#28975=CARTESIAN_POINT('Ctrl Pts',(-2.09064881812129,1.,0.589962365403406));
#28976=CARTESIAN_POINT('Ctrl Pts',(-2.0951087622027,-1.,0.594585006052162));
#28977=CARTESIAN_POINT('Ctrl Pts',(-2.0951087622027,1.,0.594585006052162));
#28978=CARTESIAN_POINT('Ctrl Pts',(-2.0995493086477,-1.,0.599241616420533));
#28979=CARTESIAN_POINT('Ctrl Pts',(-2.0995493086477,1.,0.599241616420533));
#28980=CARTESIAN_POINT('Ctrl Pts',(-2.10397049886949,-1.,0.60393203073603));
#28981=CARTESIAN_POINT('Ctrl Pts',(-2.10397049886949,1.,0.60393203073603));
#28982=CARTESIAN_POINT('Ctrl Pts',(-2.1074919961518,-1.,0.607711315454876));
#28983=CARTESIAN_POINT('Ctrl Pts',(-2.1074919961518,1.,0.607711315454876));
#28984=CARTESIAN_POINT('Ctrl Pts',(-2.11012443807238,-1.,0.610560911689899));
#28985=CARTESIAN_POINT('Ctrl Pts',(-2.11012443807238,1.,0.610560911689899));
#28986=CARTESIAN_POINT('Ctrl Pts',(-2.11187554259986,-1.,0.6124673655618));
#28987=CARTESIAN_POINT('Ctrl Pts',(-2.11187554259986,1.,0.6124673655618));
#28988=CARTESIAN_POINT('Ctrl Pts',(-2.11275013067528,-1.,0.61342227326009));
#28989=CARTESIAN_POINT('Ctrl Pts',(-2.11275013067528,1.,0.61342227326009));
#28990=CARTESIAN_POINT('',(-1.7075470150345,1.,0.383122945602004));
#28991=CARTESIAN_POINT('Ctrl Pts',(-1.7075470150345,1.,0.383122945602004));
#28992=CARTESIAN_POINT('Ctrl Pts',(-1.71231062891958,1.,0.384119047315542));
#28993=CARTESIAN_POINT('Ctrl Pts',(-1.72162022246158,1.,0.38607079032701));
#28994=CARTESIAN_POINT('Ctrl Pts',(-1.7349317097561,1.,0.388877023509191));
#28995=CARTESIAN_POINT('Ctrl Pts',(-1.75137405313962,1.,0.392375812294307));
#28996=CARTESIAN_POINT('Ctrl Pts',(-1.7697556004756,1.,0.39634619612042));
#28997=CARTESIAN_POINT('Ctrl Pts',(-1.78598826347533,1.,0.39991940378308));
#28998=CARTESIAN_POINT('Ctrl Pts',(-1.80012077176221,1.,0.403107976170441));
#28999=CARTESIAN_POINT('Ctrl Pts',(-1.81223801813988,1.,0.405933518411838));
#29000=CARTESIAN_POINT('Ctrl Pts',(-1.8224702267854,1.,0.408428948108533));
#29001=CARTESIAN_POINT('Ctrl Pts',(-1.83100408895216,1.,0.410641256301675));
#29002=CARTESIAN_POINT('Ctrl Pts',(-1.83808953475839,1.,0.412633125322161));
#29003=CARTESIAN_POINT('Ctrl Pts',(-1.8440575707371,1.,0.41448743825434));
#29004=CARTESIAN_POINT('Ctrl Pts',(-1.84929312929882,1.,0.416300022038864));
#29005=CARTESIAN_POINT('Ctrl Pts',(-1.85417632856234,1.,0.418164129143534));
#29006=CARTESIAN_POINT('Ctrl Pts',(-1.85903281096686,1.,0.420157287975619));
#29007=CARTESIAN_POINT('Ctrl Pts',(-1.86408083334028,1.,0.422327307418275));
#29008=CARTESIAN_POINT('Ctrl Pts',(-1.86937803944323,1.,0.424678177291359));
#29009=CARTESIAN_POINT('Ctrl Pts',(-1.87486989291484,1.,0.427183828519102));
#29010=CARTESIAN_POINT('Ctrl Pts',(-1.88044229001832,1.,0.429803062482344));
#29011=CARTESIAN_POINT('Ctrl Pts',(-1.88596913666793,1.,0.432493038548748));
#29012=CARTESIAN_POINT('Ctrl Pts',(-1.89136993975504,1.,0.435225660963383));
#29013=CARTESIAN_POINT('Ctrl Pts',(-1.89663648956466,1.,0.437995003948244));
#29014=CARTESIAN_POINT('Ctrl Pts',(-1.90180124389086,1.,0.440807833704038));
#29015=CARTESIAN_POINT('Ctrl Pts',(-1.90691756144898,1.,0.44367755684915));
#29016=CARTESIAN_POINT('Ctrl Pts',(-1.9120369998112,1.,0.446617343485711));
#29017=CARTESIAN_POINT('Ctrl Pts',(-1.91718342555755,1.,0.449632260106662));
#29018=CARTESIAN_POINT('Ctrl Pts',(-1.92235380648502,1.,0.452719478359432));
#29019=CARTESIAN_POINT('Ctrl Pts',(-1.92753067150476,1.,0.455872005174371));
#29020=CARTESIAN_POINT('Ctrl Pts',(-1.93269066517934,1.,0.459081234547926));
#29021=CARTESIAN_POINT('Ctrl Pts',(-1.93781486640821,1.,0.462340031009056));
#29022=CARTESIAN_POINT('Ctrl Pts',(-1.9428979419619,1.,0.46564546202603));
#29023=CARTESIAN_POINT('Ctrl Pts',(-1.94794381136514,1.,0.468997482913135));
#29024=CARTESIAN_POINT('Ctrl Pts',(-1.95296148278133,1.,0.472397672264072));
#29025=CARTESIAN_POINT('Ctrl Pts',(-1.95796111148177,1.,0.475848034683176));
#29026=CARTESIAN_POINT('Ctrl Pts',(-1.96294933055943,1.,0.479349583074855));
#29027=CARTESIAN_POINT('Ctrl Pts',(-1.96792703422362,1.,0.48290166212069));
#29028=CARTESIAN_POINT('Ctrl Pts',(-1.97289186263272,1.,0.486502692907659));
#29029=CARTESIAN_POINT('Ctrl Pts',(-1.97783973019229,1.,0.490150627860952));
#29030=CARTESIAN_POINT('Ctrl Pts',(-1.98276658761821,1.,0.493843476541494));
#29031=CARTESIAN_POINT('Ctrl Pts',(-1.98767044752932,1.,0.497579909545574));
#29032=CARTESIAN_POINT('Ctrl Pts',(-1.99255149126155,1.,0.501359287727146));
#29033=CARTESIAN_POINT('Ctrl Pts',(-1.99741107463572,1.,0.505181361323026));
#29034=CARTESIAN_POINT('Ctrl Pts',(-2.00225107134734,1.,0.509046069886157));
#29035=CARTESIAN_POINT('Ctrl Pts',(-2.00707309946949,1.,0.512953306961792));
#29036=CARTESIAN_POINT('Ctrl Pts',(-2.01187773939242,1.,0.516902681728687));
#29037=CARTESIAN_POINT('Ctrl Pts',(-2.01666477917286,1.,0.52089359039937));
#29038=CARTESIAN_POINT('Ctrl Pts',(-2.02143356304698,1.,0.524925318333476));
#29039=CARTESIAN_POINT('Ctrl Pts',(-2.0261832908329,1.,0.528997127241914));
#29040=CARTESIAN_POINT('Ctrl Pts',(-2.03091336214426,1.,0.533108355132976));
#29041=CARTESIAN_POINT('Ctrl Pts',(-2.03562362954037,1.,0.537258489833262));
#29042=CARTESIAN_POINT('Ctrl Pts',(-2.04031422690527,1.,0.541447120615659));
#29043=CARTESIAN_POINT('Ctrl Pts',(-2.04498544714588,1.,0.54567390381743));
#29044=CARTESIAN_POINT('Ctrl Pts',(-2.04963761077958,1.,0.549938525150295));
#29045=CARTESIAN_POINT('Ctrl Pts',(-2.05427091604413,1.,0.554240657463906));
#29046=CARTESIAN_POINT('Ctrl Pts',(-2.05888537756462,1.,0.558579940185151));
#29047=CARTESIAN_POINT('Ctrl Pts',(-2.06348090160589,1.,0.562955993082261));
#29048=CARTESIAN_POINT('Ctrl Pts',(-2.06805732997334,1.,0.567368421181087));
#29049=CARTESIAN_POINT('Ctrl Pts',(-2.07261449292824,1.,0.571816823242603));
#29050=CARTESIAN_POINT('Ctrl Pts',(-2.07715226767559,1.,0.576300797416844));
#29051=CARTESIAN_POINT('Ctrl Pts',(-2.08167059018418,1.,0.580819952108063));
#29052=CARTESIAN_POINT('Ctrl Pts',(-2.08616943727951,1.,0.585373918991617));
#29053=CARTESIAN_POINT('Ctrl Pts',(-2.09064881812129,1.,0.589962365403406));
#29054=CARTESIAN_POINT('Ctrl Pts',(-2.0951087622027,1.,0.594585006052162));
#29055=CARTESIAN_POINT('Ctrl Pts',(-2.0995493086477,1.,0.599241616420533));
#29056=CARTESIAN_POINT('Ctrl Pts',(-2.10397049886949,1.,0.60393203073603));
#29057=CARTESIAN_POINT('Ctrl Pts',(-2.1074919961518,1.,0.607711315454876));
#29058=CARTESIAN_POINT('Ctrl Pts',(-2.11012443807238,1.,0.610560911689899));
#29059=CARTESIAN_POINT('Ctrl Pts',(-2.11187554259986,1.,0.6124673655618));
#29060=CARTESIAN_POINT('Ctrl Pts',(-2.11275013067528,1.,0.61342227326009));
#29061=CARTESIAN_POINT('',(-1.7075470150345,0.,0.383122945602003));
#29062=CARTESIAN_POINT('Origin',(0.,0.,0.));
#29063=CARTESIAN_POINT('',(-1.74236521665491,1.,0.163289472382896));
#29064=CARTESIAN_POINT('Origin',(0.,1.,0.));
#29065=CARTESIAN_POINT('',(-1.74236521665491,0.,0.163289472382896));
#29066=CARTESIAN_POINT('Ctrl Pts',(-2.19890268624765,-1.,0.069476445021958));
#29067=CARTESIAN_POINT('Ctrl Pts',(-2.19890268624765,1.,0.069476445021958));
#29068=CARTESIAN_POINT('Ctrl Pts',(-2.19777582085423,-1.,0.0701143536325489));
#29069=CARTESIAN_POINT('Ctrl Pts',(-2.19777582085423,1.,0.0701143536325489));
#29070=CARTESIAN_POINT('Ctrl Pts',(-2.19552129484002,-1.,0.0713863779526153));
#29071=CARTESIAN_POINT('Ctrl Pts',(-2.19552129484002,1.,0.0713863779526153));
#29072=CARTESIAN_POINT('Ctrl Pts',(-2.19213712013662,-1.,0.0732830357306724));
#29073=CARTESIAN_POINT('Ctrl Pts',(-2.19213712013662,1.,0.0732830357306724));
#29074=CARTESIAN_POINT('Ctrl Pts',(-2.1876201139953,-1.,0.0757891465836146));
#29075=CARTESIAN_POINT('Ctrl Pts',(-2.1876201139953,1.,0.0757891465836146));
#29076=CARTESIAN_POINT('Ctrl Pts',(-2.18196589448887,-1.,0.0788837727685241));
#29077=CARTESIAN_POINT('Ctrl Pts',(-2.18196589448887,1.,0.0788837727685241));
#29078=CARTESIAN_POINT('Ctrl Pts',(-2.176303712113,-1.,0.0819402680872764));
#29079=CARTESIAN_POINT('Ctrl Pts',(-2.176303712113,1.,0.0819402680872764));
#29080=CARTESIAN_POINT('Ctrl Pts',(-2.17063357870952,-1.,0.0849584620835371));
#29081=CARTESIAN_POINT('Ctrl Pts',(-2.17063357870952,1.,0.0849584620835371));
#29082=CARTESIAN_POINT('Ctrl Pts',(-2.16495552645014,-1.,0.0879381291386921));
#29083=CARTESIAN_POINT('Ctrl Pts',(-2.16495552645014,1.,0.0879381291386921));
#29084=CARTESIAN_POINT('Ctrl Pts',(-2.15926961544516,-1.,0.0908789888107264));
#29085=CARTESIAN_POINT('Ctrl Pts',(-2.15926961544516,1.,0.0908789888107264));
#29086=CARTESIAN_POINT('Ctrl Pts',(-2.1535759397817,-1.,0.0937807218867642));
#29087=CARTESIAN_POINT('Ctrl Pts',(-2.1535759397817,1.,0.0937807218867642));
#29088=CARTESIAN_POINT('Ctrl Pts',(-2.14787463531795,-1.,0.0966429852305457));
#29089=CARTESIAN_POINT('Ctrl Pts',(-2.14787463531795,1.,0.0966429852305457));
#29090=CARTESIAN_POINT('Ctrl Pts',(-2.14216588396025,-1.,0.0994654261990914));
#29091=CARTESIAN_POINT('Ctrl Pts',(-2.14216588396025,1.,0.0994654261990914));
#29092=CARTESIAN_POINT('Ctrl Pts',(-2.13644992667165,-1.,0.1022477005561));
#29093=CARTESIAN_POINT('Ctrl Pts',(-2.13644992667165,1.,0.1022477005561));
#29094=CARTESIAN_POINT('Ctrl Pts',(-2.13072704887293,-1.,0.104989479152739));
#29095=CARTESIAN_POINT('Ctrl Pts',(-2.13072704887293,1.,0.104989479152739));
#29096=CARTESIAN_POINT('Ctrl Pts',(-2.12499752307,-1.,0.10769043523109));
#29097=CARTESIAN_POINT('Ctrl Pts',(-2.12499752307,1.,0.10769043523109));
#29098=CARTESIAN_POINT('Ctrl Pts',(-2.11926155590865,-1.,0.110350236135025));
#29099=CARTESIAN_POINT('Ctrl Pts',(-2.11926155590865,1.,0.110350236135025));
#29100=CARTESIAN_POINT('Ctrl Pts',(-2.11351924490306,-1.,0.112968534419737));
#29101=CARTESIAN_POINT('Ctrl Pts',(-2.11351924490306,1.,0.112968534419737));
#29102=CARTESIAN_POINT('Ctrl Pts',(-2.10777050261309,-1.,0.115544957687926));
#29103=CARTESIAN_POINT('Ctrl Pts',(-2.10777050261309,1.,0.115544957687926));
#29104=CARTESIAN_POINT('Ctrl Pts',(-2.102015121329,-1.,0.118079107988355));
#29105=CARTESIAN_POINT('Ctrl Pts',(-2.102015121329,1.,0.118079107988355));
#29106=CARTESIAN_POINT('Ctrl Pts',(-2.0962529286773,-1.,0.120570567965122));
#29107=CARTESIAN_POINT('Ctrl Pts',(-2.0962529286773,1.,0.120570567965122));
#29108=CARTESIAN_POINT('Ctrl Pts',(-2.09048392424825,-1.,0.123018905621083));
#29109=CARTESIAN_POINT('Ctrl Pts',(-2.09048392424825,1.,0.123018905621083));
#29110=CARTESIAN_POINT('Ctrl Pts',(-2.08470840653643,-1.,0.125423679412061));
#29111=CARTESIAN_POINT('Ctrl Pts',(-2.08470840653643,1.,0.125423679412061));
#29112=CARTESIAN_POINT('Ctrl Pts',(-2.07892715110987,-1.,0.12778444527612));
#29113=CARTESIAN_POINT('Ctrl Pts',(-2.07892715110987,1.,0.12778444527612));
#29114=CARTESIAN_POINT('Ctrl Pts',(-2.07314114713063,-1.,0.130100748328403));
#29115=CARTESIAN_POINT('Ctrl Pts',(-2.07314114713063,1.,0.130100748328403));
#29116=CARTESIAN_POINT('Ctrl Pts',(-2.06735123910326,-1.,0.13237211154771));
#29117=CARTESIAN_POINT('Ctrl Pts',(-2.06735123910326,1.,0.13237211154771));
#29118=CARTESIAN_POINT('Ctrl Pts',(-2.06155781517842,-1.,0.134598026192106));
#29119=CARTESIAN_POINT('Ctrl Pts',(-2.06155781517842,1.,0.134598026192106));
#29120=CARTESIAN_POINT('Ctrl Pts',(-2.05576044414264,-1.,0.136777941218043));
#29121=CARTESIAN_POINT('Ctrl Pts',(-2.05576044414264,1.,0.136777941218043));
#29122=CARTESIAN_POINT('Ctrl Pts',(-2.04995762001328,-1.,0.138911255368966));
#29123=CARTESIAN_POINT('Ctrl Pts',(-2.04995762001328,1.,0.138911255368966));
#29124=CARTESIAN_POINT('Ctrl Pts',(-2.04414757947916,-1.,0.140997332152546));
#29125=CARTESIAN_POINT('Ctrl Pts',(-2.04414757947916,1.,0.140997332152546));
#29126=CARTESIAN_POINT('Ctrl Pts',(-2.03832911025912,-1.,0.143035515058209));
#29127=CARTESIAN_POINT('Ctrl Pts',(-2.03832911025912,1.,0.143035515058209));
#29128=CARTESIAN_POINT('Ctrl Pts',(-2.03250223739942,-1.,0.145025140186057));
#29129=CARTESIAN_POINT('Ctrl Pts',(-2.03250223739942,1.,0.145025140186057));
#29130=CARTESIAN_POINT('Ctrl Pts',(-2.02666926182017,-1.,0.146965557332583));
#29131=CARTESIAN_POINT('Ctrl Pts',(-2.02666926182017,1.,0.146965557332583));
#29132=CARTESIAN_POINT('Ctrl Pts',(-2.02083464969894,-1.,0.148856124775337));
#29133=CARTESIAN_POINT('Ctrl Pts',(-2.02083464969894,1.,0.148856124775337));
#29134=CARTESIAN_POINT('Ctrl Pts',(-2.01500291940238,-1.,0.150696157673078));
#29135=CARTESIAN_POINT('Ctrl Pts',(-2.01500291940238,1.,0.150696157673078));
#29136=CARTESIAN_POINT('Ctrl Pts',(-2.00917680318424,-1.,0.15248488362145));
#29137=CARTESIAN_POINT('Ctrl Pts',(-2.00917680318424,1.,0.15248488362145));
#29138=CARTESIAN_POINT('Ctrl Pts',(-2.00335565310543,-1.,0.154221403049722));
#29139=CARTESIAN_POINT('Ctrl Pts',(-2.00335565310543,1.,0.154221403049722));
#29140=CARTESIAN_POINT('Ctrl Pts',(-1.99753284771497,-1.,0.155904629548783));
#29141=CARTESIAN_POINT('Ctrl Pts',(-1.99753284771497,1.,0.155904629548783));
#29142=CARTESIAN_POINT('Ctrl Pts',(-1.99169810931908,-1.,0.157533331459227));
#29143=CARTESIAN_POINT('Ctrl Pts',(-1.99169810931908,1.,0.157533331459227));
#29144=CARTESIAN_POINT('Ctrl Pts',(-1.98584238283292,-1.,0.159106226437299));
#29145=CARTESIAN_POINT('Ctrl Pts',(-1.98584238283292,1.,0.159106226437299));
#29146=CARTESIAN_POINT('Ctrl Pts',(-1.97996195437559,-1.,0.160622060784611));
#29147=CARTESIAN_POINT('Ctrl Pts',(-1.97996195437559,1.,0.160622060784611));
#29148=CARTESIAN_POINT('Ctrl Pts',(-1.97406280235188,-1.,0.162079693556288));
#29149=CARTESIAN_POINT('Ctrl Pts',(-1.97406280235188,1.,0.162079693556288));
#29150=CARTESIAN_POINT('Ctrl Pts',(-1.96816512677967,-1.,0.163478185457734));
#29151=CARTESIAN_POINT('Ctrl Pts',(-1.96816512677967,1.,0.163478185457734));
#29152=CARTESIAN_POINT('Ctrl Pts',(-1.96229379940136,-1.,0.164816568920269));
#29153=CARTESIAN_POINT('Ctrl Pts',(-1.96229379940136,1.,0.164816568920269));
#29154=CARTESIAN_POINT('Ctrl Pts',(-1.9564675971873,-1.,0.166093592002812));
#29155=CARTESIAN_POINT('Ctrl Pts',(-1.9564675971873,1.,0.166093592002812));
#29156=CARTESIAN_POINT('Ctrl Pts',(-1.95069027794294,-1.,0.167307501784475));
#29157=CARTESIAN_POINT('Ctrl Pts',(-1.95069027794294,1.,0.167307501784475));
#29158=CARTESIAN_POINT('Ctrl Pts',(-1.94493757756931,-1.,0.168455741607556));
#29159=CARTESIAN_POINT('Ctrl Pts',(-1.94493757756931,1.,0.168455741607556));
#29160=CARTESIAN_POINT('Ctrl Pts',(-1.93915639211581,-1.,0.169534904817491));
#29161=CARTESIAN_POINT('Ctrl Pts',(-1.93915639211581,1.,0.169534904817491));
#29162=CARTESIAN_POINT('Ctrl Pts',(-1.93329183155539,-1.,0.170541253116201));
#29163=CARTESIAN_POINT('Ctrl Pts',(-1.93329183155539,1.,0.170541253116201));
#29164=CARTESIAN_POINT('Ctrl Pts',(-1.92731093582036,-1.,0.171471191532988));
#29165=CARTESIAN_POINT('Ctrl Pts',(-1.92731093582036,1.,0.171471191532988));
#29166=CARTESIAN_POINT('Ctrl Pts',(-1.9212233439798,-1.,0.172321621259514));
#29167=CARTESIAN_POINT('Ctrl Pts',(-1.9212233439798,1.,0.172321621259514));
#29168=CARTESIAN_POINT('Ctrl Pts',(-1.91511429159527,-1.,0.173090695383496));
#29169=CARTESIAN_POINT('Ctrl Pts',(-1.91511429159527,1.,0.173090695383496));
#29170=CARTESIAN_POINT('Ctrl Pts',(-1.90911693975267,-1.,0.173776635257817));
#29171=CARTESIAN_POINT('Ctrl Pts',(-1.90911693975267,1.,0.173776635257817));
#29172=CARTESIAN_POINT('Ctrl Pts',(-1.90335253862834,-1.,0.174375518661085));
#29173=CARTESIAN_POINT('Ctrl Pts',(-1.90335253862834,1.,0.174375518661085));
#29174=CARTESIAN_POINT('Ctrl Pts',(-1.89788101117132,-1.,0.174879405091263));
#29175=CARTESIAN_POINT('Ctrl Pts',(-1.89788101117132,1.,0.174879405091263));
#29176=CARTESIAN_POINT('Ctrl Pts',(-1.892646301985,-1.,0.175274276190844));
#29177=CARTESIAN_POINT('Ctrl Pts',(-1.892646301985,1.,0.175274276190844));
#29178=CARTESIAN_POINT('Ctrl Pts',(-1.88742606273259,-1.,0.175538155840648));
#29179=CARTESIAN_POINT('Ctrl Pts',(-1.88742606273259,1.,0.175538155840648));
#29180=CARTESIAN_POINT('Ctrl Pts',(-1.88188663145367,-1.,0.175644148889698));
#29181=CARTESIAN_POINT('Ctrl Pts',(-1.88188663145367,1.,0.175644148889698));
#29182=CARTESIAN_POINT('Ctrl Pts',(-1.87563767773588,-1.,0.175563480746485));
#29183=CARTESIAN_POINT('Ctrl Pts',(-1.87563767773588,1.,0.175563480746485));
#29184=CARTESIAN_POINT('Ctrl Pts',(-1.86828349694799,-1.,0.175268337590758));
#29185=CARTESIAN_POINT('Ctrl Pts',(-1.86828349694799,1.,0.175268337590758));
#29186=CARTESIAN_POINT('Ctrl Pts',(-1.85948367088837,-1.,0.17473525927603));
#29187=CARTESIAN_POINT('Ctrl Pts',(-1.85948367088837,1.,0.17473525927603));
#29188=CARTESIAN_POINT('Ctrl Pts',(-1.8489811319852,-1.,0.173946627587731));
#29189=CARTESIAN_POINT('Ctrl Pts',(-1.8489811319852,1.,0.173946627587731));
#29190=CARTESIAN_POINT('Ctrl Pts',(-1.83658380527692,-1.,0.1728894428919));
#29191=CARTESIAN_POINT('Ctrl Pts',(-1.83658380527692,1.,0.1728894428919));
#29192=CARTESIAN_POINT('Ctrl Pts',(-1.82215766811545,-1.,0.171554770204119));
#29193=CARTESIAN_POINT('Ctrl Pts',(-1.82215766811545,1.,0.171554770204119));
#29194=CARTESIAN_POINT('Ctrl Pts',(-1.80561530629706,-1.,0.169936923904608));
#29195=CARTESIAN_POINT('Ctrl Pts',(-1.80561530629706,1.,0.169936923904608));
#29196=CARTESIAN_POINT('Ctrl Pts',(-1.7869064998507,-1.,0.168032772805197));
#29197=CARTESIAN_POINT('Ctrl Pts',(-1.7869064998507,1.,0.168032772805197));
#29198=CARTESIAN_POINT('Ctrl Pts',(-1.77018771684844,-1.,0.1662793551464));
#29199=CARTESIAN_POINT('Ctrl Pts',(-1.77018771684844,1.,0.1662793551464));
#29200=CARTESIAN_POINT('Ctrl Pts',(-1.75666056638427,-1.,0.164834765707158));
#29201=CARTESIAN_POINT('Ctrl Pts',(-1.75666056638427,1.,0.164834765707158));
#29202=CARTESIAN_POINT('Ctrl Pts',(-1.7472034950333,-1.,0.163814161002002));
#29203=CARTESIAN_POINT('Ctrl Pts',(-1.7472034950333,1.,0.163814161002002));
#29204=CARTESIAN_POINT('Ctrl Pts',(-1.74236521665491,-1.,0.163289472382896));
#29205=CARTESIAN_POINT('Ctrl Pts',(-1.74236521665491,1.,0.163289472382896));
#29206=CARTESIAN_POINT('',(-2.19890268624765,1.,0.069476445021958));
#29207=CARTESIAN_POINT('Ctrl Pts',(-2.19890268624765,1.,0.069476445021958));
#29208=CARTESIAN_POINT('Ctrl Pts',(-2.19777582085423,1.,0.0701143536325489));
#29209=CARTESIAN_POINT('Ctrl Pts',(-2.19552129484002,1.,0.0713863779526153));
#29210=CARTESIAN_POINT('Ctrl Pts',(-2.19213712013662,1.,0.0732830357306724));
#29211=CARTESIAN_POINT('Ctrl Pts',(-2.1876201139953,1.,0.0757891465836146));
#29212=CARTESIAN_POINT('Ctrl Pts',(-2.18196589448887,1.,0.0788837727685241));
#29213=CARTESIAN_POINT('Ctrl Pts',(-2.176303712113,1.,0.0819402680872764));
#29214=CARTESIAN_POINT('Ctrl Pts',(-2.17063357870952,1.,0.0849584620835371));
#29215=CARTESIAN_POINT('Ctrl Pts',(-2.16495552645014,1.,0.0879381291386921));
#29216=CARTESIAN_POINT('Ctrl Pts',(-2.15926961544516,1.,0.0908789888107264));
#29217=CARTESIAN_POINT('Ctrl Pts',(-2.1535759397817,1.,0.0937807218867642));
#29218=CARTESIAN_POINT('Ctrl Pts',(-2.14787463531795,1.,0.0966429852305457));
#29219=CARTESIAN_POINT('Ctrl Pts',(-2.14216588396025,1.,0.0994654261990914));
#29220=CARTESIAN_POINT('Ctrl Pts',(-2.13644992667165,1.,0.1022477005561));
#29221=CARTESIAN_POINT('Ctrl Pts',(-2.13072704887293,1.,0.104989479152739));
#29222=CARTESIAN_POINT('Ctrl Pts',(-2.12499752307,1.,0.10769043523109));
#29223=CARTESIAN_POINT('Ctrl Pts',(-2.11926155590865,1.,0.110350236135025));
#29224=CARTESIAN_POINT('Ctrl Pts',(-2.11351924490306,1.,0.112968534419737));
#29225=CARTESIAN_POINT('Ctrl Pts',(-2.10777050261309,1.,0.115544957687926));
#29226=CARTESIAN_POINT('Ctrl Pts',(-2.102015121329,1.,0.118079107988355));
#29227=CARTESIAN_POINT('Ctrl Pts',(-2.0962529286773,1.,0.120570567965122));
#29228=CARTESIAN_POINT('Ctrl Pts',(-2.09048392424825,1.,0.123018905621083));
#29229=CARTESIAN_POINT('Ctrl Pts',(-2.08470840653643,1.,0.125423679412061));
#29230=CARTESIAN_POINT('Ctrl Pts',(-2.07892715110987,1.,0.12778444527612));
#29231=CARTESIAN_POINT('Ctrl Pts',(-2.07314114713063,1.,0.130100748328403));
#29232=CARTESIAN_POINT('Ctrl Pts',(-2.06735123910326,1.,0.13237211154771));
#29233=CARTESIAN_POINT('Ctrl Pts',(-2.06155781517842,1.,0.134598026192106));
#29234=CARTESIAN_POINT('Ctrl Pts',(-2.05576044414264,1.,0.136777941218043));
#29235=CARTESIAN_POINT('Ctrl Pts',(-2.04995762001328,1.,0.138911255368966));
#29236=CARTESIAN_POINT('Ctrl Pts',(-2.04414757947916,1.,0.140997332152546));
#29237=CARTESIAN_POINT('Ctrl Pts',(-2.03832911025912,1.,0.143035515058209));
#29238=CARTESIAN_POINT('Ctrl Pts',(-2.03250223739942,1.,0.145025140186057));
#29239=CARTESIAN_POINT('Ctrl Pts',(-2.02666926182017,1.,0.146965557332583));
#29240=CARTESIAN_POINT('Ctrl Pts',(-2.02083464969894,1.,0.148856124775337));
#29241=CARTESIAN_POINT('Ctrl Pts',(-2.01500291940238,1.,0.150696157673078));
#29242=CARTESIAN_POINT('Ctrl Pts',(-2.00917680318424,1.,0.15248488362145));
#29243=CARTESIAN_POINT('Ctrl Pts',(-2.00335565310543,1.,0.154221403049722));
#29244=CARTESIAN_POINT('Ctrl Pts',(-1.99753284771497,1.,0.155904629548783));
#29245=CARTESIAN_POINT('Ctrl Pts',(-1.99169810931908,1.,0.157533331459227));
#29246=CARTESIAN_POINT('Ctrl Pts',(-1.98584238283292,1.,0.159106226437299));
#29247=CARTESIAN_POINT('Ctrl Pts',(-1.97996195437559,1.,0.160622060784611));
#29248=CARTESIAN_POINT('Ctrl Pts',(-1.97406280235188,1.,0.162079693556288));
#29249=CARTESIAN_POINT('Ctrl Pts',(-1.96816512677967,1.,0.163478185457734));
#29250=CARTESIAN_POINT('Ctrl Pts',(-1.96229379940136,1.,0.164816568920269));
#29251=CARTESIAN_POINT('Ctrl Pts',(-1.9564675971873,1.,0.166093592002812));
#29252=CARTESIAN_POINT('Ctrl Pts',(-1.95069027794294,1.,0.167307501784475));
#29253=CARTESIAN_POINT('Ctrl Pts',(-1.94493757756931,1.,0.168455741607556));
#29254=CARTESIAN_POINT('Ctrl Pts',(-1.93915639211581,1.,0.169534904817491));
#29255=CARTESIAN_POINT('Ctrl Pts',(-1.93329183155539,1.,0.170541253116201));
#29256=CARTESIAN_POINT('Ctrl Pts',(-1.92731093582036,1.,0.171471191532988));
#29257=CARTESIAN_POINT('Ctrl Pts',(-1.9212233439798,1.,0.172321621259514));
#29258=CARTESIAN_POINT('Ctrl Pts',(-1.91511429159527,1.,0.173090695383496));
#29259=CARTESIAN_POINT('Ctrl Pts',(-1.90911693975267,1.,0.173776635257817));
#29260=CARTESIAN_POINT('Ctrl Pts',(-1.90335253862834,1.,0.174375518661085));
#29261=CARTESIAN_POINT('Ctrl Pts',(-1.89788101117132,1.,0.174879405091263));
#29262=CARTESIAN_POINT('Ctrl Pts',(-1.892646301985,1.,0.175274276190844));
#29263=CARTESIAN_POINT('Ctrl Pts',(-1.88742606273259,1.,0.175538155840648));
#29264=CARTESIAN_POINT('Ctrl Pts',(-1.88188663145367,1.,0.175644148889698));
#29265=CARTESIAN_POINT('Ctrl Pts',(-1.87563767773588,1.,0.175563480746485));
#29266=CARTESIAN_POINT('Ctrl Pts',(-1.86828349694799,1.,0.175268337590758));
#29267=CARTESIAN_POINT('Ctrl Pts',(-1.85948367088837,1.,0.17473525927603));
#29268=CARTESIAN_POINT('Ctrl Pts',(-1.8489811319852,1.,0.173946627587731));
#29269=CARTESIAN_POINT('Ctrl Pts',(-1.83658380527692,1.,0.1728894428919));
#29270=CARTESIAN_POINT('Ctrl Pts',(-1.82215766811545,1.,0.171554770204119));
#29271=CARTESIAN_POINT('Ctrl Pts',(-1.80561530629706,1.,0.169936923904608));
#29272=CARTESIAN_POINT('Ctrl Pts',(-1.7869064998507,1.,0.168032772805197));
#29273=CARTESIAN_POINT('Ctrl Pts',(-1.77018771684844,1.,0.1662793551464));
#29274=CARTESIAN_POINT('Ctrl Pts',(-1.75666056638427,1.,0.164834765707158));
#29275=CARTESIAN_POINT('Ctrl Pts',(-1.7472034950333,1.,0.163814161002002));
#29276=CARTESIAN_POINT('Ctrl Pts',(-1.74236521665491,1.,0.163289472382896));
#29277=CARTESIAN_POINT('',(-2.19890268624765,0.,0.069476445021958));
#29278=CARTESIAN_POINT('Origin',(-2.19890268624765,0.,-0.0694764450219585));
#29279=CARTESIAN_POINT('',(-2.19890268624765,1.,-0.0694764450219585));
#29280=CARTESIAN_POINT('',(-2.19890268624765,1.,0.069476445021958));
#29281=CARTESIAN_POINT('',(-2.19890268624765,0.,-0.0694764450219585));
#29282=CARTESIAN_POINT('Ctrl Pts',(-1.74236521665491,-1.,-0.163289472382896));
#29283=CARTESIAN_POINT('Ctrl Pts',(-1.74236521665491,1.,-0.163289472382896));
#29284=CARTESIAN_POINT('Ctrl Pts',(-1.74720349503904,-1.,-0.163814161002474));
#29285=CARTESIAN_POINT('Ctrl Pts',(-1.74720349503904,1.,-0.163814161002474));
#29286=CARTESIAN_POINT('Ctrl Pts',(-1.75666056640041,-1.,-0.164834765708484));
#29287=CARTESIAN_POINT('Ctrl Pts',(-1.75666056640041,1.,-0.164834765708484));
#29288=CARTESIAN_POINT('Ctrl Pts',(-1.77018771687692,-1.,-0.166279355148738));
#29289=CARTESIAN_POINT('Ctrl Pts',(-1.77018771687692,1.,-0.166279355148738));
#29290=CARTESIAN_POINT('Ctrl Pts',(-1.78690649988931,-1.,-0.16803277280837));
#29291=CARTESIAN_POINT('Ctrl Pts',(-1.78690649988931,1.,-0.16803277280837));
#29292=CARTESIAN_POINT('Ctrl Pts',(-1.80561530633924,-1.,-0.169936923908078));
#29293=CARTESIAN_POINT('Ctrl Pts',(-1.80561530633924,1.,-0.169936923908078));
#29294=CARTESIAN_POINT('Ctrl Pts',(-1.82215766815414,-1.,-0.171554770207306));
#29295=CARTESIAN_POINT('Ctrl Pts',(-1.82215766815414,1.,-0.171554770207306));
#29296=CARTESIAN_POINT('Ctrl Pts',(-1.83658380530747,-1.,-0.17288944289442));
#29297=CARTESIAN_POINT('Ctrl Pts',(-1.83658380530747,1.,-0.17288944289442));
#29298=CARTESIAN_POINT('Ctrl Pts',(-1.84898113200543,-1.,-0.173946627589401));
#29299=CARTESIAN_POINT('Ctrl Pts',(-1.84898113200543,1.,-0.173946627589401));
#29300=CARTESIAN_POINT('Ctrl Pts',(-1.85948367089838,-1.,-0.174735259276856));
#29301=CARTESIAN_POINT('Ctrl Pts',(-1.85948367089838,1.,-0.174735259276856));
#29302=CARTESIAN_POINT('Ctrl Pts',(-1.86828349694972,-1.,-0.175268337590901));
#29303=CARTESIAN_POINT('Ctrl Pts',(-1.86828349694972,1.,-0.175268337590901));
#29304=CARTESIAN_POINT('Ctrl Pts',(-1.87563767773249,-1.,-0.175563480746205));
#29305=CARTESIAN_POINT('Ctrl Pts',(-1.87563767773249,1.,-0.175563480746205));
#29306=CARTESIAN_POINT('Ctrl Pts',(-1.88188663144846,-1.,-0.175644148889271));
#29307=CARTESIAN_POINT('Ctrl Pts',(-1.88188663144846,1.,-0.175644148889271));
#29308=CARTESIAN_POINT('Ctrl Pts',(-1.88742606272818,-1.,-0.175538155840286));
#29309=CARTESIAN_POINT('Ctrl Pts',(-1.88742606272818,1.,-0.175538155840286));
#29310=CARTESIAN_POINT('Ctrl Pts',(-1.89264630198279,-1.,-0.175274276190664));
#29311=CARTESIAN_POINT('Ctrl Pts',(-1.89264630198279,1.,-0.175274276190664));
#29312=CARTESIAN_POINT('Ctrl Pts',(-1.89788101117148,-1.,-0.174879405091277));
#29313=CARTESIAN_POINT('Ctrl Pts',(-1.89788101117148,1.,-0.174879405091277));
#29314=CARTESIAN_POINT('Ctrl Pts',(-1.90335253863003,-1.,-0.174375518661222));
#29315=CARTESIAN_POINT('Ctrl Pts',(-1.90335253863003,1.,-0.174375518661222));
#29316=CARTESIAN_POINT('Ctrl Pts',(-1.90911693975475,-1.,-0.173776635257984));
#29317=CARTESIAN_POINT('Ctrl Pts',(-1.90911693975475,1.,-0.173776635257984));
#29318=CARTESIAN_POINT('Ctrl Pts',(-1.91511429159681,-1.,-0.173090695383619));
#29319=CARTESIAN_POINT('Ctrl Pts',(-1.91511429159681,1.,-0.173090695383619));
#29320=CARTESIAN_POINT('Ctrl Pts',(-1.92122334398034,-1.,-0.172321621259557));
#29321=CARTESIAN_POINT('Ctrl Pts',(-1.92122334398034,1.,-0.172321621259557));
#29322=CARTESIAN_POINT('Ctrl Pts',(-1.92731093582,-1.,-0.17147119153296));
#29323=CARTESIAN_POINT('Ctrl Pts',(-1.92731093582,1.,-0.17147119153296));
#29324=CARTESIAN_POINT('Ctrl Pts',(-1.93329183155455,-1.,-0.170541253116136));
#29325=CARTESIAN_POINT('Ctrl Pts',(-1.93329183155455,1.,-0.170541253116136));
#29326=CARTESIAN_POINT('Ctrl Pts',(-1.93915639211497,-1.,-0.169534904817425));
#29327=CARTESIAN_POINT('Ctrl Pts',(-1.93915639211497,1.,-0.169534904817425));
#29328=CARTESIAN_POINT('Ctrl Pts',(-1.94493757756879,-1.,-0.168455741607516));
#29329=CARTESIAN_POINT('Ctrl Pts',(-1.94493757756879,1.,-0.168455741607516));
#29330=CARTESIAN_POINT('Ctrl Pts',(-1.95069027794286,-1.,-0.167307501784469));
#29331=CARTESIAN_POINT('Ctrl Pts',(-1.95069027794286,1.,-0.167307501784469));
#29332=CARTESIAN_POINT('Ctrl Pts',(-1.95646759718755,-1.,-0.166093592002833));
#29333=CARTESIAN_POINT('Ctrl Pts',(-1.95646759718755,1.,-0.166093592002833));
#29334=CARTESIAN_POINT('Ctrl Pts',(-1.96229379940174,-1.,-0.1648165689203));
#29335=CARTESIAN_POINT('Ctrl Pts',(-1.96229379940174,1.,-0.1648165689203));
#29336=CARTESIAN_POINT('Ctrl Pts',(-1.96816512678,-1.,-0.16347818545776));
#29337=CARTESIAN_POINT('Ctrl Pts',(-1.96816512678,1.,-0.16347818545776));
#29338=CARTESIAN_POINT('Ctrl Pts',(-1.97406280235204,-1.,-0.162079693556302));
#29339=CARTESIAN_POINT('Ctrl Pts',(-1.97406280235204,1.,-0.162079693556302));
#29340=CARTESIAN_POINT('Ctrl Pts',(-1.97996195437557,-1.,-0.16062206078461));
#29341=CARTESIAN_POINT('Ctrl Pts',(-1.97996195437557,1.,-0.16062206078461));
#29342=CARTESIAN_POINT('Ctrl Pts',(-1.98584238283279,-1.,-0.159106226437289));
#29343=CARTESIAN_POINT('Ctrl Pts',(-1.98584238283279,1.,-0.159106226437289));
#29344=CARTESIAN_POINT('Ctrl Pts',(-1.99169810931893,-1.,-0.157533331459215));
#29345=CARTESIAN_POINT('Ctrl Pts',(-1.99169810931893,1.,-0.157533331459215));
#29346=CARTESIAN_POINT('Ctrl Pts',(-1.99753284771487,-1.,-0.155904629548775));
#29347=CARTESIAN_POINT('Ctrl Pts',(-1.99753284771487,1.,-0.155904629548775));
#29348=CARTESIAN_POINT('Ctrl Pts',(-2.00335565310539,-1.,-0.154221403049719));
#29349=CARTESIAN_POINT('Ctrl Pts',(-2.00335565310539,1.,-0.154221403049719));
#29350=CARTESIAN_POINT('Ctrl Pts',(-2.00917680318426,-1.,-0.152484883621452));
#29351=CARTESIAN_POINT('Ctrl Pts',(-2.00917680318426,1.,-0.152484883621452));
#29352=CARTESIAN_POINT('Ctrl Pts',(-2.01500291940243,-1.,-0.150696157673084));
#29353=CARTESIAN_POINT('Ctrl Pts',(-2.01500291940243,1.,-0.150696157673084));
#29354=CARTESIAN_POINT('Ctrl Pts',(-2.02083464969897,-1.,-0.148856124775343));
#29355=CARTESIAN_POINT('Ctrl Pts',(-2.02083464969897,1.,-0.148856124775343));
#29356=CARTESIAN_POINT('Ctrl Pts',(-2.02666926182017,-1.,-0.146965557332586));
#29357=CARTESIAN_POINT('Ctrl Pts',(-2.02666926182017,1.,-0.146965557332586));
#29358=CARTESIAN_POINT('Ctrl Pts',(-2.03250223739941,-1.,-0.145025140186058));
#29359=CARTESIAN_POINT('Ctrl Pts',(-2.03250223739941,1.,-0.145025140186058));
#29360=CARTESIAN_POINT('Ctrl Pts',(-2.03832911025913,-1.,-0.143035515058208));
#29361=CARTESIAN_POINT('Ctrl Pts',(-2.03832911025913,1.,-0.143035515058208));
#29362=CARTESIAN_POINT('Ctrl Pts',(-2.04414757947919,-1.,-0.140997332152545));
#29363=CARTESIAN_POINT('Ctrl Pts',(-2.04414757947919,1.,-0.140997332152545));
#29364=CARTESIAN_POINT('Ctrl Pts',(-2.04995762001333,-1.,-0.138911255368966));
#29365=CARTESIAN_POINT('Ctrl Pts',(-2.04995762001333,1.,-0.138911255368966));
#29366=CARTESIAN_POINT('Ctrl Pts',(-2.0557604441427,-1.,-0.136777941218044));
#29367=CARTESIAN_POINT('Ctrl Pts',(-2.0557604441427,1.,-0.136777941218044));
#29368=CARTESIAN_POINT('Ctrl Pts',(-2.06155781517844,-1.,-0.134598026192107));
#29369=CARTESIAN_POINT('Ctrl Pts',(-2.06155781517844,1.,-0.134598026192107));
#29370=CARTESIAN_POINT('Ctrl Pts',(-2.06735123910319,-1.,-0.13237211154771));
#29371=CARTESIAN_POINT('Ctrl Pts',(-2.06735123910319,1.,-0.13237211154771));
#29372=CARTESIAN_POINT('Ctrl Pts',(-2.07314114713047,-1.,-0.130100748328401));
#29373=CARTESIAN_POINT('Ctrl Pts',(-2.07314114713047,1.,-0.130100748328401));
#29374=CARTESIAN_POINT('Ctrl Pts',(-2.07892715110967,-1.,-0.127784445276116));
#29375=CARTESIAN_POINT('Ctrl Pts',(-2.07892715110967,1.,-0.127784445276116));
#29376=CARTESIAN_POINT('Ctrl Pts',(-2.08470840653628,-1.,-0.125423679412058));
#29377=CARTESIAN_POINT('Ctrl Pts',(-2.08470840653628,1.,-0.125423679412058));
#29378=CARTESIAN_POINT('Ctrl Pts',(-2.09048392424826,-1.,-0.123018905621083));
#29379=CARTESIAN_POINT('Ctrl Pts',(-2.09048392424826,1.,-0.123018905621083));
#29380=CARTESIAN_POINT('Ctrl Pts',(-2.09625292867756,-1.,-0.120570567965129));
#29381=CARTESIAN_POINT('Ctrl Pts',(-2.09625292867756,1.,-0.120570567965129));
#29382=CARTESIAN_POINT('Ctrl Pts',(-2.10201512132945,-1.,-0.118079107988368));
#29383=CARTESIAN_POINT('Ctrl Pts',(-2.10201512132945,1.,-0.118079107988368));
#29384=CARTESIAN_POINT('Ctrl Pts',(-2.10777050261359,-1.,-0.11554495768794));
#29385=CARTESIAN_POINT('Ctrl Pts',(-2.10777050261359,1.,-0.11554495768794));
#29386=CARTESIAN_POINT('Ctrl Pts',(-2.11351924490335,-1.,-0.112968534419746));
#29387=CARTESIAN_POINT('Ctrl Pts',(-2.11351924490335,1.,-0.112968534419746));
#29388=CARTESIAN_POINT('Ctrl Pts',(-2.11926155590849,-1.,-0.11035023613502));
#29389=CARTESIAN_POINT('Ctrl Pts',(-2.11926155590849,1.,-0.11035023613502));
#29390=CARTESIAN_POINT('Ctrl Pts',(-2.12499752306927,-1.,-0.107690435231068));
#29391=CARTESIAN_POINT('Ctrl Pts',(-2.12499752306927,1.,-0.107690435231068));
#29392=CARTESIAN_POINT('Ctrl Pts',(-2.1307270488718,-1.,-0.104989479152703));
#29393=CARTESIAN_POINT('Ctrl Pts',(-2.1307270488718,1.,-0.104989479152703));
#29394=CARTESIAN_POINT('Ctrl Pts',(-2.13644992667052,-1.,-0.102247700556064));
#29395=CARTESIAN_POINT('Ctrl Pts',(-2.13644992667052,1.,-0.102247700556064));
#29396=CARTESIAN_POINT('Ctrl Pts',(-2.14216588395974,-1.,-0.0994654261990744));
#29397=CARTESIAN_POINT('Ctrl Pts',(-2.14216588395974,1.,-0.0994654261990744));
#29398=CARTESIAN_POINT('Ctrl Pts',(-2.14787463531864,-1.,-0.096642985230569));
#29399=CARTESIAN_POINT('Ctrl Pts',(-2.14787463531864,1.,-0.096642985230569));
#29400=CARTESIAN_POINT('Ctrl Pts',(-2.15357593978377,-1.,-0.0937807218868346));
#29401=CARTESIAN_POINT('Ctrl Pts',(-2.15357593978377,1.,-0.0937807218868346));
#29402=CARTESIAN_POINT('Ctrl Pts',(-2.15926961544808,-1.,-0.0908789888108267));
#29403=CARTESIAN_POINT('Ctrl Pts',(-2.15926961544808,1.,-0.0908789888108267));
#29404=CARTESIAN_POINT('Ctrl Pts',(-2.16495552645275,-1.,-0.0879381291387824));
#29405=CARTESIAN_POINT('Ctrl Pts',(-2.16495552645275,1.,-0.0879381291387824));
#29406=CARTESIAN_POINT('Ctrl Pts',(-2.17063357871031,-1.,-0.0849584620835644));
#29407=CARTESIAN_POINT('Ctrl Pts',(-2.17063357871031,1.,-0.0849584620835644));
#29408=CARTESIAN_POINT('Ctrl Pts',(-2.1763037121106,-1.,-0.0819402680871941));
#29409=CARTESIAN_POINT('Ctrl Pts',(-2.1763037121106,1.,-0.0819402680871941));
#29410=CARTESIAN_POINT('Ctrl Pts',(-2.18196589448304,-1.,-0.0788837727683229));
#29411=CARTESIAN_POINT('Ctrl Pts',(-2.18196589448304,1.,-0.0788837727683229));
#29412=CARTESIAN_POINT('Ctrl Pts',(-2.1876201139874,-1.,-0.0757891465833413));
#29413=CARTESIAN_POINT('Ctrl Pts',(-2.1876201139874,1.,-0.0757891465833413));
#29414=CARTESIAN_POINT('Ctrl Pts',(-2.19213712012956,-1.,-0.0732830357304277));
#29415=CARTESIAN_POINT('Ctrl Pts',(-2.19213712012956,1.,-0.0732830357304277));
#29416=CARTESIAN_POINT('Ctrl Pts',(-2.19552129483562,-1.,-0.0713863779524629));
#29417=CARTESIAN_POINT('Ctrl Pts',(-2.19552129483562,1.,-0.0713863779524629));
#29418=CARTESIAN_POINT('Ctrl Pts',(-2.19777582085261,-1.,-0.0701143536324927));
#29419=CARTESIAN_POINT('Ctrl Pts',(-2.19777582085261,1.,-0.0701143536324927));
#29420=CARTESIAN_POINT('Ctrl Pts',(-2.19890268624765,-1.,-0.0694764450219585));
#29421=CARTESIAN_POINT('Ctrl Pts',(-2.19890268624765,1.,-0.0694764450219585));
#29422=CARTESIAN_POINT('',(-1.74236521665491,1.,-0.163289472382896));
#29423=CARTESIAN_POINT('Ctrl Pts',(-1.74236521665491,1.,-0.163289472382896));
#29424=CARTESIAN_POINT('Ctrl Pts',(-1.74720349503904,1.,-0.163814161002474));
#29425=CARTESIAN_POINT('Ctrl Pts',(-1.75666056640041,1.,-0.164834765708484));
#29426=CARTESIAN_POINT('Ctrl Pts',(-1.77018771687692,1.,-0.166279355148738));
#29427=CARTESIAN_POINT('Ctrl Pts',(-1.78690649988931,1.,-0.16803277280837));
#29428=CARTESIAN_POINT('Ctrl Pts',(-1.80561530633924,1.,-0.169936923908078));
#29429=CARTESIAN_POINT('Ctrl Pts',(-1.82215766815414,1.,-0.171554770207306));
#29430=CARTESIAN_POINT('Ctrl Pts',(-1.83658380530747,1.,-0.17288944289442));
#29431=CARTESIAN_POINT('Ctrl Pts',(-1.84898113200543,1.,-0.173946627589401));
#29432=CARTESIAN_POINT('Ctrl Pts',(-1.85948367089838,1.,-0.174735259276856));
#29433=CARTESIAN_POINT('Ctrl Pts',(-1.86828349694972,1.,-0.175268337590901));
#29434=CARTESIAN_POINT('Ctrl Pts',(-1.87563767773249,1.,-0.175563480746205));
#29435=CARTESIAN_POINT('Ctrl Pts',(-1.88188663144846,1.,-0.175644148889271));
#29436=CARTESIAN_POINT('Ctrl Pts',(-1.88742606272818,1.,-0.175538155840286));
#29437=CARTESIAN_POINT('Ctrl Pts',(-1.89264630198279,1.,-0.175274276190664));
#29438=CARTESIAN_POINT('Ctrl Pts',(-1.89788101117148,1.,-0.174879405091277));
#29439=CARTESIAN_POINT('Ctrl Pts',(-1.90335253863003,1.,-0.174375518661222));
#29440=CARTESIAN_POINT('Ctrl Pts',(-1.90911693975475,1.,-0.173776635257984));
#29441=CARTESIAN_POINT('Ctrl Pts',(-1.91511429159681,1.,-0.173090695383619));
#29442=CARTESIAN_POINT('Ctrl Pts',(-1.92122334398034,1.,-0.172321621259557));
#29443=CARTESIAN_POINT('Ctrl Pts',(-1.92731093582,1.,-0.17147119153296));
#29444=CARTESIAN_POINT('Ctrl Pts',(-1.93329183155455,1.,-0.170541253116136));
#29445=CARTESIAN_POINT('Ctrl Pts',(-1.93915639211497,1.,-0.169534904817425));
#29446=CARTESIAN_POINT('Ctrl Pts',(-1.94493757756879,1.,-0.168455741607516));
#29447=CARTESIAN_POINT('Ctrl Pts',(-1.95069027794286,1.,-0.167307501784469));
#29448=CARTESIAN_POINT('Ctrl Pts',(-1.95646759718755,1.,-0.166093592002833));
#29449=CARTESIAN_POINT('Ctrl Pts',(-1.96229379940174,1.,-0.1648165689203));
#29450=CARTESIAN_POINT('Ctrl Pts',(-1.96816512678,1.,-0.16347818545776));
#29451=CARTESIAN_POINT('Ctrl Pts',(-1.97406280235204,1.,-0.162079693556302));
#29452=CARTESIAN_POINT('Ctrl Pts',(-1.97996195437557,1.,-0.16062206078461));
#29453=CARTESIAN_POINT('Ctrl Pts',(-1.98584238283279,1.,-0.159106226437289));
#29454=CARTESIAN_POINT('Ctrl Pts',(-1.99169810931893,1.,-0.157533331459215));
#29455=CARTESIAN_POINT('Ctrl Pts',(-1.99753284771487,1.,-0.155904629548775));
#29456=CARTESIAN_POINT('Ctrl Pts',(-2.00335565310539,1.,-0.154221403049719));
#29457=CARTESIAN_POINT('Ctrl Pts',(-2.00917680318426,1.,-0.152484883621452));
#29458=CARTESIAN_POINT('Ctrl Pts',(-2.01500291940243,1.,-0.150696157673084));
#29459=CARTESIAN_POINT('Ctrl Pts',(-2.02083464969897,1.,-0.148856124775343));
#29460=CARTESIAN_POINT('Ctrl Pts',(-2.02666926182017,1.,-0.146965557332586));
#29461=CARTESIAN_POINT('Ctrl Pts',(-2.03250223739941,1.,-0.145025140186058));
#29462=CARTESIAN_POINT('Ctrl Pts',(-2.03832911025913,1.,-0.143035515058208));
#29463=CARTESIAN_POINT('Ctrl Pts',(-2.04414757947919,1.,-0.140997332152545));
#29464=CARTESIAN_POINT('Ctrl Pts',(-2.04995762001333,1.,-0.138911255368966));
#29465=CARTESIAN_POINT('Ctrl Pts',(-2.0557604441427,1.,-0.136777941218044));
#29466=CARTESIAN_POINT('Ctrl Pts',(-2.06155781517844,1.,-0.134598026192107));
#29467=CARTESIAN_POINT('Ctrl Pts',(-2.06735123910319,1.,-0.13237211154771));
#29468=CARTESIAN_POINT('Ctrl Pts',(-2.07314114713047,1.,-0.130100748328401));
#29469=CARTESIAN_POINT('Ctrl Pts',(-2.07892715110967,1.,-0.127784445276116));
#29470=CARTESIAN_POINT('Ctrl Pts',(-2.08470840653628,1.,-0.125423679412058));
#29471=CARTESIAN_POINT('Ctrl Pts',(-2.09048392424826,1.,-0.123018905621083));
#29472=CARTESIAN_POINT('Ctrl Pts',(-2.09625292867756,1.,-0.120570567965129));
#29473=CARTESIAN_POINT('Ctrl Pts',(-2.10201512132945,1.,-0.118079107988368));
#29474=CARTESIAN_POINT('Ctrl Pts',(-2.10777050261359,1.,-0.11554495768794));
#29475=CARTESIAN_POINT('Ctrl Pts',(-2.11351924490335,1.,-0.112968534419746));
#29476=CARTESIAN_POINT('Ctrl Pts',(-2.11926155590849,1.,-0.11035023613502));
#29477=CARTESIAN_POINT('Ctrl Pts',(-2.12499752306927,1.,-0.107690435231068));
#29478=CARTESIAN_POINT('Ctrl Pts',(-2.1307270488718,1.,-0.104989479152703));
#29479=CARTESIAN_POINT('Ctrl Pts',(-2.13644992667052,1.,-0.102247700556064));
#29480=CARTESIAN_POINT('Ctrl Pts',(-2.14216588395974,1.,-0.0994654261990744));
#29481=CARTESIAN_POINT('Ctrl Pts',(-2.14787463531864,1.,-0.096642985230569));
#29482=CARTESIAN_POINT('Ctrl Pts',(-2.15357593978377,1.,-0.0937807218868346));
#29483=CARTESIAN_POINT('Ctrl Pts',(-2.15926961544808,1.,-0.0908789888108267));
#29484=CARTESIAN_POINT('Ctrl Pts',(-2.16495552645275,1.,-0.0879381291387824));
#29485=CARTESIAN_POINT('Ctrl Pts',(-2.17063357871031,1.,-0.0849584620835644));
#29486=CARTESIAN_POINT('Ctrl Pts',(-2.1763037121106,1.,-0.0819402680871941));
#29487=CARTESIAN_POINT('Ctrl Pts',(-2.18196589448304,1.,-0.0788837727683229));
#29488=CARTESIAN_POINT('Ctrl Pts',(-2.1876201139874,1.,-0.0757891465833413));
#29489=CARTESIAN_POINT('Ctrl Pts',(-2.19213712012956,1.,-0.0732830357304277));
#29490=CARTESIAN_POINT('Ctrl Pts',(-2.19552129483562,1.,-0.0713863779524629));
#29491=CARTESIAN_POINT('Ctrl Pts',(-2.19777582085261,1.,-0.0701143536324927));
#29492=CARTESIAN_POINT('Ctrl Pts',(-2.19890268624765,1.,-0.0694764450219585));
#29493=CARTESIAN_POINT('',(-1.74236521665491,0.,-0.163289472382896));
#29494=CARTESIAN_POINT('Origin',(0.,0.,0.));
#29495=CARTESIAN_POINT('',(-1.7075470150345,1.,-0.383122945602004));
#29496=CARTESIAN_POINT('Origin',(0.,1.,0.));
#29497=CARTESIAN_POINT('',(-1.7075470150345,0.,-0.383122945602004));
#29498=CARTESIAN_POINT('Ctrl Pts',(-2.11275013067528,-1.,-0.61342227326009));
#29499=CARTESIAN_POINT('Ctrl Pts',(-2.11275013067528,1.,-0.61342227326009));
#29500=CARTESIAN_POINT('Ctrl Pts',(-2.11187554260142,-1.,-0.61246736556225));
#29501=CARTESIAN_POINT('Ctrl Pts',(-2.11187554260142,1.,-0.61246736556225));
#29502=CARTESIAN_POINT('Ctrl Pts',(-2.11012443807661,-1.,-0.610560911691113));
#29503=CARTESIAN_POINT('Ctrl Pts',(-2.11012443807661,1.,-0.610560911691113));
#29504=CARTESIAN_POINT('Ctrl Pts',(-2.10749199615859,-1.,-0.607711315456826));
#29505=CARTESIAN_POINT('Ctrl Pts',(-2.10749199615859,1.,-0.607711315456826));
#29506=CARTESIAN_POINT('Ctrl Pts',(-2.10397049887709,-1.,-0.603932030738212));
#29507=CARTESIAN_POINT('Ctrl Pts',(-2.10397049887709,1.,-0.603932030738212));
#29508=CARTESIAN_POINT('Ctrl Pts',(-2.09954930865331,-1.,-0.599241616422144));
#29509=CARTESIAN_POINT('Ctrl Pts',(-2.09954930865331,1.,-0.599241616422144));
#29510=CARTESIAN_POINT('Ctrl Pts',(-2.09510876220501,-1.,-0.594585006052823));
#29511=CARTESIAN_POINT('Ctrl Pts',(-2.09510876220501,1.,-0.594585006052823));
#29512=CARTESIAN_POINT('Ctrl Pts',(-2.09064881812053,-1.,-0.589962365403189));
#29513=CARTESIAN_POINT('Ctrl Pts',(-2.09064881812053,1.,-0.589962365403189));
#29514=CARTESIAN_POINT('Ctrl Pts',(-2.086169437277,-1.,-0.585373918990895));
#29515=CARTESIAN_POINT('Ctrl Pts',(-2.086169437277,1.,-0.585373918990895));
#29516=CARTESIAN_POINT('Ctrl Pts',(-2.08167059018138,-1.,-0.580819952107257));
#29517=CARTESIAN_POINT('Ctrl Pts',(-2.08167059018138,1.,-0.580819952107257));
#29518=CARTESIAN_POINT('Ctrl Pts',(-2.07715226767361,-1.,-0.576300797416274));
#29519=CARTESIAN_POINT('Ctrl Pts',(-2.07715226767361,1.,-0.576300797416274));
#29520=CARTESIAN_POINT('Ctrl Pts',(-2.07261449292757,-1.,-0.571816823242411));
#29521=CARTESIAN_POINT('Ctrl Pts',(-2.07261449292757,1.,-0.571816823242411));
#29522=CARTESIAN_POINT('Ctrl Pts',(-2.06805732997383,-1.,-0.567368421181229));
#29523=CARTESIAN_POINT('Ctrl Pts',(-2.06805732997383,1.,-0.567368421181229));
#29524=CARTESIAN_POINT('Ctrl Pts',(-2.06348090160697,-1.,-0.562955993082574));
#29525=CARTESIAN_POINT('Ctrl Pts',(-2.06348090160697,1.,-0.562955993082574));
#29526=CARTESIAN_POINT('Ctrl Pts',(-2.05888537756571,-1.,-0.558579940185467));
#29527=CARTESIAN_POINT('Ctrl Pts',(-2.05888537756571,1.,-0.558579940185467));
#29528=CARTESIAN_POINT('Ctrl Pts',(-2.05427091604482,-1.,-0.554240657464109));
#29529=CARTESIAN_POINT('Ctrl Pts',(-2.05427091604482,1.,-0.554240657464109));
#29530=CARTESIAN_POINT('Ctrl Pts',(-2.04963761077974,-1.,-0.549938525150342));
#29531=CARTESIAN_POINT('Ctrl Pts',(-2.04963761077974,1.,-0.549938525150342));
#29532=CARTESIAN_POINT('Ctrl Pts',(-2.0449854471456,-1.,-0.545673903817348));
#29533=CARTESIAN_POINT('Ctrl Pts',(-2.0449854471456,1.,-0.545673903817348));
#29534=CARTESIAN_POINT('Ctrl Pts',(-2.0403142269048,-1.,-0.54144712061552));
#29535=CARTESIAN_POINT('Ctrl Pts',(-2.0403142269048,1.,-0.54144712061552));
#29536=CARTESIAN_POINT('Ctrl Pts',(-2.03562362953993,-1.,-0.537258489833134));
#29537=CARTESIAN_POINT('Ctrl Pts',(-2.03562362953993,1.,-0.537258489833134));
#29538=CARTESIAN_POINT('Ctrl Pts',(-2.03091336214401,-1.,-0.533108355132905));
#29539=CARTESIAN_POINT('Ctrl Pts',(-2.03091336214401,1.,-0.533108355132905));
#29540=CARTESIAN_POINT('Ctrl Pts',(-2.02618329083289,-1.,-0.52899712724191));
#29541=CARTESIAN_POINT('Ctrl Pts',(-2.02618329083289,1.,-0.52899712724191));
#29542=CARTESIAN_POINT('Ctrl Pts',(-2.02143356304712,-1.,-0.524925318333518));
#29543=CARTESIAN_POINT('Ctrl Pts',(-2.02143356304712,1.,-0.524925318333518));
#29544=CARTESIAN_POINT('Ctrl Pts',(-2.01666477917305,-1.,-0.520893590399428));
#29545=CARTESIAN_POINT('Ctrl Pts',(-2.01666477917305,1.,-0.520893590399428));
#29546=CARTESIAN_POINT('Ctrl Pts',(-2.01187773939257,-1.,-0.516902681728733));
#29547=CARTESIAN_POINT('Ctrl Pts',(-2.01187773939257,1.,-0.516902681728733));
#29548=CARTESIAN_POINT('Ctrl Pts',(-2.00707309946955,-1.,-0.512953306961813));
#29549=CARTESIAN_POINT('Ctrl Pts',(-2.00707309946955,1.,-0.512953306961813));
#29550=CARTESIAN_POINT('Ctrl Pts',(-2.00225107134733,-1.,-0.509046069886152));
#29551=CARTESIAN_POINT('Ctrl Pts',(-2.00225107134733,1.,-0.509046069886152));
#29552=CARTESIAN_POINT('Ctrl Pts',(-1.99741107463567,-1.,-0.505181361323011));
#29553=CARTESIAN_POINT('Ctrl Pts',(-1.99741107463567,1.,-0.505181361323011));
#29554=CARTESIAN_POINT('Ctrl Pts',(-1.9925514912615,-1.,-0.501359287727129));
#29555=CARTESIAN_POINT('Ctrl Pts',(-1.9925514912615,1.,-0.501359287727129));
#29556=CARTESIAN_POINT('Ctrl Pts',(-1.98767044752929,-1.,-0.497579909545564));
#29557=CARTESIAN_POINT('Ctrl Pts',(-1.98767044752929,1.,-0.497579909545564));
#29558=CARTESIAN_POINT('Ctrl Pts',(-1.9827665876182,-1.,-0.493843476541492));
#29559=CARTESIAN_POINT('Ctrl Pts',(-1.9827665876182,1.,-0.493843476541492));
#29560=CARTESIAN_POINT('Ctrl Pts',(-1.97783973019229,-1.,-0.490150627860955));
#29561=CARTESIAN_POINT('Ctrl Pts',(-1.97783973019229,1.,-0.490150627860955));
#29562=CARTESIAN_POINT('Ctrl Pts',(-1.97289186263272,-1.,-0.486502692907661));
#29563=CARTESIAN_POINT('Ctrl Pts',(-1.97289186263272,1.,-0.486502692907661));
#29564=CARTESIAN_POINT('Ctrl Pts',(-1.96792703422358,-1.,-0.482901662120686));
#29565=CARTESIAN_POINT('Ctrl Pts',(-1.96792703422358,1.,-0.482901662120686));
#29566=CARTESIAN_POINT('Ctrl Pts',(-1.96294933055938,-1.,-0.479349583074846));
#29567=CARTESIAN_POINT('Ctrl Pts',(-1.96294933055938,1.,-0.479349583074846));
#29568=CARTESIAN_POINT('Ctrl Pts',(-1.95796111148175,-1.,-0.475848034683171));
#29569=CARTESIAN_POINT('Ctrl Pts',(-1.95796111148175,1.,-0.475848034683171));
#29570=CARTESIAN_POINT('Ctrl Pts',(-1.95296148278136,-1.,-0.472397672264079));
#29571=CARTESIAN_POINT('Ctrl Pts',(-1.95296148278136,1.,-0.472397672264079));
#29572=CARTESIAN_POINT('Ctrl Pts',(-1.94794381136524,-1.,-0.468997482913158));
#29573=CARTESIAN_POINT('Ctrl Pts',(-1.94794381136524,1.,-0.468997482913158));
#29574=CARTESIAN_POINT('Ctrl Pts',(-1.94289794196205,-1.,-0.465645462026064));
#29575=CARTESIAN_POINT('Ctrl Pts',(-1.94289794196205,1.,-0.465645462026064));
#29576=CARTESIAN_POINT('Ctrl Pts',(-1.93781486640834,-1.,-0.462340031009087));
#29577=CARTESIAN_POINT('Ctrl Pts',(-1.93781486640834,1.,-0.462340031009087));
#29578=CARTESIAN_POINT('Ctrl Pts',(-1.93269066517936,-1.,-0.459081234547931));
#29579=CARTESIAN_POINT('Ctrl Pts',(-1.93269066517936,1.,-0.459081234547931));
#29580=CARTESIAN_POINT('Ctrl Pts',(-1.92753067150461,-1.,-0.455872005174335));
#29581=CARTESIAN_POINT('Ctrl Pts',(-1.92753067150461,1.,-0.455872005174335));
#29582=CARTESIAN_POINT('Ctrl Pts',(-1.9223538064847,-1.,-0.452719478359356));
#29583=CARTESIAN_POINT('Ctrl Pts',(-1.9223538064847,1.,-0.452719478359356));
#29584=CARTESIAN_POINT('Ctrl Pts',(-1.91718342555717,-1.,-0.449632260106572));
#29585=CARTESIAN_POINT('Ctrl Pts',(-1.91718342555717,1.,-0.449632260106572));
#29586=CARTESIAN_POINT('Ctrl Pts',(-1.91203699981095,-1.,-0.446617343485651));
#29587=CARTESIAN_POINT('Ctrl Pts',(-1.91203699981095,1.,-0.446617343485651));
#29588=CARTESIAN_POINT('Ctrl Pts',(-1.90691756144906,-1.,-0.44367755684917));
#29589=CARTESIAN_POINT('Ctrl Pts',(-1.90691756144906,1.,-0.44367755684917));
#29590=CARTESIAN_POINT('Ctrl Pts',(-1.90180124389137,-1.,-0.44080783370416));
#29591=CARTESIAN_POINT('Ctrl Pts',(-1.90180124389137,1.,-0.44080783370416));
#29592=CARTESIAN_POINT('Ctrl Pts',(-1.89663648956549,-1.,-0.437995003948443));
#29593=CARTESIAN_POINT('Ctrl Pts',(-1.89663648956549,1.,-0.437995003948443));
#29594=CARTESIAN_POINT('Ctrl Pts',(-1.89136993975585,-1.,-0.43522566096358));
#29595=CARTESIAN_POINT('Ctrl Pts',(-1.89136993975585,1.,-0.43522566096358));
#29596=CARTESIAN_POINT('Ctrl Pts',(-1.88596913666828,-1.,-0.432493038548833));
#29597=CARTESIAN_POINT('Ctrl Pts',(-1.88596913666828,1.,-0.432493038548833));
#29598=CARTESIAN_POINT('Ctrl Pts',(-1.88044229001778,-1.,-0.429803062482217));
#29599=CARTESIAN_POINT('Ctrl Pts',(-1.88044229001778,1.,-0.429803062482217));
#29600=CARTESIAN_POINT('Ctrl Pts',(-1.87486989291333,-1.,-0.427183828518743));
#29601=CARTESIAN_POINT('Ctrl Pts',(-1.87486989291333,1.,-0.427183828518743));
#29602=CARTESIAN_POINT('Ctrl Pts',(-1.8693780394412,-1.,-0.424678177290876));
#29603=CARTESIAN_POINT('Ctrl Pts',(-1.8693780394412,1.,-0.424678177290876));
#29604=CARTESIAN_POINT('Ctrl Pts',(-1.86408083333863,-1.,-0.422327307417884));
#29605=CARTESIAN_POINT('Ctrl Pts',(-1.86408083333863,1.,-0.422327307417884));
#29606=CARTESIAN_POINT('Ctrl Pts',(-1.8590328109667,-1.,-0.420157287975583));
#29607=CARTESIAN_POINT('Ctrl Pts',(-1.8590328109667,1.,-0.420157287975583));
#29608=CARTESIAN_POINT('Ctrl Pts',(-1.8541763285645,-1.,-0.418164129144045));
#29609=CARTESIAN_POINT('Ctrl Pts',(-1.8541763285645,1.,-0.418164129144045));
#29610=CARTESIAN_POINT('Ctrl Pts',(-1.84929312930314,-1.,-0.416300022039885));
#29611=CARTESIAN_POINT('Ctrl Pts',(-1.84929312930314,1.,-0.416300022039885));
#29612=CARTESIAN_POINT('Ctrl Pts',(-1.84405757074218,-1.,-0.414487438255542));
#29613=CARTESIAN_POINT('Ctrl Pts',(-1.84405757074218,1.,-0.414487438255542));
#29614=CARTESIAN_POINT('Ctrl Pts',(-1.8380895347617,-1.,-0.412633125322945));
#29615=CARTESIAN_POINT('Ctrl Pts',(-1.8380895347617,1.,-0.412633125322945));
#29616=CARTESIAN_POINT('Ctrl Pts',(-1.83100408895047,-1.,-0.410641256301276));
#29617=CARTESIAN_POINT('Ctrl Pts',(-1.83100408895047,1.,-0.410641256301276));
#29618=CARTESIAN_POINT('Ctrl Pts',(-1.82247022677562,-1.,-0.408428948106227));
#29619=CARTESIAN_POINT('Ctrl Pts',(-1.82247022677562,1.,-0.408428948106227));
#29620=CARTESIAN_POINT('Ctrl Pts',(-1.81223801812013,-1.,-0.405933518407175));
#29621=CARTESIAN_POINT('Ctrl Pts',(-1.81223801812013,1.,-0.405933518407175));
#29622=CARTESIAN_POINT('Ctrl Pts',(-1.80012077173238,-1.,-0.403107976163396));
#29623=CARTESIAN_POINT('Ctrl Pts',(-1.80012077173238,1.,-0.403107976163396));
#29624=CARTESIAN_POINT('Ctrl Pts',(-1.78598826343754,-1.,-0.399919403774155));
#29625=CARTESIAN_POINT('Ctrl Pts',(-1.78598826343754,1.,-0.399919403774155));
#29626=CARTESIAN_POINT('Ctrl Pts',(-1.76975560043442,-1.,-0.396346196110688));
#29627=CARTESIAN_POINT('Ctrl Pts',(-1.76975560043442,1.,-0.396346196110688));
#29628=CARTESIAN_POINT('Ctrl Pts',(-1.75137405310193,-1.,-0.392375812285395));
#29629=CARTESIAN_POINT('Ctrl Pts',(-1.75137405310193,1.,-0.392375812285395));
#29630=CARTESIAN_POINT('Ctrl Pts',(-1.73493170972829,-1.,-0.388877023502615));
#29631=CARTESIAN_POINT('Ctrl Pts',(-1.73493170972829,1.,-0.388877023502615));
#29632=CARTESIAN_POINT('Ctrl Pts',(-1.72162022244582,-1.,-0.386070790323281));
#29633=CARTESIAN_POINT('Ctrl Pts',(-1.72162022244582,1.,-0.386070790323281));
#29634=CARTESIAN_POINT('Ctrl Pts',(-1.71231062891398,-1.,-0.384119047314215));
#29635=CARTESIAN_POINT('Ctrl Pts',(-1.71231062891398,1.,-0.384119047314215));
#29636=CARTESIAN_POINT('Ctrl Pts',(-1.7075470150345,-1.,-0.383122945602004));
#29637=CARTESIAN_POINT('Ctrl Pts',(-1.7075470150345,1.,-0.383122945602004));
#29638=CARTESIAN_POINT('',(-2.11275013067528,1.,-0.61342227326009));
#29639=CARTESIAN_POINT('Ctrl Pts',(-2.11275013067528,1.,-0.61342227326009));
#29640=CARTESIAN_POINT('Ctrl Pts',(-2.11187554260142,1.,-0.61246736556225));
#29641=CARTESIAN_POINT('Ctrl Pts',(-2.11012443807661,1.,-0.610560911691113));
#29642=CARTESIAN_POINT('Ctrl Pts',(-2.10749199615859,1.,-0.607711315456826));
#29643=CARTESIAN_POINT('Ctrl Pts',(-2.10397049887709,1.,-0.603932030738212));
#29644=CARTESIAN_POINT('Ctrl Pts',(-2.09954930865331,1.,-0.599241616422144));
#29645=CARTESIAN_POINT('Ctrl Pts',(-2.09510876220501,1.,-0.594585006052823));
#29646=CARTESIAN_POINT('Ctrl Pts',(-2.09064881812053,1.,-0.589962365403189));
#29647=CARTESIAN_POINT('Ctrl Pts',(-2.086169437277,1.,-0.585373918990895));
#29648=CARTESIAN_POINT('Ctrl Pts',(-2.08167059018138,1.,-0.580819952107257));
#29649=CARTESIAN_POINT('Ctrl Pts',(-2.07715226767361,1.,-0.576300797416274));
#29650=CARTESIAN_POINT('Ctrl Pts',(-2.07261449292757,1.,-0.571816823242411));
#29651=CARTESIAN_POINT('Ctrl Pts',(-2.06805732997383,1.,-0.567368421181229));
#29652=CARTESIAN_POINT('Ctrl Pts',(-2.06348090160697,1.,-0.562955993082574));
#29653=CARTESIAN_POINT('Ctrl Pts',(-2.05888537756571,1.,-0.558579940185467));
#29654=CARTESIAN_POINT('Ctrl Pts',(-2.05427091604482,1.,-0.554240657464109));
#29655=CARTESIAN_POINT('Ctrl Pts',(-2.04963761077974,1.,-0.549938525150342));
#29656=CARTESIAN_POINT('Ctrl Pts',(-2.0449854471456,1.,-0.545673903817348));
#29657=CARTESIAN_POINT('Ctrl Pts',(-2.0403142269048,1.,-0.54144712061552));
#29658=CARTESIAN_POINT('Ctrl Pts',(-2.03562362953993,1.,-0.537258489833134));
#29659=CARTESIAN_POINT('Ctrl Pts',(-2.03091336214401,1.,-0.533108355132905));
#29660=CARTESIAN_POINT('Ctrl Pts',(-2.02618329083289,1.,-0.52899712724191));
#29661=CARTESIAN_POINT('Ctrl Pts',(-2.02143356304712,1.,-0.524925318333518));
#29662=CARTESIAN_POINT('Ctrl Pts',(-2.01666477917305,1.,-0.520893590399428));
#29663=CARTESIAN_POINT('Ctrl Pts',(-2.01187773939257,1.,-0.516902681728733));
#29664=CARTESIAN_POINT('Ctrl Pts',(-2.00707309946955,1.,-0.512953306961813));
#29665=CARTESIAN_POINT('Ctrl Pts',(-2.00225107134733,1.,-0.509046069886152));
#29666=CARTESIAN_POINT('Ctrl Pts',(-1.99741107463567,1.,-0.505181361323011));
#29667=CARTESIAN_POINT('Ctrl Pts',(-1.9925514912615,1.,-0.501359287727129));
#29668=CARTESIAN_POINT('Ctrl Pts',(-1.98767044752929,1.,-0.497579909545564));
#29669=CARTESIAN_POINT('Ctrl Pts',(-1.9827665876182,1.,-0.493843476541492));
#29670=CARTESIAN_POINT('Ctrl Pts',(-1.97783973019229,1.,-0.490150627860955));
#29671=CARTESIAN_POINT('Ctrl Pts',(-1.97289186263272,1.,-0.486502692907661));
#29672=CARTESIAN_POINT('Ctrl Pts',(-1.96792703422358,1.,-0.482901662120686));
#29673=CARTESIAN_POINT('Ctrl Pts',(-1.96294933055938,1.,-0.479349583074846));
#29674=CARTESIAN_POINT('Ctrl Pts',(-1.95796111148175,1.,-0.475848034683171));
#29675=CARTESIAN_POINT('Ctrl Pts',(-1.95296148278136,1.,-0.472397672264079));
#29676=CARTESIAN_POINT('Ctrl Pts',(-1.94794381136524,1.,-0.468997482913158));
#29677=CARTESIAN_POINT('Ctrl Pts',(-1.94289794196205,1.,-0.465645462026064));
#29678=CARTESIAN_POINT('Ctrl Pts',(-1.93781486640834,1.,-0.462340031009087));
#29679=CARTESIAN_POINT('Ctrl Pts',(-1.93269066517936,1.,-0.459081234547931));
#29680=CARTESIAN_POINT('Ctrl Pts',(-1.92753067150461,1.,-0.455872005174335));
#29681=CARTESIAN_POINT('Ctrl Pts',(-1.9223538064847,1.,-0.452719478359356));
#29682=CARTESIAN_POINT('Ctrl Pts',(-1.91718342555717,1.,-0.449632260106572));
#29683=CARTESIAN_POINT('Ctrl Pts',(-1.91203699981095,1.,-0.446617343485651));
#29684=CARTESIAN_POINT('Ctrl Pts',(-1.90691756144906,1.,-0.44367755684917));
#29685=CARTESIAN_POINT('Ctrl Pts',(-1.90180124389137,1.,-0.44080783370416));
#29686=CARTESIAN_POINT('Ctrl Pts',(-1.89663648956549,1.,-0.437995003948443));
#29687=CARTESIAN_POINT('Ctrl Pts',(-1.89136993975585,1.,-0.43522566096358));
#29688=CARTESIAN_POINT('Ctrl Pts',(-1.88596913666828,1.,-0.432493038548833));
#29689=CARTESIAN_POINT('Ctrl Pts',(-1.88044229001778,1.,-0.429803062482217));
#29690=CARTESIAN_POINT('Ctrl Pts',(-1.87486989291333,1.,-0.427183828518743));
#29691=CARTESIAN_POINT('Ctrl Pts',(-1.8693780394412,1.,-0.424678177290876));
#29692=CARTESIAN_POINT('Ctrl Pts',(-1.86408083333863,1.,-0.422327307417884));
#29693=CARTESIAN_POINT('Ctrl Pts',(-1.8590328109667,1.,-0.420157287975583));
#29694=CARTESIAN_POINT('Ctrl Pts',(-1.8541763285645,1.,-0.418164129144045));
#29695=CARTESIAN_POINT('Ctrl Pts',(-1.84929312930314,1.,-0.416300022039885));
#29696=CARTESIAN_POINT('Ctrl Pts',(-1.84405757074218,1.,-0.414487438255542));
#29697=CARTESIAN_POINT('Ctrl Pts',(-1.8380895347617,1.,-0.412633125322945));
#29698=CARTESIAN_POINT('Ctrl Pts',(-1.83100408895047,1.,-0.410641256301276));
#29699=CARTESIAN_POINT('Ctrl Pts',(-1.82247022677562,1.,-0.408428948106227));
#29700=CARTESIAN_POINT('Ctrl Pts',(-1.81223801812013,1.,-0.405933518407175));
#29701=CARTESIAN_POINT('Ctrl Pts',(-1.80012077173238,1.,-0.403107976163396));
#29702=CARTESIAN_POINT('Ctrl Pts',(-1.78598826343754,1.,-0.399919403774155));
#29703=CARTESIAN_POINT('Ctrl Pts',(-1.76975560043442,1.,-0.396346196110688));
#29704=CARTESIAN_POINT('Ctrl Pts',(-1.75137405310193,1.,-0.392375812285395));
#29705=CARTESIAN_POINT('Ctrl Pts',(-1.73493170972829,1.,-0.388877023502615));
#29706=CARTESIAN_POINT('Ctrl Pts',(-1.72162022244582,1.,-0.386070790323281));
#29707=CARTESIAN_POINT('Ctrl Pts',(-1.71231062891398,1.,-0.384119047314215));
#29708=CARTESIAN_POINT('Ctrl Pts',(-1.7075470150345,1.,-0.383122945602004));
#29709=CARTESIAN_POINT('',(-2.11275013067528,0.,-0.61342227326009));
#29710=CARTESIAN_POINT('Origin',(-2.0698113262342,0.,-0.745574324794401));
#29711=CARTESIAN_POINT('',(-2.0698113262342,1.,-0.745574324794401));
#29712=CARTESIAN_POINT('',(-2.11275013067528,1.,-0.61342227326009));
#29713=CARTESIAN_POINT('',(-2.0698113262342,0.,-0.745574324794401));
#29714=CARTESIAN_POINT('Ctrl Pts',(-1.60662857109684,-1.,-0.693717979106306));
#29715=CARTESIAN_POINT('Ctrl Pts',(-1.60662857109684,1.,-0.693717979106306));
#29716=CARTESIAN_POINT('Ctrl Pts',(-1.61106790958151,-1.,-0.695712097881194));
#29717=CARTESIAN_POINT('Ctrl Pts',(-1.61106790958151,1.,-0.695712097881194));
#29718=CARTESIAN_POINT('Ctrl Pts',(-1.61974673472612,-1.,-0.699605146405088));
#29719=CARTESIAN_POINT('Ctrl Pts',(-1.61974673472612,1.,-0.699605146405088));
#29720=CARTESIAN_POINT('Ctrl Pts',(-1.63216541664676,-1.,-0.705159151988319));
#29721=CARTESIAN_POINT('Ctrl Pts',(-1.63216541664676,1.,-0.705159151988319));
#29722=CARTESIAN_POINT('Ctrl Pts',(-1.64752408832016,-1.,-0.711993139355394));
#29723=CARTESIAN_POINT('Ctrl Pts',(-1.64752408832016,1.,-0.711993139355394));
#29724=CARTESIAN_POINT('Ctrl Pts',(-1.6647288055568,-1.,-0.719585433804282));
#29725=CARTESIAN_POINT('Ctrl Pts',(-1.6647288055568,1.,-0.719585433804282));
#29726=CARTESIAN_POINT('Ctrl Pts',(-1.67996158455503,-1.,-0.726235967997433));
#29727=CARTESIAN_POINT('Ctrl Pts',(-1.67996158455503,1.,-0.726235967997433));
#29728=CARTESIAN_POINT('Ctrl Pts',(-1.69326921975743,-1.,-0.731963238697195));
#29729=CARTESIAN_POINT('Ctrl Pts',(-1.69326921975743,1.,-0.731963238697195));
#29730=CARTESIAN_POINT('Ctrl Pts',(-1.70473309006121,-1.,-0.736799665724771));
#29731=CARTESIAN_POINT('Ctrl Pts',(-1.70473309006121,1.,-0.736799665724771));
#29732=CARTESIAN_POINT('Ctrl Pts',(-1.71447789751927,-1.,-0.740795162032087));
#29733=CARTESIAN_POINT('Ctrl Pts',(-1.71447789751927,1.,-0.740795162032087));
#29734=CARTESIAN_POINT('Ctrl Pts',(-1.7226822991693,-1.,-0.744021445433764));
#29735=CARTESIAN_POINT('Ctrl Pts',(-1.7226822991693,1.,-0.744021445433764));
#29736=CARTESIAN_POINT('Ctrl Pts',(-1.72958533647399,-1.,-0.746574710096436));
#29737=CARTESIAN_POINT('Ctrl Pts',(-1.72958533647399,1.,-0.746574710096436));
#29738=CARTESIAN_POINT('Ctrl Pts',(-1.73550351679848,-1.,-0.748582462954854));
#29739=CARTESIAN_POINT('Ctrl Pts',(-1.73550351679848,1.,-0.748582462954854));
#29740=CARTESIAN_POINT('Ctrl Pts',(-1.74080458266705,-1.,-0.75019343597954));
#29741=CARTESIAN_POINT('Ctrl Pts',(-1.74080458266705,1.,-0.75019343597954));
#29742=CARTESIAN_POINT('Ctrl Pts',(-1.74585086852298,-1.,-0.751555614163629));
#29743=CARTESIAN_POINT('Ctrl Pts',(-1.74585086852298,1.,-0.751555614163629));
#29744=CARTESIAN_POINT('Ctrl Pts',(-1.75095139468809,-1.,-0.752797683531377));
#29745=CARTESIAN_POINT('Ctrl Pts',(-1.75095139468809,1.,-0.752797683531377));
#29746=CARTESIAN_POINT('Ctrl Pts',(-1.75631083600175,-1.,-0.75400925402848));
#29747=CARTESIAN_POINT('Ctrl Pts',(-1.75631083600175,1.,-0.75400925402848));
#29748=CARTESIAN_POINT('Ctrl Pts',(-1.7619781724032,-1.,-0.755220979975262));
#29749=CARTESIAN_POINT('Ctrl Pts',(-1.7619781724032,1.,-0.755220979975262));
#29750=CARTESIAN_POINT('Ctrl Pts',(-1.76789396003141,-1.,-0.756421896028403));
#29751=CARTESIAN_POINT('Ctrl Pts',(-1.76789396003141,1.,-0.756421896028403));
#29752=CARTESIAN_POINT('Ctrl Pts',(-1.77394167108342,-1.,-0.757578264077238));
#29753=CARTESIAN_POINT('Ctrl Pts',(-1.77394167108342,1.,-0.757578264077238));
#29754=CARTESIAN_POINT('Ctrl Pts',(-1.77999411220912,-1.,-0.75865062667738));
#29755=CARTESIAN_POINT('Ctrl Pts',(-1.77999411220912,1.,-0.75865062667738));
#29756=CARTESIAN_POINT('Ctrl Pts',(-1.78596964884526,-1.,-0.759614401109868));
#29757=CARTESIAN_POINT('Ctrl Pts',(-1.78596964884526,1.,-0.759614401109868));
#29758=CARTESIAN_POINT('Ctrl Pts',(-1.79185815610802,-1.,-0.760469555880425));
#29759=CARTESIAN_POINT('Ctrl Pts',(-1.79185815610802,1.,-0.760469555880425));
#29760=CARTESIAN_POINT('Ctrl Pts',(-1.79768986997735,-1.,-0.761229695230359));
#29761=CARTESIAN_POINT('Ctrl Pts',(-1.79768986997735,1.,-0.761229695230359));
#29762=CARTESIAN_POINT('Ctrl Pts',(-1.80351583877334,-1.,-0.761915336443515));
#29763=CARTESIAN_POINT('Ctrl Pts',(-1.80351583877334,1.,-0.761915336443515));
#29764=CARTESIAN_POINT('Ctrl Pts',(-1.80938551463989,-1.,-0.762546129464036));
#29765=CARTESIAN_POINT('Ctrl Pts',(-1.80938551463989,1.,-0.762546129464036));
#29766=CARTESIAN_POINT('Ctrl Pts',(-1.81532118405566,-1.,-0.763132003836783));
#29767=CARTESIAN_POINT('Ctrl Pts',(-1.81532118405566,1.,-0.763132003836783));
#29768=CARTESIAN_POINT('Ctrl Pts',(-1.82131873145297,-1.,-0.763673465462854));
#29769=CARTESIAN_POINT('Ctrl Pts',(-1.82131873145297,1.,-0.763673465462854));
#29770=CARTESIAN_POINT('Ctrl Pts',(-1.8273599120008,-1.,-0.764165902606055));
#29771=CARTESIAN_POINT('Ctrl Pts',(-1.8273599120008,1.,-0.764165902606055));
#29772=CARTESIAN_POINT('Ctrl Pts',(-1.8334207722714,-1.,-0.764602549687845));
#29773=CARTESIAN_POINT('Ctrl Pts',(-1.8334207722714,1.,-0.764602549687845));
#29774=CARTESIAN_POINT('Ctrl Pts',(-1.83948181064823,-1.,-0.764978057881687));
#29775=CARTESIAN_POINT('Ctrl Pts',(-1.83948181064823,1.,-0.764978057881687));
#29776=CARTESIAN_POINT('Ctrl Pts',(-1.8455369887591,-1.,-0.765291664861971));
#29777=CARTESIAN_POINT('Ctrl Pts',(-1.8455369887591,1.,-0.765291664861971));
#29778=CARTESIAN_POINT('Ctrl Pts',(-1.85158945130054,-1.,-0.765545710619023));
#29779=CARTESIAN_POINT('Ctrl Pts',(-1.85158945130054,1.,-0.765545710619023));
#29780=CARTESIAN_POINT('Ctrl Pts',(-1.85764741390391,-1.,-0.765744212909305));
#29781=CARTESIAN_POINT('Ctrl Pts',(-1.85764741390391,1.,-0.765744212909305));
#29782=CARTESIAN_POINT('Ctrl Pts',(-1.86372027063314,-1.,-0.765891519092557));
#29783=CARTESIAN_POINT('Ctrl Pts',(-1.86372027063314,1.,-0.765891519092557));
#29784=CARTESIAN_POINT('Ctrl Pts',(-1.86981398314345,-1.,-0.765990708546111));
#29785=CARTESIAN_POINT('Ctrl Pts',(-1.86981398314345,1.,-0.765990708546111));
#29786=CARTESIAN_POINT('Ctrl Pts',(-1.87592888967886,-1.,-0.766042837036759));
#29787=CARTESIAN_POINT('Ctrl Pts',(-1.87592888967886,1.,-0.766042837036759));
#29788=CARTESIAN_POINT('Ctrl Pts',(-1.88206215302561,-1.,-0.766047794851868));
#29789=CARTESIAN_POINT('Ctrl Pts',(-1.88206215302561,1.,-0.766047794851868));
#29790=CARTESIAN_POINT('Ctrl Pts',(-1.88820926433409,-1.,-0.76600483706209));
#29791=CARTESIAN_POINT('Ctrl Pts',(-1.88820926433409,1.,-0.76600483706209));
#29792=CARTESIAN_POINT('Ctrl Pts',(-1.89436577771389,-1.,-0.765913193856979));
#29793=CARTESIAN_POINT('Ctrl Pts',(-1.89436577771389,1.,-0.765913193856979));
#29794=CARTESIAN_POINT('Ctrl Pts',(-1.90052930393599,-1.,-0.765772772593395));
#29795=CARTESIAN_POINT('Ctrl Pts',(-1.90052930393599,1.,-0.765772772593395));
#29796=CARTESIAN_POINT('Ctrl Pts',(-1.90669961402362,-1.,-0.765584196937936));
#29797=CARTESIAN_POINT('Ctrl Pts',(-1.90669961402362,1.,-0.765584196937936));
#29798=CARTESIAN_POINT('Ctrl Pts',(-1.91287765805174,-1.,-0.765348465884739));
#29799=CARTESIAN_POINT('Ctrl Pts',(-1.91287765805174,1.,-0.765348465884739));
#29800=CARTESIAN_POINT('Ctrl Pts',(-1.91906491634197,-1.,-0.765066729667095));
#29801=CARTESIAN_POINT('Ctrl Pts',(-1.91906491634197,1.,-0.765066729667095));
#29802=CARTESIAN_POINT('Ctrl Pts',(-1.92526263537041,-1.,-0.764740025488189));
#29803=CARTESIAN_POINT('Ctrl Pts',(-1.92526263537041,1.,-0.764740025488189));
#29804=CARTESIAN_POINT('Ctrl Pts',(-1.93147105496367,-1.,-0.764369010673889));
#29805=CARTESIAN_POINT('Ctrl Pts',(-1.93147105496367,1.,-0.764369010673889));
#29806=CARTESIAN_POINT('Ctrl Pts',(-1.93768964875867,-1.,-0.763954049121393));
#29807=CARTESIAN_POINT('Ctrl Pts',(-1.93768964875867,1.,-0.763954049121393));
#29808=CARTESIAN_POINT('Ctrl Pts',(-1.94391746617626,-1.,-0.76349533353858));
#29809=CARTESIAN_POINT('Ctrl Pts',(-1.94391746617626,1.,-0.76349533353858));
#29810=CARTESIAN_POINT('Ctrl Pts',(-1.95015342590025,-1.,-0.762992990878774));
#29811=CARTESIAN_POINT('Ctrl Pts',(-1.95015342590025,1.,-0.762992990878774));
#29812=CARTESIAN_POINT('Ctrl Pts',(-1.95639665309893,-1.,-0.762447203806263));
#29813=CARTESIAN_POINT('Ctrl Pts',(-1.95639665309893,1.,-0.762447203806263));
#29814=CARTESIAN_POINT('Ctrl Pts',(-1.96264672744229,-1.,-0.761858300014575));
#29815=CARTESIAN_POINT('Ctrl Pts',(-1.96264672744229,1.,-0.761858300014575));
#29816=CARTESIAN_POINT('Ctrl Pts',(-1.96890351582545,-1.,-0.761226690483986));
#29817=CARTESIAN_POINT('Ctrl Pts',(-1.96890351582545,1.,-0.761226690483986));
#29818=CARTESIAN_POINT('Ctrl Pts',(-1.97516705321521,-1.,-0.760552825409855));
#29819=CARTESIAN_POINT('Ctrl Pts',(-1.97516705321521,1.,-0.760552825409855));
#29820=CARTESIAN_POINT('Ctrl Pts',(-1.98143741418156,-1.,-0.759837147452135));
#29821=CARTESIAN_POINT('Ctrl Pts',(-1.98143741418156,1.,-0.759837147452135));
#29822=CARTESIAN_POINT('Ctrl Pts',(-1.98771456680806,-1.,-0.759080037802242));
#29823=CARTESIAN_POINT('Ctrl Pts',(-1.98771456680806,1.,-0.759080037802242));
#29824=CARTESIAN_POINT('Ctrl Pts',(-1.9939983109871,-1.,-0.758281796766377));
#29825=CARTESIAN_POINT('Ctrl Pts',(-1.9939983109871,1.,-0.758281796766377));
#29826=CARTESIAN_POINT('Ctrl Pts',(-2.00028834739072,-1.,-0.757442676862341));
#29827=CARTESIAN_POINT('Ctrl Pts',(-2.00028834739072,1.,-0.757442676862341));
#29828=CARTESIAN_POINT('Ctrl Pts',(-2.00658431587682,-1.,-0.756562904646496));
#29829=CARTESIAN_POINT('Ctrl Pts',(-2.00658431587682,1.,-0.756562904646496));
#29830=CARTESIAN_POINT('Ctrl Pts',(-2.01288584328149,-1.,-0.7556427049581));
#29831=CARTESIAN_POINT('Ctrl Pts',(-2.01288584328149,1.,-0.7556427049581));
#29832=CARTESIAN_POINT('Ctrl Pts',(-2.01919259406003,-1.,-0.75468233072352));
#29833=CARTESIAN_POINT('Ctrl Pts',(-2.01919259406003,1.,-0.75468233072352));
#29834=CARTESIAN_POINT('Ctrl Pts',(-2.02550428623587,-1.,-0.753682061113765));
#29835=CARTESIAN_POINT('Ctrl Pts',(-2.02550428623587,1.,-0.753682061113765));
#29836=CARTESIAN_POINT('Ctrl Pts',(-2.03182068456467,-1.,-0.752642180488104));
#29837=CARTESIAN_POINT('Ctrl Pts',(-2.03182068456467,1.,-0.752642180488104));
#29838=CARTESIAN_POINT('Ctrl Pts',(-2.03814160092173,-1.,-0.751562963361383));
#29839=CARTESIAN_POINT('Ctrl Pts',(-2.03814160092173,1.,-0.751562963361383));
#29840=CARTESIAN_POINT('Ctrl Pts',(-2.04446689147754,-1.,-0.750444657874758));
#29841=CARTESIAN_POINT('Ctrl Pts',(-2.04446689147754,1.,-0.750444657874758));
#29842=CARTESIAN_POINT('Ctrl Pts',(-2.05079645591606,-1.,-0.749287468663053));
#29843=CARTESIAN_POINT('Ctrl Pts',(-2.05079645591606,1.,-0.749287468663053));
#29844=CARTESIAN_POINT('Ctrl Pts',(-2.05713023030263,-1.,-0.748091554181101));
#29845=CARTESIAN_POINT('Ctrl Pts',(-2.05713023030263,1.,-0.748091554181101));
#29846=CARTESIAN_POINT('Ctrl Pts',(-2.06220058927162,-1.,-0.747103932785504));
#29847=CARTESIAN_POINT('Ctrl Pts',(-2.06220058927162,1.,-0.747103932785504));
#29848=CARTESIAN_POINT('Ctrl Pts',(-2.06600523016401,-1.,-0.746345871542695));
#29849=CARTESIAN_POINT('Ctrl Pts',(-2.06600523016401,1.,-0.746345871542695));
#29850=CARTESIAN_POINT('Ctrl Pts',(-2.06854248895575,-1.,-0.74583279137781));
#29851=CARTESIAN_POINT('Ctrl Pts',(-2.06854248895575,1.,-0.74583279137781));
#29852=CARTESIAN_POINT('Ctrl Pts',(-2.0698113262342,-1.,-0.745574324794401));
#29853=CARTESIAN_POINT('Ctrl Pts',(-2.0698113262342,1.,-0.745574324794401));
#29854=CARTESIAN_POINT('',(-1.60662857109684,1.,-0.693717979106306));
#29855=CARTESIAN_POINT('Ctrl Pts',(-1.60662857109684,1.,-0.693717979106306));
#29856=CARTESIAN_POINT('Ctrl Pts',(-1.61106790958151,1.,-0.695712097881194));
#29857=CARTESIAN_POINT('Ctrl Pts',(-1.61974673472612,1.,-0.699605146405088));
#29858=CARTESIAN_POINT('Ctrl Pts',(-1.63216541664676,1.,-0.705159151988319));
#29859=CARTESIAN_POINT('Ctrl Pts',(-1.64752408832016,1.,-0.711993139355394));
#29860=CARTESIAN_POINT('Ctrl Pts',(-1.6647288055568,1.,-0.719585433804282));
#29861=CARTESIAN_POINT('Ctrl Pts',(-1.67996158455503,1.,-0.726235967997433));
#29862=CARTESIAN_POINT('Ctrl Pts',(-1.69326921975743,1.,-0.731963238697195));
#29863=CARTESIAN_POINT('Ctrl Pts',(-1.70473309006121,1.,-0.736799665724771));
#29864=CARTESIAN_POINT('Ctrl Pts',(-1.71447789751927,1.,-0.740795162032087));
#29865=CARTESIAN_POINT('Ctrl Pts',(-1.7226822991693,1.,-0.744021445433764));
#29866=CARTESIAN_POINT('Ctrl Pts',(-1.72958533647399,1.,-0.746574710096436));
#29867=CARTESIAN_POINT('Ctrl Pts',(-1.73550351679848,1.,-0.748582462954854));
#29868=CARTESIAN_POINT('Ctrl Pts',(-1.74080458266705,1.,-0.75019343597954));
#29869=CARTESIAN_POINT('Ctrl Pts',(-1.74585086852298,1.,-0.751555614163629));
#29870=CARTESIAN_POINT('Ctrl Pts',(-1.75095139468809,1.,-0.752797683531377));
#29871=CARTESIAN_POINT('Ctrl Pts',(-1.75631083600175,1.,-0.75400925402848));
#29872=CARTESIAN_POINT('Ctrl Pts',(-1.7619781724032,1.,-0.755220979975262));
#29873=CARTESIAN_POINT('Ctrl Pts',(-1.76789396003141,1.,-0.756421896028403));
#29874=CARTESIAN_POINT('Ctrl Pts',(-1.77394167108342,1.,-0.757578264077238));
#29875=CARTESIAN_POINT('Ctrl Pts',(-1.77999411220912,1.,-0.75865062667738));
#29876=CARTESIAN_POINT('Ctrl Pts',(-1.78596964884526,1.,-0.759614401109868));
#29877=CARTESIAN_POINT('Ctrl Pts',(-1.79185815610802,1.,-0.760469555880425));
#29878=CARTESIAN_POINT('Ctrl Pts',(-1.79768986997735,1.,-0.761229695230359));
#29879=CARTESIAN_POINT('Ctrl Pts',(-1.80351583877334,1.,-0.761915336443515));
#29880=CARTESIAN_POINT('Ctrl Pts',(-1.80938551463989,1.,-0.762546129464036));
#29881=CARTESIAN_POINT('Ctrl Pts',(-1.81532118405566,1.,-0.763132003836783));
#29882=CARTESIAN_POINT('Ctrl Pts',(-1.82131873145297,1.,-0.763673465462854));
#29883=CARTESIAN_POINT('Ctrl Pts',(-1.8273599120008,1.,-0.764165902606055));
#29884=CARTESIAN_POINT('Ctrl Pts',(-1.8334207722714,1.,-0.764602549687845));
#29885=CARTESIAN_POINT('Ctrl Pts',(-1.83948181064823,1.,-0.764978057881687));
#29886=CARTESIAN_POINT('Ctrl Pts',(-1.8455369887591,1.,-0.765291664861971));
#29887=CARTESIAN_POINT('Ctrl Pts',(-1.85158945130054,1.,-0.765545710619023));
#29888=CARTESIAN_POINT('Ctrl Pts',(-1.85764741390391,1.,-0.765744212909305));
#29889=CARTESIAN_POINT('Ctrl Pts',(-1.86372027063314,1.,-0.765891519092557));
#29890=CARTESIAN_POINT('Ctrl Pts',(-1.86981398314345,1.,-0.765990708546111));
#29891=CARTESIAN_POINT('Ctrl Pts',(-1.87592888967886,1.,-0.766042837036759));
#29892=CARTESIAN_POINT('Ctrl Pts',(-1.88206215302561,1.,-0.766047794851868));
#29893=CARTESIAN_POINT('Ctrl Pts',(-1.88820926433409,1.,-0.76600483706209));
#29894=CARTESIAN_POINT('Ctrl Pts',(-1.89436577771389,1.,-0.765913193856979));
#29895=CARTESIAN_POINT('Ctrl Pts',(-1.90052930393599,1.,-0.765772772593395));
#29896=CARTESIAN_POINT('Ctrl Pts',(-1.90669961402362,1.,-0.765584196937936));
#29897=CARTESIAN_POINT('Ctrl Pts',(-1.91287765805174,1.,-0.765348465884739));
#29898=CARTESIAN_POINT('Ctrl Pts',(-1.91906491634197,1.,-0.765066729667095));
#29899=CARTESIAN_POINT('Ctrl Pts',(-1.92526263537041,1.,-0.764740025488189));
#29900=CARTESIAN_POINT('Ctrl Pts',(-1.93147105496367,1.,-0.764369010673889));
#29901=CARTESIAN_POINT('Ctrl Pts',(-1.93768964875867,1.,-0.763954049121393));
#29902=CARTESIAN_POINT('Ctrl Pts',(-1.94391746617626,1.,-0.76349533353858));
#29903=CARTESIAN_POINT('Ctrl Pts',(-1.95015342590025,1.,-0.762992990878774));
#29904=CARTESIAN_POINT('Ctrl Pts',(-1.95639665309893,1.,-0.762447203806263));
#29905=CARTESIAN_POINT('Ctrl Pts',(-1.96264672744229,1.,-0.761858300014575));
#29906=CARTESIAN_POINT('Ctrl Pts',(-1.96890351582545,1.,-0.761226690483986));
#29907=CARTESIAN_POINT('Ctrl Pts',(-1.97516705321521,1.,-0.760552825409855));
#29908=CARTESIAN_POINT('Ctrl Pts',(-1.98143741418156,1.,-0.759837147452135));
#29909=CARTESIAN_POINT('Ctrl Pts',(-1.98771456680806,1.,-0.759080037802242));
#29910=CARTESIAN_POINT('Ctrl Pts',(-1.9939983109871,1.,-0.758281796766377));
#29911=CARTESIAN_POINT('Ctrl Pts',(-2.00028834739072,1.,-0.757442676862341));
#29912=CARTESIAN_POINT('Ctrl Pts',(-2.00658431587682,1.,-0.756562904646496));
#29913=CARTESIAN_POINT('Ctrl Pts',(-2.01288584328149,1.,-0.7556427049581));
#29914=CARTESIAN_POINT('Ctrl Pts',(-2.01919259406003,1.,-0.75468233072352));
#29915=CARTESIAN_POINT('Ctrl Pts',(-2.02550428623587,1.,-0.753682061113765));
#29916=CARTESIAN_POINT('Ctrl Pts',(-2.03182068456467,1.,-0.752642180488104));
#29917=CARTESIAN_POINT('Ctrl Pts',(-2.03814160092173,1.,-0.751562963361383));
#29918=CARTESIAN_POINT('Ctrl Pts',(-2.04446689147754,1.,-0.750444657874758));
#29919=CARTESIAN_POINT('Ctrl Pts',(-2.05079645591606,1.,-0.749287468663053));
#29920=CARTESIAN_POINT('Ctrl Pts',(-2.05713023030263,1.,-0.748091554181101));
#29921=CARTESIAN_POINT('Ctrl Pts',(-2.06220058927162,1.,-0.747103932785504));
#29922=CARTESIAN_POINT('Ctrl Pts',(-2.06600523016401,1.,-0.746345871542695));
#29923=CARTESIAN_POINT('Ctrl Pts',(-2.06854248895575,1.,-0.74583279137781));
#29924=CARTESIAN_POINT('Ctrl Pts',(-2.0698113262342,1.,-0.745574324794401));
#29925=CARTESIAN_POINT('',(-1.60662857109684,0.,-0.693717979106306));
#29926=CARTESIAN_POINT('Origin',(0.,0.,0.));
#29927=CARTESIAN_POINT('',(-1.5055822144029,1.,-0.892032620296855));
#29928=CARTESIAN_POINT('Origin',(0.,1.,0.));
#29929=CARTESIAN_POINT('',(-1.5055822144029,0.,-0.892032620296855));
#29930=CARTESIAN_POINT('Ctrl Pts',(-1.81978687191668,-1.,-1.23627494547115));
#29931=CARTESIAN_POINT('Ctrl Pts',(-1.81978687191668,1.,-1.23627494547115));
#29932=CARTESIAN_POINT('Ctrl Pts',(-1.81925017193666,-1.,-1.23509651170476));
#29933=CARTESIAN_POINT('Ctrl Pts',(-1.81925017193666,1.,-1.23509651170476));
#29934=CARTESIAN_POINT('Ctrl Pts',(-1.81817389921279,-1.,-1.2327422452705));
#29935=CARTESIAN_POINT('Ctrl Pts',(-1.81817389921279,1.,-1.2327422452705));
#29936=CARTESIAN_POINT('Ctrl Pts',(-1.8165508718364,-1.,-1.2292186489137));
#29937=CARTESIAN_POINT('Ctrl Pts',(-1.8165508718364,1.,-1.2292186489137));
#29938=CARTESIAN_POINT('Ctrl Pts',(-1.81436959210434,-1.,-1.2245361330495));
#29939=CARTESIAN_POINT('Ctrl Pts',(-1.81436959210434,1.,-1.2245361330495));
#29940=CARTESIAN_POINT('Ctrl Pts',(-1.81161420806656,-1.,-1.21870906103557));
#29941=CARTESIAN_POINT('Ctrl Pts',(-1.81161420806656,1.,-1.21870906103557));
#29942=CARTESIAN_POINT('Ctrl Pts',(-1.80882996917129,-1.,-1.21290815708314));
#29943=CARTESIAN_POINT('Ctrl Pts',(-1.80882996917129,1.,-1.21290815708314));
#29944=CARTESIAN_POINT('Ctrl Pts',(-1.80601678480707,-1.,-1.20713356605475));
#29945=CARTESIAN_POINT('Ctrl Pts',(-1.80601678480707,1.,-1.20713356605475));
#29946=CARTESIAN_POINT('Ctrl Pts',(-1.80317454838603,-1.,-1.20138548938974));
#29947=CARTESIAN_POINT('Ctrl Pts',(-1.80317454838603,1.,-1.20138548938974));
#29948=CARTESIAN_POINT('Ctrl Pts',(-1.80030314369879,-1.,-1.19566418930242));
#29949=CARTESIAN_POINT('Ctrl Pts',(-1.80030314369879,1.,-1.19566418930242));
#29950=CARTESIAN_POINT('Ctrl Pts',(-1.79740245923478,-1.,-1.18996997934445));
#29951=CARTESIAN_POINT('Ctrl Pts',(-1.79740245923478,1.,-1.18996997934445));
#29952=CARTESIAN_POINT('Ctrl Pts',(-1.79447240321515,-1.,-1.18430321697432));
#29953=CARTESIAN_POINT('Ctrl Pts',(-1.79447240321515,1.,-1.18430321697432));
#29954=CARTESIAN_POINT('Ctrl Pts',(-1.79151291552689,-1.,-1.17866429440809));
#29955=CARTESIAN_POINT('Ctrl Pts',(-1.79151291552689,1.,-1.17866429440809));
#29956=CARTESIAN_POINT('Ctrl Pts',(-1.78852398877616,-1.,-1.17305363177328));
#29957=CARTESIAN_POINT('Ctrl Pts',(-1.78852398877616,1.,-1.17305363177328));
#29958=CARTESIAN_POINT('Ctrl Pts',(-1.78550566040443,-1.,-1.16747166312303));
#29959=CARTESIAN_POINT('Ctrl Pts',(-1.78550566040443,1.,-1.16747166312303));
#29960=CARTESIAN_POINT('Ctrl Pts',(-1.78245795881009,-1.,-1.16191881298499));
#29961=CARTESIAN_POINT('Ctrl Pts',(-1.78245795881009,1.,-1.16191881298499));
#29962=CARTESIAN_POINT('Ctrl Pts',(-1.77938085564275,-1.,-1.15639547194698));
#29963=CARTESIAN_POINT('Ctrl Pts',(-1.77938085564275,1.,-1.15639547194698));
#29964=CARTESIAN_POINT('Ctrl Pts',(-1.7762742255701,-1.,-1.15090197841515));
#29965=CARTESIAN_POINT('Ctrl Pts',(-1.7762742255701,1.,-1.15090197841515));
#29966=CARTESIAN_POINT('Ctrl Pts',(-1.77313777896194,-1.,-1.1454385822692));
#29967=CARTESIAN_POINT('Ctrl Pts',(-1.77313777896194,1.,-1.1454385822692));
#29968=CARTESIAN_POINT('Ctrl Pts',(-1.76997111386769,-1.,-1.14000548336975));
#29969=CARTESIAN_POINT('Ctrl Pts',(-1.76997111386769,1.,-1.14000548336975));
#29970=CARTESIAN_POINT('Ctrl Pts',(-1.76677384551862,-1.,-1.1346029180462));
#29971=CARTESIAN_POINT('Ctrl Pts',(-1.76677384551862,1.,-1.1346029180462));
#29972=CARTESIAN_POINT('Ctrl Pts',(-1.7635457196617,-1.,-1.12923123555075));
#29973=CARTESIAN_POINT('Ctrl Pts',(-1.7635457196617,1.,-1.12923123555075));
#29974=CARTESIAN_POINT('Ctrl Pts',(-1.76028671825096,-1.,-1.12389096855086));
#29975=CARTESIAN_POINT('Ctrl Pts',(-1.76028671825096,1.,-1.12389096855086));
#29976=CARTESIAN_POINT('Ctrl Pts',(-1.75699720772105,-1.,-1.11858293216763));
#29977=CARTESIAN_POINT('Ctrl Pts',(-1.75699720772105,1.,-1.11858293216763));
#29978=CARTESIAN_POINT('Ctrl Pts',(-1.7536777209463,-1.,-1.11330807582551));
#29979=CARTESIAN_POINT('Ctrl Pts',(-1.7536777209463,1.,-1.11330807582551));
#29980=CARTESIAN_POINT('Ctrl Pts',(-1.7503286607592,-1.,-1.10806728183007));
#29981=CARTESIAN_POINT('Ctrl Pts',(-1.7503286607592,1.,-1.10806728183007));
#29982=CARTESIAN_POINT('Ctrl Pts',(-1.74695004214923,-1.,-1.10286118991143));
#29983=CARTESIAN_POINT('Ctrl Pts',(-1.74695004214923,1.,-1.10286118991143));
#29984=CARTESIAN_POINT('Ctrl Pts',(-1.74354119236208,-1.,-1.09768999241225));
#29985=CARTESIAN_POINT('Ctrl Pts',(-1.74354119236208,1.,-1.09768999241225));
#29986=CARTESIAN_POINT('Ctrl Pts',(-1.74010053962247,-1.,-1.09255329056493));
#29987=CARTESIAN_POINT('Ctrl Pts',(-1.74010053962247,1.,-1.09255329056493));
#29988=CARTESIAN_POINT('Ctrl Pts',(-1.73662628326091,-1.,-1.08745056285427));
#29989=CARTESIAN_POINT('Ctrl Pts',(-1.73662628326091,1.,-1.08745056285427));
#29990=CARTESIAN_POINT('Ctrl Pts',(-1.73311705663407,-1.,-1.08238162784749));
#29991=CARTESIAN_POINT('Ctrl Pts',(-1.73311705663407,1.,-1.08238162784749));
#29992=CARTESIAN_POINT('Ctrl Pts',(-1.72957248977424,-1.,-1.0773470373727));
#29993=CARTESIAN_POINT('Ctrl Pts',(-1.72957248977424,1.,-1.0773470373727));
#29994=CARTESIAN_POINT('Ctrl Pts',(-1.72599406198488,-1.,-1.07234866990252));
#29995=CARTESIAN_POINT('Ctrl Pts',(-1.72599406198488,1.,-1.07234866990252));
#29996=CARTESIAN_POINT('Ctrl Pts',(-1.72238500928453,-1.,-1.06738966975462));
#29997=CARTESIAN_POINT('Ctrl Pts',(-1.72238500928453,1.,-1.06738966975462));
#29998=CARTESIAN_POINT('Ctrl Pts',(-1.71874858456904,-1.,-1.06247324680647));
#29999=CARTESIAN_POINT('Ctrl Pts',(-1.71874858456904,1.,-1.06247324680647));
#30000=CARTESIAN_POINT('Ctrl Pts',(-1.7150865442702,-1.,-1.05760163192479));
#30001=CARTESIAN_POINT('Ctrl Pts',(-1.7150865442702,1.,-1.05760163192479));
#30002=CARTESIAN_POINT('Ctrl Pts',(-1.71139783543989,-1.,-1.05277517202855));
#30003=CARTESIAN_POINT('Ctrl Pts',(-1.71139783543989,1.,-1.05277517202855));
#30004=CARTESIAN_POINT('Ctrl Pts',(-1.70767646263649,-1.,-1.04799085404995));
#30005=CARTESIAN_POINT('Ctrl Pts',(-1.70767646263649,1.,-1.04799085404995));
#30006=CARTESIAN_POINT('Ctrl Pts',(-1.70391338707982,-1.,-1.04324363334554));
#30007=CARTESIAN_POINT('Ctrl Pts',(-1.70391338707982,1.,-1.04324363334554));
#30008=CARTESIAN_POINT('Ctrl Pts',(-1.70010052930962,-1.,-1.03852922490789));
#30009=CARTESIAN_POINT('Ctrl Pts',(-1.70010052930962,1.,-1.03852922490789));
#30010=CARTESIAN_POINT('Ctrl Pts',(-1.69623414782771,-1.,-1.03384646003588));
#30011=CARTESIAN_POINT('Ctrl Pts',(-1.69623414782771,1.,-1.03384646003588));
#30012=CARTESIAN_POINT('Ctrl Pts',(-1.69231840863458,-1.,-1.02919977579147));
#30013=CARTESIAN_POINT('Ctrl Pts',(-1.69231840863458,1.,-1.02919977579147));
#30014=CARTESIAN_POINT('Ctrl Pts',(-1.68836910178447,-1.,-1.02460180535255));
#30015=CARTESIAN_POINT('Ctrl Pts',(-1.68836910178447,1.,-1.02460180535255));
#30016=CARTESIAN_POINT('Ctrl Pts',(-1.68440578021706,-1.,-1.02006795074201));
#30017=CARTESIAN_POINT('Ctrl Pts',(-1.68440578021706,1.,-1.02006795074201));
#30018=CARTESIAN_POINT('Ctrl Pts',(-1.68044289894798,-1.,-1.01561026162773));
#30019=CARTESIAN_POINT('Ctrl Pts',(-1.68044289894798,1.,-1.01561026162773));
#30020=CARTESIAN_POINT('Ctrl Pts',(-1.67648246776464,-1.,-1.01123236493511));
#30021=CARTESIAN_POINT('Ctrl Pts',(-1.67648246776464,1.,-1.01123236493511));
#30022=CARTESIAN_POINT('Ctrl Pts',(-1.67250335383293,-1.,-1.00692206696414));
#30023=CARTESIAN_POINT('Ctrl Pts',(-1.67250335383293,1.,-1.00692206696414));
#30024=CARTESIAN_POINT('Ctrl Pts',(-1.66846059277303,-1.,-1.00265091003727));
#30025=CARTESIAN_POINT('Ctrl Pts',(-1.66846059277303,1.,-1.00265091003727));
#30026=CARTESIAN_POINT('Ctrl Pts',(-1.66430758030376,-1.,-0.998389654952758));
#30027=CARTESIAN_POINT('Ctrl Pts',(-1.66430758030376,1.,-0.998389654952758));
#30028=CARTESIAN_POINT('Ctrl Pts',(-1.66001553809947,-1.,-0.994121836661306));
#30029=CARTESIAN_POINT('Ctrl Pts',(-1.66001553809947,1.,-0.994121836661306));
#30030=CARTESIAN_POINT('Ctrl Pts',(-1.65559044289699,-1.,-0.989855627854165));
#30031=CARTESIAN_POINT('Ctrl Pts',(-1.65559044289699,1.,-0.989855627854165));
#30032=CARTESIAN_POINT('Ctrl Pts',(-1.65110016612638,-1.,-0.985642622920821));
#30033=CARTESIAN_POINT('Ctrl Pts',(-1.65110016612638,1.,-0.985642622920821));
#30034=CARTESIAN_POINT('Ctrl Pts',(-1.64665139190656,-1.,-0.981562530939489));
#30035=CARTESIAN_POINT('Ctrl Pts',(-1.64665139190656,1.,-0.981562530939489));
#30036=CARTESIAN_POINT('Ctrl Pts',(-1.64233990826687,-1.,-0.977689794119416));
#30037=CARTESIAN_POINT('Ctrl Pts',(-1.64233990826687,1.,-0.977689794119416));
#30038=CARTESIAN_POINT('Ctrl Pts',(-1.63820952658144,-1.,-0.974066058287418));
#30039=CARTESIAN_POINT('Ctrl Pts',(-1.63820952658144,1.,-0.974066058287418));
#30040=CARTESIAN_POINT('Ctrl Pts',(-1.63420665729798,-1.,-0.970669715997509));
#30041=CARTESIAN_POINT('Ctrl Pts',(-1.63420665729798,1.,-0.970669715997509));
#30042=CARTESIAN_POINT('Ctrl Pts',(-1.63013849959461,-1.,-0.967387853230345));
#30043=CARTESIAN_POINT('Ctrl Pts',(-1.63013849959461,1.,-0.967387853230345));
#30044=CARTESIAN_POINT('Ctrl Pts',(-1.62571930670187,-1.,-0.964046107040536));
#30045=CARTESIAN_POINT('Ctrl Pts',(-1.62571930670187,1.,-0.964046107040536));
#30046=CARTESIAN_POINT('Ctrl Pts',(-1.62061638140221,-1.,-0.960438326101729));
#30047=CARTESIAN_POINT('Ctrl Pts',(-1.62061638140221,1.,-0.960438326101729));
#30048=CARTESIAN_POINT('Ctrl Pts',(-1.61449324337085,-1.,-0.956354422920671));
#30049=CARTESIAN_POINT('Ctrl Pts',(-1.61449324337085,1.,-0.956354422920671));
#30050=CARTESIAN_POINT('Ctrl Pts',(-1.60706069896936,-1.,-0.951613284356035));
#30051=CARTESIAN_POINT('Ctrl Pts',(-1.60706069896936,1.,-0.951613284356035));
#30052=CARTESIAN_POINT('Ctrl Pts',(-1.59810042043673,-1.,-0.946078063315257));
#30053=CARTESIAN_POINT('Ctrl Pts',(-1.59810042043673,1.,-0.946078063315257));
#30054=CARTESIAN_POINT('Ctrl Pts',(-1.58744937487176,-1.,-0.939646377893399));
#30055=CARTESIAN_POINT('Ctrl Pts',(-1.58744937487176,1.,-0.939646377893399));
#30056=CARTESIAN_POINT('Ctrl Pts',(-1.57499388382243,-1.,-0.932246680108685));
#30057=CARTESIAN_POINT('Ctrl Pts',(-1.57499388382243,1.,-0.932246680108685));
#30058=CARTESIAN_POINT('Ctrl Pts',(-1.56065988578893,-1.,-0.923832188944341));
#30059=CARTESIAN_POINT('Ctrl Pts',(-1.56065988578893,1.,-0.923832188944341));
#30060=CARTESIAN_POINT('Ctrl Pts',(-1.54440491149498,-1.,-0.914375919026456));
#30061=CARTESIAN_POINT('Ctrl Pts',(-1.54440491149498,1.,-0.914375919026456));
#30062=CARTESIAN_POINT('Ctrl Pts',(-1.52984849887993,-1.,-0.905967409625651));
#30063=CARTESIAN_POINT('Ctrl Pts',(-1.52984849887993,1.,-0.905967409625651));
#30064=CARTESIAN_POINT('Ctrl Pts',(-1.51805569590094,-1.,-0.899185047483511));
#30065=CARTESIAN_POINT('Ctrl Pts',(-1.51805569590094,1.,-0.899185047483511));
#30066=CARTESIAN_POINT('Ctrl Pts',(-1.50980486806688,-1.,-0.894452006964543));
#30067=CARTESIAN_POINT('Ctrl Pts',(-1.50980486806688,1.,-0.894452006964543));
#30068=CARTESIAN_POINT('Ctrl Pts',(-1.5055822144029,-1.,-0.892032620296855));
#30069=CARTESIAN_POINT('Ctrl Pts',(-1.5055822144029,1.,-0.892032620296855));
#30070=CARTESIAN_POINT('',(-1.81978687191668,1.,-1.23627494547115));
#30071=CARTESIAN_POINT('Ctrl Pts',(-1.81978687191668,1.,-1.23627494547115));
#30072=CARTESIAN_POINT('Ctrl Pts',(-1.81925017193666,1.,-1.23509651170476));
#30073=CARTESIAN_POINT('Ctrl Pts',(-1.81817389921279,1.,-1.2327422452705));
#30074=CARTESIAN_POINT('Ctrl Pts',(-1.8165508718364,1.,-1.2292186489137));
#30075=CARTESIAN_POINT('Ctrl Pts',(-1.81436959210434,1.,-1.2245361330495));
#30076=CARTESIAN_POINT('Ctrl Pts',(-1.81161420806656,1.,-1.21870906103557));
#30077=CARTESIAN_POINT('Ctrl Pts',(-1.80882996917129,1.,-1.21290815708314));
#30078=CARTESIAN_POINT('Ctrl Pts',(-1.80601678480707,1.,-1.20713356605475));
#30079=CARTESIAN_POINT('Ctrl Pts',(-1.80317454838603,1.,-1.20138548938974));
#30080=CARTESIAN_POINT('Ctrl Pts',(-1.80030314369879,1.,-1.19566418930242));
#30081=CARTESIAN_POINT('Ctrl Pts',(-1.79740245923478,1.,-1.18996997934445));
#30082=CARTESIAN_POINT('Ctrl Pts',(-1.79447240321515,1.,-1.18430321697432));
#30083=CARTESIAN_POINT('Ctrl Pts',(-1.79151291552689,1.,-1.17866429440809));
#30084=CARTESIAN_POINT('Ctrl Pts',(-1.78852398877616,1.,-1.17305363177328));
#30085=CARTESIAN_POINT('Ctrl Pts',(-1.78550566040443,1.,-1.16747166312303));
#30086=CARTESIAN_POINT('Ctrl Pts',(-1.78245795881009,1.,-1.16191881298499));
#30087=CARTESIAN_POINT('Ctrl Pts',(-1.77938085564275,1.,-1.15639547194698));
#30088=CARTESIAN_POINT('Ctrl Pts',(-1.7762742255701,1.,-1.15090197841515));
#30089=CARTESIAN_POINT('Ctrl Pts',(-1.77313777896194,1.,-1.1454385822692));
#30090=CARTESIAN_POINT('Ctrl Pts',(-1.76997111386769,1.,-1.14000548336975));
#30091=CARTESIAN_POINT('Ctrl Pts',(-1.76677384551862,1.,-1.1346029180462));
#30092=CARTESIAN_POINT('Ctrl Pts',(-1.7635457196617,1.,-1.12923123555075));
#30093=CARTESIAN_POINT('Ctrl Pts',(-1.76028671825096,1.,-1.12389096855086));
#30094=CARTESIAN_POINT('Ctrl Pts',(-1.75699720772105,1.,-1.11858293216763));
#30095=CARTESIAN_POINT('Ctrl Pts',(-1.7536777209463,1.,-1.11330807582551));
#30096=CARTESIAN_POINT('Ctrl Pts',(-1.7503286607592,1.,-1.10806728183007));
#30097=CARTESIAN_POINT('Ctrl Pts',(-1.74695004214923,1.,-1.10286118991143));
#30098=CARTESIAN_POINT('Ctrl Pts',(-1.74354119236208,1.,-1.09768999241225));
#30099=CARTESIAN_POINT('Ctrl Pts',(-1.74010053962247,1.,-1.09255329056493));
#30100=CARTESIAN_POINT('Ctrl Pts',(-1.73662628326091,1.,-1.08745056285427));
#30101=CARTESIAN_POINT('Ctrl Pts',(-1.73311705663407,1.,-1.08238162784749));
#30102=CARTESIAN_POINT('Ctrl Pts',(-1.72957248977424,1.,-1.0773470373727));
#30103=CARTESIAN_POINT('Ctrl Pts',(-1.72599406198488,1.,-1.07234866990252));
#30104=CARTESIAN_POINT('Ctrl Pts',(-1.72238500928453,1.,-1.06738966975462));
#30105=CARTESIAN_POINT('Ctrl Pts',(-1.71874858456904,1.,-1.06247324680647));
#30106=CARTESIAN_POINT('Ctrl Pts',(-1.7150865442702,1.,-1.05760163192479));
#30107=CARTESIAN_POINT('Ctrl Pts',(-1.71139783543989,1.,-1.05277517202855));
#30108=CARTESIAN_POINT('Ctrl Pts',(-1.70767646263649,1.,-1.04799085404995));
#30109=CARTESIAN_POINT('Ctrl Pts',(-1.70391338707982,1.,-1.04324363334554));
#30110=CARTESIAN_POINT('Ctrl Pts',(-1.70010052930962,1.,-1.03852922490789));
#30111=CARTESIAN_POINT('Ctrl Pts',(-1.69623414782771,1.,-1.03384646003588));
#30112=CARTESIAN_POINT('Ctrl Pts',(-1.69231840863458,1.,-1.02919977579147));
#30113=CARTESIAN_POINT('Ctrl Pts',(-1.68836910178447,1.,-1.02460180535255));
#30114=CARTESIAN_POINT('Ctrl Pts',(-1.68440578021706,1.,-1.02006795074201));
#30115=CARTESIAN_POINT('Ctrl Pts',(-1.68044289894798,1.,-1.01561026162773));
#30116=CARTESIAN_POINT('Ctrl Pts',(-1.67648246776464,1.,-1.01123236493511));
#30117=CARTESIAN_POINT('Ctrl Pts',(-1.67250335383293,1.,-1.00692206696414));
#30118=CARTESIAN_POINT('Ctrl Pts',(-1.66846059277303,1.,-1.00265091003727));
#30119=CARTESIAN_POINT('Ctrl Pts',(-1.66430758030376,1.,-0.998389654952758));
#30120=CARTESIAN_POINT('Ctrl Pts',(-1.66001553809947,1.,-0.994121836661306));
#30121=CARTESIAN_POINT('Ctrl Pts',(-1.65559044289699,1.,-0.989855627854165));
#30122=CARTESIAN_POINT('Ctrl Pts',(-1.65110016612638,1.,-0.985642622920821));
#30123=CARTESIAN_POINT('Ctrl Pts',(-1.64665139190656,1.,-0.981562530939489));
#30124=CARTESIAN_POINT('Ctrl Pts',(-1.64233990826687,1.,-0.977689794119416));
#30125=CARTESIAN_POINT('Ctrl Pts',(-1.63820952658144,1.,-0.974066058287418));
#30126=CARTESIAN_POINT('Ctrl Pts',(-1.63420665729798,1.,-0.970669715997509));
#30127=CARTESIAN_POINT('Ctrl Pts',(-1.63013849959461,1.,-0.967387853230345));
#30128=CARTESIAN_POINT('Ctrl Pts',(-1.62571930670187,1.,-0.964046107040536));
#30129=CARTESIAN_POINT('Ctrl Pts',(-1.62061638140221,1.,-0.960438326101729));
#30130=CARTESIAN_POINT('Ctrl Pts',(-1.61449324337085,1.,-0.956354422920671));
#30131=CARTESIAN_POINT('Ctrl Pts',(-1.60706069896936,1.,-0.951613284356035));
#30132=CARTESIAN_POINT('Ctrl Pts',(-1.59810042043673,1.,-0.946078063315257));
#30133=CARTESIAN_POINT('Ctrl Pts',(-1.58744937487176,1.,-0.939646377893399));
#30134=CARTESIAN_POINT('Ctrl Pts',(-1.57499388382243,1.,-0.932246680108685));
#30135=CARTESIAN_POINT('Ctrl Pts',(-1.56065988578893,1.,-0.923832188944341));
#30136=CARTESIAN_POINT('Ctrl Pts',(-1.54440491149498,1.,-0.914375919026456));
#30137=CARTESIAN_POINT('Ctrl Pts',(-1.52984849887993,1.,-0.905967409625651));
#30138=CARTESIAN_POINT('Ctrl Pts',(-1.51805569590094,1.,-0.899185047483511));
#30139=CARTESIAN_POINT('Ctrl Pts',(-1.50980486806688,1.,-0.894452006964543));
#30140=CARTESIAN_POINT('Ctrl Pts',(-1.5055822144029,1.,-0.892032620296855));
#30141=CARTESIAN_POINT('',(-1.81978687191668,0.,-1.23627494547115));
#30142=CARTESIAN_POINT('Origin',(-1.73811241238545,0.,-1.34869019493419));
#30143=CARTESIAN_POINT('',(-1.73811241238545,1.,-1.34869019493419));
#30144=CARTESIAN_POINT('',(-1.81978687191668,1.,-1.23627494547115));
#30145=CARTESIAN_POINT('',(-1.73811241238545,0.,-1.34869019493419));
#30146=CARTESIAN_POINT('Ctrl Pts',(-1.31362392696032,-1.,-1.15624053661742));
#30147=CARTESIAN_POINT('Ctrl Pts',(-1.31362392696032,1.,-1.15624053661742));
#30148=CARTESIAN_POINT('Ctrl Pts',(-1.31722977216397,-1.,-1.15950888730809));
#30149=CARTESIAN_POINT('Ctrl Pts',(-1.31722977216397,1.,-1.15950888730809));
#30150=CARTESIAN_POINT('Ctrl Pts',(-1.32428080721772,-1.,-1.16589330093588));
#30151=CARTESIAN_POINT('Ctrl Pts',(-1.32428080721772,1.,-1.16589330093588));
#30152=CARTESIAN_POINT('Ctrl Pts',(-1.33437539347008,-1.,-1.17501305789857));
#30153=CARTESIAN_POINT('Ctrl Pts',(-1.33437539347008,1.,-1.17501305789857));
#30154=CARTESIAN_POINT('Ctrl Pts',(-1.34687054001093,-1.,-1.18625865667441));
#30155=CARTESIAN_POINT('Ctrl Pts',(-1.34687054001093,1.,-1.18625865667441));
#30156=CARTESIAN_POINT('Ctrl Pts',(-1.36088705043885,-1.,-1.1987959077932));
#30157=CARTESIAN_POINT('Ctrl Pts',(-1.36088705043885,1.,-1.1987959077932));
#30158=CARTESIAN_POINT('Ctrl Pts',(-1.37331915607905,-1.,-1.20982812925645));
#30159=CARTESIAN_POINT('Ctrl Pts',(-1.37331915607905,1.,-1.20982812925645));
#30160=CARTESIAN_POINT('Ctrl Pts',(-1.38420564527715,-1.,-1.21938737280852));
#30161=CARTESIAN_POINT('Ctrl Pts',(-1.38420564527715,1.,-1.21938737280852));
#30162=CARTESIAN_POINT('Ctrl Pts',(-1.39361389568796,-1.,-1.22752961899387));
#30163=CARTESIAN_POINT('Ctrl Pts',(-1.39361389568796,1.,-1.22752961899387));
#30164=CARTESIAN_POINT('Ctrl Pts',(-1.40164708206106,-1.,-1.23434087290423));
#30165=CARTESIAN_POINT('Ctrl Pts',(-1.40164708206106,1.,-1.23434087290423));
#30166=CARTESIAN_POINT('Ctrl Pts',(-1.40845295531283,-1.,-1.23994455029534));
#30167=CARTESIAN_POINT('Ctrl Pts',(-1.40845295531283,1.,-1.23994455029534));
#30168=CARTESIAN_POINT('Ctrl Pts',(-1.41422913175179,-1.,-1.24450600513056));
#30169=CARTESIAN_POINT('Ctrl Pts',(-1.41422913175179,1.,-1.24450600513056));
#30170=CARTESIAN_POINT('Ctrl Pts',(-1.41923722596025,-1.,-1.24824430986571));
#30171=CARTESIAN_POINT('Ctrl Pts',(-1.41923722596025,1.,-1.24824430986571));
#30172=CARTESIAN_POINT('Ctrl Pts',(-1.42378102115575,-1.,-1.2514145557001));
#30173=CARTESIAN_POINT('Ctrl Pts',(-1.42378102115575,1.,-1.2514145557001));
#30174=CARTESIAN_POINT('Ctrl Pts',(-1.42815938799387,-1.,-1.25426945222639));
#30175=CARTESIAN_POINT('Ctrl Pts',(-1.42815938799387,1.,-1.25426945222639));
#30176=CARTESIAN_POINT('Ctrl Pts',(-1.43262645609691,-1.,-1.25702687965755));
#30177=CARTESIAN_POINT('Ctrl Pts',(-1.43262645609691,1.,-1.25702687965755));
#30178=CARTESIAN_POINT('Ctrl Pts',(-1.43734919180848,-1.,-1.25983531012005));
#30179=CARTESIAN_POINT('Ctrl Pts',(-1.43734919180848,1.,-1.25983531012005));
#30180=CARTESIAN_POINT('Ctrl Pts',(-1.44236470511303,-1.,-1.26273903323859));
#30181=CARTESIAN_POINT('Ctrl Pts',(-1.44236470511303,1.,-1.26273903323859));
#30182=CARTESIAN_POINT('Ctrl Pts',(-1.44761985001662,-1.,-1.26570925118868));
#30183=CARTESIAN_POINT('Ctrl Pts',(-1.44761985001662,1.,-1.26570925118868));
#30184=CARTESIAN_POINT('Ctrl Pts',(-1.45301422764247,-1.,-1.2686778680489));
#30185=CARTESIAN_POINT('Ctrl Pts',(-1.45301422764247,1.,-1.2686778680489));
#30186=CARTESIAN_POINT('Ctrl Pts',(-1.45843906294697,-1.,-1.27156805265289));
#30187=CARTESIAN_POINT('Ctrl Pts',(-1.45843906294697,1.,-1.27156805265289));
#30188=CARTESIAN_POINT('Ctrl Pts',(-1.46382431332476,-1.,-1.27433119897822));
#30189=CARTESIAN_POINT('Ctrl Pts',(-1.46382431332476,1.,-1.27433119897822));
#30190=CARTESIAN_POINT('Ctrl Pts',(-1.46916035917133,-1.,-1.27696414831089));
#30191=CARTESIAN_POINT('Ctrl Pts',(-1.46916035917133,1.,-1.27696414831089));
#30192=CARTESIAN_POINT('Ctrl Pts',(-1.4744717526707,-1.,-1.2794891824849));
#30193=CARTESIAN_POINT('Ctrl Pts',(-1.4744717526707,1.,-1.2794891824849));
#30194=CARTESIAN_POINT('Ctrl Pts',(-1.47980070347095,-1.,-1.28194158939517));
#30195=CARTESIAN_POINT('Ctrl Pts',(-1.47980070347095,1.,-1.28194158939517));
#30196=CARTESIAN_POINT('Ctrl Pts',(-1.4851881711891,-1.,-1.28435533880201));
#30197=CARTESIAN_POINT('Ctrl Pts',(-1.4851881711891,1.,-1.28435533880201));
#30198=CARTESIAN_POINT('Ctrl Pts',(-1.4906522831278,-1.,-1.2867467611644));
#30199=CARTESIAN_POINT('Ctrl Pts',(-1.4906522831278,1.,-1.2867467611644));
#30200=CARTESIAN_POINT('Ctrl Pts',(-1.49618896881754,-1.,-1.28911506584254));
#30201=CARTESIAN_POINT('Ctrl Pts',(-1.49618896881754,1.,-1.28911506584254));
#30202=CARTESIAN_POINT('Ctrl Pts',(-1.50178230149776,-1.,-1.29145022885181));
#30203=CARTESIAN_POINT('Ctrl Pts',(-1.50178230149776,1.,-1.29145022885181));
#30204=CARTESIAN_POINT('Ctrl Pts',(-1.50741159078365,-1.,-1.29373841372842));
#30205=CARTESIAN_POINT('Ctrl Pts',(-1.50741159078365,1.,-1.29373841372842));
#30206=CARTESIAN_POINT('Ctrl Pts',(-1.51305994241402,-1.,-1.29596850710509));
#30207=CARTESIAN_POINT('Ctrl Pts',(-1.51305994241402,1.,-1.29596850710509));
#30208=CARTESIAN_POINT('Ctrl Pts',(-1.51872184912724,-1.,-1.29813791800747));
#30209=CARTESIAN_POINT('Ctrl Pts',(-1.51872184912724,1.,-1.29813791800747));
#30210=CARTESIAN_POINT('Ctrl Pts',(-1.52439957861062,-1.,-1.30024984366328));
#30211=CARTESIAN_POINT('Ctrl Pts',(-1.52439957861062,1.,-1.30024984366328));
#30212=CARTESIAN_POINT('Ctrl Pts',(-1.53009970283891,-1.,-1.30231064395568));
#30213=CARTESIAN_POINT('Ctrl Pts',(-1.53009970283891,1.,-1.30231064395568));
#30214=CARTESIAN_POINT('Ctrl Pts',(-1.53582981268977,-1.,-1.30432735639489));
#30215=CARTESIAN_POINT('Ctrl Pts',(-1.53582981268977,1.,-1.30432735639489));
#30216=CARTESIAN_POINT('Ctrl Pts',(-1.54159462645432,-1.,-1.30630475189556));
#30217=CARTESIAN_POINT('Ctrl Pts',(-1.54159462645432,1.,-1.30630475189556));
#30218=CARTESIAN_POINT('Ctrl Pts',(-1.54739413957185,-1.,-1.30824393907473));
#30219=CARTESIAN_POINT('Ctrl Pts',(-1.54739413957185,1.,-1.30824393907473));
#30220=CARTESIAN_POINT('Ctrl Pts',(-1.55322568759481,-1.,-1.31014393684222));
#30221=CARTESIAN_POINT('Ctrl Pts',(-1.55322568759481,1.,-1.31014393684222));
#30222=CARTESIAN_POINT('Ctrl Pts',(-1.55908521254821,-1.,-1.31200264341696));
#30223=CARTESIAN_POINT('Ctrl Pts',(-1.55908521254821,1.,-1.31200264341696));
#30224=CARTESIAN_POINT('Ctrl Pts',(-1.56496872402353,-1.,-1.31381795281002));
#30225=CARTESIAN_POINT('Ctrl Pts',(-1.56496872402353,1.,-1.31381795281002));
#30226=CARTESIAN_POINT('Ctrl Pts',(-1.57087397835723,-1.,-1.31558903860016));
#30227=CARTESIAN_POINT('Ctrl Pts',(-1.57087397835723,1.,-1.31558903860016));
#30228=CARTESIAN_POINT('Ctrl Pts',(-1.5768005650559,-1.,-1.31731642317187));
#30229=CARTESIAN_POINT('Ctrl Pts',(-1.5768005650559,1.,-1.31731642317187));
#30230=CARTESIAN_POINT('Ctrl Pts',(-1.58274907898834,-1.,-1.31900135021432));
#30231=CARTESIAN_POINT('Ctrl Pts',(-1.58274907898834,1.,-1.31900135021432));
#30232=CARTESIAN_POINT('Ctrl Pts',(-1.58872057258245,-1.,-1.32064537110892));
#30233=CARTESIAN_POINT('Ctrl Pts',(-1.58872057258245,1.,-1.32064537110892));
#30234=CARTESIAN_POINT('Ctrl Pts',(-1.59471591079403,-1.,-1.32224985747682));
#30235=CARTESIAN_POINT('Ctrl Pts',(-1.59471591079403,1.,-1.32224985747682));
#30236=CARTESIAN_POINT('Ctrl Pts',(-1.60073511858687,-1.,-1.32381550858256));
#30237=CARTESIAN_POINT('Ctrl Pts',(-1.60073511858687,1.,-1.32381550858256));
#30238=CARTESIAN_POINT('Ctrl Pts',(-1.60677758290954,-1.,-1.32534250785782));
#30239=CARTESIAN_POINT('Ctrl Pts',(-1.60677758290954,1.,-1.32534250785782));
#30240=CARTESIAN_POINT('Ctrl Pts',(-1.6128423401575,-1.,-1.32683074483356));
#30241=CARTESIAN_POINT('Ctrl Pts',(-1.6128423401575,1.,-1.32683074483356));
#30242=CARTESIAN_POINT('Ctrl Pts',(-1.61892832270724,-1.,-1.32828000610449));
#30243=CARTESIAN_POINT('Ctrl Pts',(-1.61892832270724,1.,-1.32828000610449));
#30244=CARTESIAN_POINT('Ctrl Pts',(-1.62503464209797,-1.,-1.3296901950568));
#30245=CARTESIAN_POINT('Ctrl Pts',(-1.62503464209797,1.,-1.3296901950568));
#30246=CARTESIAN_POINT('Ctrl Pts',(-1.63116079730923,-1.,-1.33106149345645));
#30247=CARTESIAN_POINT('Ctrl Pts',(-1.63116079730923,1.,-1.33106149345645));
#30248=CARTESIAN_POINT('Ctrl Pts',(-1.63730653475089,-1.,-1.33239425103724));
#30249=CARTESIAN_POINT('Ctrl Pts',(-1.63730653475089,1.,-1.33239425103724));
#30250=CARTESIAN_POINT('Ctrl Pts',(-1.6434717485603,-1.,-1.33368890676572));
#30251=CARTESIAN_POINT('Ctrl Pts',(-1.6434717485603,1.,-1.33368890676572));
#30252=CARTESIAN_POINT('Ctrl Pts',(-1.6496563728683,-1.,-1.33494590467993));
#30253=CARTESIAN_POINT('Ctrl Pts',(-1.6496563728683,1.,-1.33494590467993));
#30254=CARTESIAN_POINT('Ctrl Pts',(-1.65586025952593,-1.,-1.33616559745172));
#30255=CARTESIAN_POINT('Ctrl Pts',(-1.65586025952593,1.,-1.33616559745172));
#30256=CARTESIAN_POINT('Ctrl Pts',(-1.66208312541983,-1.,-1.33734820885262));
#30257=CARTESIAN_POINT('Ctrl Pts',(-1.66208312541983,1.,-1.33734820885262));
#30258=CARTESIAN_POINT('Ctrl Pts',(-1.66832460783989,-1.,-1.33849388654388));
#30259=CARTESIAN_POINT('Ctrl Pts',(-1.66832460783989,1.,-1.33849388654388));
#30260=CARTESIAN_POINT('Ctrl Pts',(-1.67458429426086,-1.,-1.3396027347034));
#30261=CARTESIAN_POINT('Ctrl Pts',(-1.67458429426086,1.,-1.3396027347034));
#30262=CARTESIAN_POINT('Ctrl Pts',(-1.68086176030362,-1.,-1.34067485185203));
#30263=CARTESIAN_POINT('Ctrl Pts',(-1.68086176030362,1.,-1.34067485185203));
#30264=CARTESIAN_POINT('Ctrl Pts',(-1.68715660868764,-1.,-1.341710374848));
#30265=CARTESIAN_POINT('Ctrl Pts',(-1.68715660868764,1.,-1.341710374848));
#30266=CARTESIAN_POINT('Ctrl Pts',(-1.6934684849687,-1.,-1.34270948206319));
#30267=CARTESIAN_POINT('Ctrl Pts',(-1.6934684849687,1.,-1.34270948206319));
#30268=CARTESIAN_POINT('Ctrl Pts',(-1.69979707754427,-1.,-1.34367237124483));
#30269=CARTESIAN_POINT('Ctrl Pts',(-1.69979707754427,1.,-1.34367237124483));
#30270=CARTESIAN_POINT('Ctrl Pts',(-1.70614212266738,-1.,-1.34459924533831));
#30271=CARTESIAN_POINT('Ctrl Pts',(-1.70614212266738,1.,-1.34459924533831));
#30272=CARTESIAN_POINT('Ctrl Pts',(-1.71250340686822,-1.,-1.34549029589416));
#30273=CARTESIAN_POINT('Ctrl Pts',(-1.71250340686822,1.,-1.34549029589416));
#30274=CARTESIAN_POINT('Ctrl Pts',(-1.7188807715049,-1.,-1.34634568653227));
#30275=CARTESIAN_POINT('Ctrl Pts',(-1.7188807715049,1.,-1.34634568653227));
#30276=CARTESIAN_POINT('Ctrl Pts',(-1.72527410680674,-1.,-1.34716554819527));
#30277=CARTESIAN_POINT('Ctrl Pts',(-1.72527410680674,1.,-1.34716554819527));
#30278=CARTESIAN_POINT('Ctrl Pts',(-1.7304014965394,-1.,-1.34779309152035));
#30279=CARTESIAN_POINT('Ctrl Pts',(-1.7304014965394,1.,-1.34779309152035));
#30280=CARTESIAN_POINT('Ctrl Pts',(-1.73425417885907,-1.,-1.34824783112887));
#30281=CARTESIAN_POINT('Ctrl Pts',(-1.73425417885907,1.,-1.34824783112887));
#30282=CARTESIAN_POINT('Ctrl Pts',(-1.73682580585691,-1.,-1.34854391898045));
#30283=CARTESIAN_POINT('Ctrl Pts',(-1.73682580585691,1.,-1.34854391898045));
#30284=CARTESIAN_POINT('Ctrl Pts',(-1.73811241238545,-1.,-1.34869019493419));
#30285=CARTESIAN_POINT('Ctrl Pts',(-1.73811241238545,1.,-1.34869019493419));
#30286=CARTESIAN_POINT('',(-1.31362392696032,1.,-1.15624053661742));
#30287=CARTESIAN_POINT('Ctrl Pts',(-1.31362392696032,1.,-1.15624053661742));
#30288=CARTESIAN_POINT('Ctrl Pts',(-1.31722977216397,1.,-1.15950888730809));
#30289=CARTESIAN_POINT('Ctrl Pts',(-1.32428080721772,1.,-1.16589330093588));
#30290=CARTESIAN_POINT('Ctrl Pts',(-1.33437539347008,1.,-1.17501305789857));
#30291=CARTESIAN_POINT('Ctrl Pts',(-1.34687054001093,1.,-1.18625865667441));
#30292=CARTESIAN_POINT('Ctrl Pts',(-1.36088705043885,1.,-1.1987959077932));
#30293=CARTESIAN_POINT('Ctrl Pts',(-1.37331915607905,1.,-1.20982812925645));
#30294=CARTESIAN_POINT('Ctrl Pts',(-1.38420564527715,1.,-1.21938737280852));
#30295=CARTESIAN_POINT('Ctrl Pts',(-1.39361389568796,1.,-1.22752961899387));
#30296=CARTESIAN_POINT('Ctrl Pts',(-1.40164708206106,1.,-1.23434087290423));
#30297=CARTESIAN_POINT('Ctrl Pts',(-1.40845295531283,1.,-1.23994455029534));
#30298=CARTESIAN_POINT('Ctrl Pts',(-1.41422913175179,1.,-1.24450600513056));
#30299=CARTESIAN_POINT('Ctrl Pts',(-1.41923722596025,1.,-1.24824430986571));
#30300=CARTESIAN_POINT('Ctrl Pts',(-1.42378102115575,1.,-1.2514145557001));
#30301=CARTESIAN_POINT('Ctrl Pts',(-1.42815938799387,1.,-1.25426945222639));
#30302=CARTESIAN_POINT('Ctrl Pts',(-1.43262645609691,1.,-1.25702687965755));
#30303=CARTESIAN_POINT('Ctrl Pts',(-1.43734919180848,1.,-1.25983531012005));
#30304=CARTESIAN_POINT('Ctrl Pts',(-1.44236470511303,1.,-1.26273903323859));
#30305=CARTESIAN_POINT('Ctrl Pts',(-1.44761985001662,1.,-1.26570925118868));
#30306=CARTESIAN_POINT('Ctrl Pts',(-1.45301422764247,1.,-1.2686778680489));
#30307=CARTESIAN_POINT('Ctrl Pts',(-1.45843906294697,1.,-1.27156805265289));
#30308=CARTESIAN_POINT('Ctrl Pts',(-1.46382431332476,1.,-1.27433119897822));
#30309=CARTESIAN_POINT('Ctrl Pts',(-1.46916035917133,1.,-1.27696414831089));
#30310=CARTESIAN_POINT('Ctrl Pts',(-1.4744717526707,1.,-1.2794891824849));
#30311=CARTESIAN_POINT('Ctrl Pts',(-1.47980070347095,1.,-1.28194158939517));
#30312=CARTESIAN_POINT('Ctrl Pts',(-1.4851881711891,1.,-1.28435533880201));
#30313=CARTESIAN_POINT('Ctrl Pts',(-1.4906522831278,1.,-1.2867467611644));
#30314=CARTESIAN_POINT('Ctrl Pts',(-1.49618896881754,1.,-1.28911506584254));
#30315=CARTESIAN_POINT('Ctrl Pts',(-1.50178230149776,1.,-1.29145022885181));
#30316=CARTESIAN_POINT('Ctrl Pts',(-1.50741159078365,1.,-1.29373841372842));
#30317=CARTESIAN_POINT('Ctrl Pts',(-1.51305994241402,1.,-1.29596850710509));
#30318=CARTESIAN_POINT('Ctrl Pts',(-1.51872184912724,1.,-1.29813791800747));
#30319=CARTESIAN_POINT('Ctrl Pts',(-1.52439957861062,1.,-1.30024984366328));
#30320=CARTESIAN_POINT('Ctrl Pts',(-1.53009970283891,1.,-1.30231064395568));
#30321=CARTESIAN_POINT('Ctrl Pts',(-1.53582981268977,1.,-1.30432735639489));
#30322=CARTESIAN_POINT('Ctrl Pts',(-1.54159462645432,1.,-1.30630475189556));
#30323=CARTESIAN_POINT('Ctrl Pts',(-1.54739413957185,1.,-1.30824393907473));
#30324=CARTESIAN_POINT('Ctrl Pts',(-1.55322568759481,1.,-1.31014393684222));
#30325=CARTESIAN_POINT('Ctrl Pts',(-1.55908521254821,1.,-1.31200264341696));
#30326=CARTESIAN_POINT('Ctrl Pts',(-1.56496872402353,1.,-1.31381795281002));
#30327=CARTESIAN_POINT('Ctrl Pts',(-1.57087397835723,1.,-1.31558903860016));
#30328=CARTESIAN_POINT('Ctrl Pts',(-1.5768005650559,1.,-1.31731642317187));
#30329=CARTESIAN_POINT('Ctrl Pts',(-1.58274907898834,1.,-1.31900135021432));
#30330=CARTESIAN_POINT('Ctrl Pts',(-1.58872057258245,1.,-1.32064537110892));
#30331=CARTESIAN_POINT('Ctrl Pts',(-1.59471591079403,1.,-1.32224985747682));
#30332=CARTESIAN_POINT('Ctrl Pts',(-1.60073511858687,1.,-1.32381550858256));
#30333=CARTESIAN_POINT('Ctrl Pts',(-1.60677758290954,1.,-1.32534250785782));
#30334=CARTESIAN_POINT('Ctrl Pts',(-1.6128423401575,1.,-1.32683074483356));
#30335=CARTESIAN_POINT('Ctrl Pts',(-1.61892832270724,1.,-1.32828000610449));
#30336=CARTESIAN_POINT('Ctrl Pts',(-1.62503464209797,1.,-1.3296901950568));
#30337=CARTESIAN_POINT('Ctrl Pts',(-1.63116079730923,1.,-1.33106149345645));
#30338=CARTESIAN_POINT('Ctrl Pts',(-1.63730653475089,1.,-1.33239425103724));
#30339=CARTESIAN_POINT('Ctrl Pts',(-1.6434717485603,1.,-1.33368890676572));
#30340=CARTESIAN_POINT('Ctrl Pts',(-1.6496563728683,1.,-1.33494590467993));
#30341=CARTESIAN_POINT('Ctrl Pts',(-1.65586025952593,1.,-1.33616559745172));
#30342=CARTESIAN_POINT('Ctrl Pts',(-1.66208312541983,1.,-1.33734820885262));
#30343=CARTESIAN_POINT('Ctrl Pts',(-1.66832460783989,1.,-1.33849388654388));
#30344=CARTESIAN_POINT('Ctrl Pts',(-1.67458429426086,1.,-1.3396027347034));
#30345=CARTESIAN_POINT('Ctrl Pts',(-1.68086176030362,1.,-1.34067485185203));
#30346=CARTESIAN_POINT('Ctrl Pts',(-1.68715660868764,1.,-1.341710374848));
#30347=CARTESIAN_POINT('Ctrl Pts',(-1.6934684849687,1.,-1.34270948206319));
#30348=CARTESIAN_POINT('Ctrl Pts',(-1.69979707754427,1.,-1.34367237124483));
#30349=CARTESIAN_POINT('Ctrl Pts',(-1.70614212266738,1.,-1.34459924533831));
#30350=CARTESIAN_POINT('Ctrl Pts',(-1.71250340686822,1.,-1.34549029589416));
#30351=CARTESIAN_POINT('Ctrl Pts',(-1.7188807715049,1.,-1.34634568653227));
#30352=CARTESIAN_POINT('Ctrl Pts',(-1.72527410680674,1.,-1.34716554819527));
#30353=CARTESIAN_POINT('Ctrl Pts',(-1.7304014965394,1.,-1.34779309152035));
#30354=CARTESIAN_POINT('Ctrl Pts',(-1.73425417885907,1.,-1.34824783112887));
#30355=CARTESIAN_POINT('Ctrl Pts',(-1.73682580585691,1.,-1.34854391898045));
#30356=CARTESIAN_POINT('Ctrl Pts',(-1.73811241238545,1.,-1.34869019493419));
#30357=CARTESIAN_POINT('',(-1.31362392696032,0.,-1.15624053661742));
#30358=CARTESIAN_POINT('Origin',(0.,0.,0.));
#30359=CARTESIAN_POINT('',(-1.15624053661742,1.,-1.31362392696033));
#30360=CARTESIAN_POINT('Origin',(0.,1.,0.));
#30361=CARTESIAN_POINT('',(-1.15624053661742,0.,-1.31362392696033));
#30362=CARTESIAN_POINT('Ctrl Pts',(-1.34869019493419,-1.,-1.73811241238545));
#30363=CARTESIAN_POINT('Ctrl Pts',(-1.34869019493419,1.,-1.73811241238545));
#30364=CARTESIAN_POINT('Ctrl Pts',(-1.34854391898145,-1.,-1.73682580585819));
#30365=CARTESIAN_POINT('Ctrl Pts',(-1.34854391898145,1.,-1.73682580585819));
#30366=CARTESIAN_POINT('Ctrl Pts',(-1.34824783113158,-1.,-1.73425417886255));
#30367=CARTESIAN_POINT('Ctrl Pts',(-1.34824783113158,1.,-1.73425417886255));
#30368=CARTESIAN_POINT('Ctrl Pts',(-1.3477930915247,-1.,-1.73040149654497));
#30369=CARTESIAN_POINT('Ctrl Pts',(-1.3477930915247,1.,-1.73040149654497));
#30370=CARTESIAN_POINT('Ctrl Pts',(-1.34716554820013,-1.,-1.72527410681298));
#30371=CARTESIAN_POINT('Ctrl Pts',(-1.34716554820013,1.,-1.72527410681298));
#30372=CARTESIAN_POINT('Ctrl Pts',(-1.34634568653586,-1.,-1.7188807715095));
#30373=CARTESIAN_POINT('Ctrl Pts',(-1.34634568653586,1.,-1.7188807715095));
#30374=CARTESIAN_POINT('Ctrl Pts',(-1.34549029589563,-1.,-1.71250340687011));
#30375=CARTESIAN_POINT('Ctrl Pts',(-1.34549029589563,1.,-1.71250340687011));
#30376=CARTESIAN_POINT('Ctrl Pts',(-1.34459924533783,-1.,-1.70614212266676));
#30377=CARTESIAN_POINT('Ctrl Pts',(-1.34459924533783,1.,-1.70614212266676));
#30378=CARTESIAN_POINT('Ctrl Pts',(-1.34367237124322,-1.,-1.69979707754221));
#30379=CARTESIAN_POINT('Ctrl Pts',(-1.34367237124322,1.,-1.69979707754221));
#30380=CARTESIAN_POINT('Ctrl Pts',(-1.34270948206139,-1.,-1.6934684849664));
#30381=CARTESIAN_POINT('Ctrl Pts',(-1.34270948206139,1.,-1.6934684849664));
#30382=CARTESIAN_POINT('Ctrl Pts',(-1.34171037484673,-1.,-1.68715660868602));
#30383=CARTESIAN_POINT('Ctrl Pts',(-1.34171037484673,1.,-1.68715660868602));
#30384=CARTESIAN_POINT('Ctrl Pts',(-1.3406748518516,-1.,-1.68086176030308));
#30385=CARTESIAN_POINT('Ctrl Pts',(-1.3406748518516,1.,-1.68086176030308));
#30386=CARTESIAN_POINT('Ctrl Pts',(-1.33960273470372,-1.,-1.67458429426126));
#30387=CARTESIAN_POINT('Ctrl Pts',(-1.33960273470372,1.,-1.67458429426126));
#30388=CARTESIAN_POINT('Ctrl Pts',(-1.33849388654458,-1.,-1.66832460784078));
#30389=CARTESIAN_POINT('Ctrl Pts',(-1.33849388654458,1.,-1.66832460784078));
#30390=CARTESIAN_POINT('Ctrl Pts',(-1.33734820885331,-1.,-1.66208312542073));
#30391=CARTESIAN_POINT('Ctrl Pts',(-1.33734820885331,1.,-1.66208312542073));
#30392=CARTESIAN_POINT('Ctrl Pts',(-1.33616559745217,-1.,-1.65586025952651));
#30393=CARTESIAN_POINT('Ctrl Pts',(-1.33616559745217,1.,-1.65586025952651));
#30394=CARTESIAN_POINT('Ctrl Pts',(-1.33494590468003,-1.,-1.64965637286843));
#30395=CARTESIAN_POINT('Ctrl Pts',(-1.33494590468003,1.,-1.64965637286843));
#30396=CARTESIAN_POINT('Ctrl Pts',(-1.33368890676554,-1.,-1.64347174856007));
#30397=CARTESIAN_POINT('Ctrl Pts',(-1.33368890676554,1.,-1.64347174856007));
#30398=CARTESIAN_POINT('Ctrl Pts',(-1.33239425103694,-1.,-1.6373065347505));
#30399=CARTESIAN_POINT('Ctrl Pts',(-1.33239425103694,1.,-1.6373065347505));
#30400=CARTESIAN_POINT('Ctrl Pts',(-1.33106149345618,-1.,-1.63116079730887));
#30401=CARTESIAN_POINT('Ctrl Pts',(-1.33106149345618,1.,-1.63116079730887));
#30402=CARTESIAN_POINT('Ctrl Pts',(-1.32969019505665,-1.,-1.62503464209777));
#30403=CARTESIAN_POINT('Ctrl Pts',(-1.32969019505665,1.,-1.62503464209777));
#30404=CARTESIAN_POINT('Ctrl Pts',(-1.32828000610448,-1.,-1.61892832270723));
#30405=CARTESIAN_POINT('Ctrl Pts',(-1.32828000610448,1.,-1.61892832270723));
#30406=CARTESIAN_POINT('Ctrl Pts',(-1.32683074483365,-1.,-1.61284234015762));
#30407=CARTESIAN_POINT('Ctrl Pts',(-1.32683074483365,1.,-1.61284234015762));
#30408=CARTESIAN_POINT('Ctrl Pts',(-1.32534250785794,-1.,-1.6067775829097));
#30409=CARTESIAN_POINT('Ctrl Pts',(-1.32534250785794,1.,-1.6067775829097));
#30410=CARTESIAN_POINT('Ctrl Pts',(-1.32381550858266,-1.,-1.600735118587));
#30411=CARTESIAN_POINT('Ctrl Pts',(-1.32381550858266,1.,-1.600735118587));
#30412=CARTESIAN_POINT('Ctrl Pts',(-1.32224985747686,-1.,-1.59471591079408));
#30413=CARTESIAN_POINT('Ctrl Pts',(-1.32224985747686,1.,-1.59471591079408));
#30414=CARTESIAN_POINT('Ctrl Pts',(-1.32064537110891,-1.,-1.58872057258244));
#30415=CARTESIAN_POINT('Ctrl Pts',(-1.32064537110891,1.,-1.58872057258244));
#30416=CARTESIAN_POINT('Ctrl Pts',(-1.31900135021428,-1.,-1.58274907898829));
#30417=CARTESIAN_POINT('Ctrl Pts',(-1.31900135021428,1.,-1.58274907898829));
#30418=CARTESIAN_POINT('Ctrl Pts',(-1.31731642317183,-1.,-1.57680056505585));
#30419=CARTESIAN_POINT('Ctrl Pts',(-1.31731642317183,1.,-1.57680056505585));
#30420=CARTESIAN_POINT('Ctrl Pts',(-1.31558903860015,-1.,-1.57087397835721));
#30421=CARTESIAN_POINT('Ctrl Pts',(-1.31558903860015,1.,-1.57087397835721));
#30422=CARTESIAN_POINT('Ctrl Pts',(-1.31381795281002,-1.,-1.56496872402352));
#30423=CARTESIAN_POINT('Ctrl Pts',(-1.31381795281002,1.,-1.56496872402352));
#30424=CARTESIAN_POINT('Ctrl Pts',(-1.31200264341696,-1.,-1.55908521254822));
#30425=CARTESIAN_POINT('Ctrl Pts',(-1.31200264341696,1.,-1.55908521254822));
#30426=CARTESIAN_POINT('Ctrl Pts',(-1.31014393684221,-1.,-1.55322568759481));
#30427=CARTESIAN_POINT('Ctrl Pts',(-1.31014393684221,1.,-1.55322568759481));
#30428=CARTESIAN_POINT('Ctrl Pts',(-1.30824393907471,-1.,-1.54739413957183));
#30429=CARTESIAN_POINT('Ctrl Pts',(-1.30824393907471,1.,-1.54739413957183));
#30430=CARTESIAN_POINT('Ctrl Pts',(-1.30630475189553,-1.,-1.54159462645428));
#30431=CARTESIAN_POINT('Ctrl Pts',(-1.30630475189553,1.,-1.54159462645428));
#30432=CARTESIAN_POINT('Ctrl Pts',(-1.30432735639487,-1.,-1.53582981268976));
#30433=CARTESIAN_POINT('Ctrl Pts',(-1.30432735639487,1.,-1.53582981268976));
#30434=CARTESIAN_POINT('Ctrl Pts',(-1.3023106439557,-1.,-1.53009970283893));
#30435=CARTESIAN_POINT('Ctrl Pts',(-1.3023106439557,1.,-1.53009970283893));
#30436=CARTESIAN_POINT('Ctrl Pts',(-1.30024984366334,-1.,-1.5243995786107));
#30437=CARTESIAN_POINT('Ctrl Pts',(-1.30024984366334,1.,-1.5243995786107));
#30438=CARTESIAN_POINT('Ctrl Pts',(-1.29813791800757,-1.,-1.51872184912735));
#30439=CARTESIAN_POINT('Ctrl Pts',(-1.29813791800757,1.,-1.51872184912735));
#30440=CARTESIAN_POINT('Ctrl Pts',(-1.29596850710518,-1.,-1.51305994241412));
#30441=CARTESIAN_POINT('Ctrl Pts',(-1.29596850710518,1.,-1.51305994241412));
#30442=CARTESIAN_POINT('Ctrl Pts',(-1.29373841372843,-1.,-1.50741159078367));
#30443=CARTESIAN_POINT('Ctrl Pts',(-1.29373841372843,1.,-1.50741159078367));
#30444=CARTESIAN_POINT('Ctrl Pts',(-1.29145022885171,-1.,-1.50178230149764));
#30445=CARTESIAN_POINT('Ctrl Pts',(-1.29145022885171,1.,-1.50178230149764));
#30446=CARTESIAN_POINT('Ctrl Pts',(-1.28911506584232,-1.,-1.49618896881729));
#30447=CARTESIAN_POINT('Ctrl Pts',(-1.28911506584232,1.,-1.49618896881729));
#30448=CARTESIAN_POINT('Ctrl Pts',(-1.28674676116415,-1.,-1.4906522831275));
#30449=CARTESIAN_POINT('Ctrl Pts',(-1.28674676116415,1.,-1.4906522831275));
#30450=CARTESIAN_POINT('Ctrl Pts',(-1.28435533880184,-1.,-1.48518817118891));
#30451=CARTESIAN_POINT('Ctrl Pts',(-1.28435533880184,1.,-1.48518817118891));
#30452=CARTESIAN_POINT('Ctrl Pts',(-1.28194158939522,-1.,-1.47980070347102));
#30453=CARTESIAN_POINT('Ctrl Pts',(-1.28194158939522,1.,-1.47980070347102));
#30454=CARTESIAN_POINT('Ctrl Pts',(-1.27948918248524,-1.,-1.4744717526711));
#30455=CARTESIAN_POINT('Ctrl Pts',(-1.27948918248524,1.,-1.4744717526711));
#30456=CARTESIAN_POINT('Ctrl Pts',(-1.27696414831144,-1.,-1.46916035917197));
#30457=CARTESIAN_POINT('Ctrl Pts',(-1.27696414831144,1.,-1.46916035917197));
#30458=CARTESIAN_POINT('Ctrl Pts',(-1.27433119897877,-1.,-1.4638243133254));
#30459=CARTESIAN_POINT('Ctrl Pts',(-1.27433119897877,1.,-1.4638243133254));
#30460=CARTESIAN_POINT('Ctrl Pts',(-1.27156805265312,-1.,-1.45843906294725));
#30461=CARTESIAN_POINT('Ctrl Pts',(-1.27156805265312,1.,-1.45843906294725));
#30462=CARTESIAN_POINT('Ctrl Pts',(-1.26867786804854,-1.,-1.45301422764205));
#30463=CARTESIAN_POINT('Ctrl Pts',(-1.26867786804854,1.,-1.45301422764205));
#30464=CARTESIAN_POINT('Ctrl Pts',(-1.26570925118767,-1.,-1.44761985001544));
#30465=CARTESIAN_POINT('Ctrl Pts',(-1.26570925118767,1.,-1.44761985001544));
#30466=CARTESIAN_POINT('Ctrl Pts',(-1.26273903323723,-1.,-1.44236470511145));
#30467=CARTESIAN_POINT('Ctrl Pts',(-1.26273903323723,1.,-1.44236470511145));
#30468=CARTESIAN_POINT('Ctrl Pts',(-1.25983531011894,-1.,-1.43734919180719));
#30469=CARTESIAN_POINT('Ctrl Pts',(-1.25983531011894,1.,-1.43734919180719));
#30470=CARTESIAN_POINT('Ctrl Pts',(-1.25702687965744,-1.,-1.43262645609679));
#30471=CARTESIAN_POINT('Ctrl Pts',(-1.25702687965744,1.,-1.43262645609679));
#30472=CARTESIAN_POINT('Ctrl Pts',(-1.25426945222783,-1.,-1.42815938799555));
#30473=CARTESIAN_POINT('Ctrl Pts',(-1.25426945222783,1.,-1.42815938799555));
#30474=CARTESIAN_POINT('Ctrl Pts',(-1.25141455570299,-1.,-1.42378102115911));
#30475=CARTESIAN_POINT('Ctrl Pts',(-1.25141455570299,1.,-1.42378102115911));
#30476=CARTESIAN_POINT('Ctrl Pts',(-1.24824430986911,-1.,-1.41923722596421));
#30477=CARTESIAN_POINT('Ctrl Pts',(-1.24824430986911,1.,-1.41923722596421));
#30478=CARTESIAN_POINT('Ctrl Pts',(-1.24450600513278,-1.,-1.41422913175437));
#30479=CARTESIAN_POINT('Ctrl Pts',(-1.24450600513278,1.,-1.41422913175437));
#30480=CARTESIAN_POINT('Ctrl Pts',(-1.23994455029421,-1.,-1.40845295531151));
#30481=CARTESIAN_POINT('Ctrl Pts',(-1.23994455029421,1.,-1.40845295531151));
#30482=CARTESIAN_POINT('Ctrl Pts',(-1.23434087289768,-1.,-1.40164708205345));
#30483=CARTESIAN_POINT('Ctrl Pts',(-1.23434087289768,1.,-1.40164708205345));
#30484=CARTESIAN_POINT('Ctrl Pts',(-1.22752961898063,-1.,-1.39361389567257));
#30485=CARTESIAN_POINT('Ctrl Pts',(-1.22752961898063,1.,-1.39361389567257));
#30486=CARTESIAN_POINT('Ctrl Pts',(-1.21938737278853,-1.,-1.38420564525391));
#30487=CARTESIAN_POINT('Ctrl Pts',(-1.21938737278853,1.,-1.38420564525391));
#30488=CARTESIAN_POINT('Ctrl Pts',(-1.20982812923113,-1.,-1.37331915604962));
#30489=CARTESIAN_POINT('Ctrl Pts',(-1.20982812923113,1.,-1.37331915604962));
#30490=CARTESIAN_POINT('Ctrl Pts',(-1.1987959077656,-1.,-1.36088705040677));
#30491=CARTESIAN_POINT('Ctrl Pts',(-1.1987959077656,1.,-1.36088705040677));
#30492=CARTESIAN_POINT('Ctrl Pts',(-1.18625865664915,-1.,-1.34687053998157));
#30493=CARTESIAN_POINT('Ctrl Pts',(-1.18625865664915,1.,-1.34687053998157));
#30494=CARTESIAN_POINT('Ctrl Pts',(-1.17501305787994,-1.,-1.33437539344842));
#30495=CARTESIAN_POINT('Ctrl Pts',(-1.17501305787994,1.,-1.33437539344842));
#30496=CARTESIAN_POINT('Ctrl Pts',(-1.16589330092532,-1.,-1.32428080720544));
#30497=CARTESIAN_POINT('Ctrl Pts',(-1.16589330092532,1.,-1.32428080720544));
#30498=CARTESIAN_POINT('Ctrl Pts',(-1.15950888730433,-1.,-1.3172297721596));
#30499=CARTESIAN_POINT('Ctrl Pts',(-1.15950888730433,1.,-1.3172297721596));
#30500=CARTESIAN_POINT('Ctrl Pts',(-1.15624053661742,-1.,-1.31362392696033));
#30501=CARTESIAN_POINT('Ctrl Pts',(-1.15624053661742,1.,-1.31362392696033));
#30502=CARTESIAN_POINT('',(-1.34869019493419,1.,-1.73811241238545));
#30503=CARTESIAN_POINT('Ctrl Pts',(-1.34869019493419,1.,-1.73811241238545));
#30504=CARTESIAN_POINT('Ctrl Pts',(-1.34854391898145,1.,-1.73682580585819));
#30505=CARTESIAN_POINT('Ctrl Pts',(-1.34824783113158,1.,-1.73425417886255));
#30506=CARTESIAN_POINT('Ctrl Pts',(-1.3477930915247,1.,-1.73040149654497));
#30507=CARTESIAN_POINT('Ctrl Pts',(-1.34716554820013,1.,-1.72527410681298));
#30508=CARTESIAN_POINT('Ctrl Pts',(-1.34634568653586,1.,-1.7188807715095));
#30509=CARTESIAN_POINT('Ctrl Pts',(-1.34549029589563,1.,-1.71250340687011));
#30510=CARTESIAN_POINT('Ctrl Pts',(-1.34459924533783,1.,-1.70614212266676));
#30511=CARTESIAN_POINT('Ctrl Pts',(-1.34367237124322,1.,-1.69979707754221));
#30512=CARTESIAN_POINT('Ctrl Pts',(-1.34270948206139,1.,-1.6934684849664));
#30513=CARTESIAN_POINT('Ctrl Pts',(-1.34171037484673,1.,-1.68715660868602));
#30514=CARTESIAN_POINT('Ctrl Pts',(-1.3406748518516,1.,-1.68086176030308));
#30515=CARTESIAN_POINT('Ctrl Pts',(-1.33960273470372,1.,-1.67458429426126));
#30516=CARTESIAN_POINT('Ctrl Pts',(-1.33849388654458,1.,-1.66832460784078));
#30517=CARTESIAN_POINT('Ctrl Pts',(-1.33734820885331,1.,-1.66208312542073));
#30518=CARTESIAN_POINT('Ctrl Pts',(-1.33616559745217,1.,-1.65586025952651));
#30519=CARTESIAN_POINT('Ctrl Pts',(-1.33494590468003,1.,-1.64965637286843));
#30520=CARTESIAN_POINT('Ctrl Pts',(-1.33368890676554,1.,-1.64347174856007));
#30521=CARTESIAN_POINT('Ctrl Pts',(-1.33239425103694,1.,-1.6373065347505));
#30522=CARTESIAN_POINT('Ctrl Pts',(-1.33106149345618,1.,-1.63116079730887));
#30523=CARTESIAN_POINT('Ctrl Pts',(-1.32969019505665,1.,-1.62503464209777));
#30524=CARTESIAN_POINT('Ctrl Pts',(-1.32828000610448,1.,-1.61892832270723));
#30525=CARTESIAN_POINT('Ctrl Pts',(-1.32683074483365,1.,-1.61284234015762));
#30526=CARTESIAN_POINT('Ctrl Pts',(-1.32534250785794,1.,-1.6067775829097));
#30527=CARTESIAN_POINT('Ctrl Pts',(-1.32381550858266,1.,-1.600735118587));
#30528=CARTESIAN_POINT('Ctrl Pts',(-1.32224985747686,1.,-1.59471591079408));
#30529=CARTESIAN_POINT('Ctrl Pts',(-1.32064537110891,1.,-1.58872057258244));
#30530=CARTESIAN_POINT('Ctrl Pts',(-1.31900135021428,1.,-1.58274907898829));
#30531=CARTESIAN_POINT('Ctrl Pts',(-1.31731642317183,1.,-1.57680056505585));
#30532=CARTESIAN_POINT('Ctrl Pts',(-1.31558903860015,1.,-1.57087397835721));
#30533=CARTESIAN_POINT('Ctrl Pts',(-1.31381795281002,1.,-1.56496872402352));
#30534=CARTESIAN_POINT('Ctrl Pts',(-1.31200264341696,1.,-1.55908521254822));
#30535=CARTESIAN_POINT('Ctrl Pts',(-1.31014393684221,1.,-1.55322568759481));
#30536=CARTESIAN_POINT('Ctrl Pts',(-1.30824393907471,1.,-1.54739413957183));
#30537=CARTESIAN_POINT('Ctrl Pts',(-1.30630475189553,1.,-1.54159462645428));
#30538=CARTESIAN_POINT('Ctrl Pts',(-1.30432735639487,1.,-1.53582981268976));
#30539=CARTESIAN_POINT('Ctrl Pts',(-1.3023106439557,1.,-1.53009970283893));
#30540=CARTESIAN_POINT('Ctrl Pts',(-1.30024984366334,1.,-1.5243995786107));
#30541=CARTESIAN_POINT('Ctrl Pts',(-1.29813791800757,1.,-1.51872184912735));
#30542=CARTESIAN_POINT('Ctrl Pts',(-1.29596850710518,1.,-1.51305994241412));
#30543=CARTESIAN_POINT('Ctrl Pts',(-1.29373841372843,1.,-1.50741159078367));
#30544=CARTESIAN_POINT('Ctrl Pts',(-1.29145022885171,1.,-1.50178230149764));
#30545=CARTESIAN_POINT('Ctrl Pts',(-1.28911506584232,1.,-1.49618896881729));
#30546=CARTESIAN_POINT('Ctrl Pts',(-1.28674676116415,1.,-1.4906522831275));
#30547=CARTESIAN_POINT('Ctrl Pts',(-1.28435533880184,1.,-1.48518817118891));
#30548=CARTESIAN_POINT('Ctrl Pts',(-1.28194158939522,1.,-1.47980070347102));
#30549=CARTESIAN_POINT('Ctrl Pts',(-1.27948918248524,1.,-1.4744717526711));
#30550=CARTESIAN_POINT('Ctrl Pts',(-1.27696414831144,1.,-1.46916035917197));
#30551=CARTESIAN_POINT('Ctrl Pts',(-1.27433119897877,1.,-1.4638243133254));
#30552=CARTESIAN_POINT('Ctrl Pts',(-1.27156805265312,1.,-1.45843906294725));
#30553=CARTESIAN_POINT('Ctrl Pts',(-1.26867786804854,1.,-1.45301422764205));
#30554=CARTESIAN_POINT('Ctrl Pts',(-1.26570925118767,1.,-1.44761985001544));
#30555=CARTESIAN_POINT('Ctrl Pts',(-1.26273903323723,1.,-1.44236470511145));
#30556=CARTESIAN_POINT('Ctrl Pts',(-1.25983531011894,1.,-1.43734919180719));
#30557=CARTESIAN_POINT('Ctrl Pts',(-1.25702687965744,1.,-1.43262645609679));
#30558=CARTESIAN_POINT('Ctrl Pts',(-1.25426945222783,1.,-1.42815938799555));
#30559=CARTESIAN_POINT('Ctrl Pts',(-1.25141455570299,1.,-1.42378102115911));
#30560=CARTESIAN_POINT('Ctrl Pts',(-1.24824430986911,1.,-1.41923722596421));
#30561=CARTESIAN_POINT('Ctrl Pts',(-1.24450600513278,1.,-1.41422913175437));
#30562=CARTESIAN_POINT('Ctrl Pts',(-1.23994455029421,1.,-1.40845295531151));
#30563=CARTESIAN_POINT('Ctrl Pts',(-1.23434087289768,1.,-1.40164708205345));
#30564=CARTESIAN_POINT('Ctrl Pts',(-1.22752961898063,1.,-1.39361389567257));
#30565=CARTESIAN_POINT('Ctrl Pts',(-1.21938737278853,1.,-1.38420564525391));
#30566=CARTESIAN_POINT('Ctrl Pts',(-1.20982812923113,1.,-1.37331915604962));
#30567=CARTESIAN_POINT('Ctrl Pts',(-1.1987959077656,1.,-1.36088705040677));
#30568=CARTESIAN_POINT('Ctrl Pts',(-1.18625865664915,1.,-1.34687053998157));
#30569=CARTESIAN_POINT('Ctrl Pts',(-1.17501305787994,1.,-1.33437539344842));
#30570=CARTESIAN_POINT('Ctrl Pts',(-1.16589330092532,1.,-1.32428080720544));
#30571=CARTESIAN_POINT('Ctrl Pts',(-1.15950888730433,1.,-1.3172297721596));
#30572=CARTESIAN_POINT('Ctrl Pts',(-1.15624053661742,1.,-1.31362392696033));
#30573=CARTESIAN_POINT('',(-1.34869019493419,0.,-1.73811241238545));
#30574=CARTESIAN_POINT('Origin',(-1.23627494547115,0.,-1.81978687191668));
#30575=CARTESIAN_POINT('',(-1.23627494547115,1.,-1.81978687191668));
#30576=CARTESIAN_POINT('',(-1.34869019493419,1.,-1.73811241238545));
#30577=CARTESIAN_POINT('',(-1.23627494547115,0.,-1.81978687191668));
#30578=CARTESIAN_POINT('Ctrl Pts',(-0.892032620296855,-1.,-1.5055822144029));
#30579=CARTESIAN_POINT('Ctrl Pts',(-0.892032620296855,1.,-1.5055822144029));
#30580=CARTESIAN_POINT('Ctrl Pts',(-0.894452006967538,-1.,-1.50980486807181));
#30581=CARTESIAN_POINT('Ctrl Pts',(-0.894452006967538,1.,-1.50980486807181));
#30582=CARTESIAN_POINT('Ctrl Pts',(-0.89918504749193,-1.,-1.51805569591479));
#30583=CARTESIAN_POINT('Ctrl Pts',(-0.89918504749193,1.,-1.51805569591479));
#30584=CARTESIAN_POINT('Ctrl Pts',(-0.905967409640499,-1.,-1.52984849890434));
#30585=CARTESIAN_POINT('Ctrl Pts',(-0.905967409640499,1.,-1.52984849890434));
#30586=CARTESIAN_POINT('Ctrl Pts',(-0.91437591904658,-1.,-1.54440491152808));
#30587=CARTESIAN_POINT('Ctrl Pts',(-0.91437591904658,1.,-1.54440491152808));
#30588=CARTESIAN_POINT('Ctrl Pts',(-0.923832188966322,-1.,-1.56065988582509));
#30589=CARTESIAN_POINT('Ctrl Pts',(-0.923832188966322,1.,-1.56065988582509));
#30590=CARTESIAN_POINT('Ctrl Pts',(-0.932246680128849,-1.,-1.57499388385561));
#30591=CARTESIAN_POINT('Ctrl Pts',(-0.932246680128849,1.,-1.57499388385561));
#30592=CARTESIAN_POINT('Ctrl Pts',(-0.939646377909319,-1.,-1.58744937489796));
#30593=CARTESIAN_POINT('Ctrl Pts',(-0.939646377909319,1.,-1.58744937489796));
#30594=CARTESIAN_POINT('Ctrl Pts',(-0.946078063325796,-1.,-1.59810042045408));
#30595=CARTESIAN_POINT('Ctrl Pts',(-0.946078063325796,1.,-1.59810042045408));
#30596=CARTESIAN_POINT('Ctrl Pts',(-0.951613284361248,-1.,-1.60706069897794));
#30597=CARTESIAN_POINT('Ctrl Pts',(-0.951613284361248,1.,-1.60706069897794));
#30598=CARTESIAN_POINT('Ctrl Pts',(-0.956354422921573,-1.,-1.61449324337233));
#30599=CARTESIAN_POINT('Ctrl Pts',(-0.956354422921573,1.,-1.61449324337233));
#30600=CARTESIAN_POINT('Ctrl Pts',(-0.960438326099958,-1.,-1.62061638139929));
#30601=CARTESIAN_POINT('Ctrl Pts',(-0.960438326099958,1.,-1.62061638139929));
#30602=CARTESIAN_POINT('Ctrl Pts',(-0.964046107037821,-1.,-1.6257193066974));
#30603=CARTESIAN_POINT('Ctrl Pts',(-0.964046107037821,1.,-1.6257193066974));
#30604=CARTESIAN_POINT('Ctrl Pts',(-0.967387853228041,-1.,-1.63013849959083));
#30605=CARTESIAN_POINT('Ctrl Pts',(-0.967387853228041,1.,-1.63013849959083));
#30606=CARTESIAN_POINT('Ctrl Pts',(-0.970669715996356,-1.,-1.63420665729609));
#30607=CARTESIAN_POINT('Ctrl Pts',(-0.970669715996356,1.,-1.63420665729609));
#30608=CARTESIAN_POINT('Ctrl Pts',(-0.974066058287501,-1.,-1.63820952658157));
#30609=CARTESIAN_POINT('Ctrl Pts',(-0.974066058287501,1.,-1.63820952658157));
#30610=CARTESIAN_POINT('Ctrl Pts',(-0.977689794120297,-1.,-1.64233990826831));
#30611=CARTESIAN_POINT('Ctrl Pts',(-0.977689794120297,1.,-1.64233990826831));
#30612=CARTESIAN_POINT('Ctrl Pts',(-0.981562530940574,-1.,-1.64665139190834));
#30613=CARTESIAN_POINT('Ctrl Pts',(-0.981562530940574,1.,-1.64665139190834));
#30614=CARTESIAN_POINT('Ctrl Pts',(-0.985642622921626,-1.,-1.6511001661277));
#30615=CARTESIAN_POINT('Ctrl Pts',(-0.985642622921626,1.,-1.6511001661277));
#30616=CARTESIAN_POINT('Ctrl Pts',(-0.98985562785445,-1.,-1.65559044289746));
#30617=CARTESIAN_POINT('Ctrl Pts',(-0.98985562785445,1.,-1.65559044289746));
#30618=CARTESIAN_POINT('Ctrl Pts',(-0.994121836661116,-1.,-1.66001553809916));
#30619=CARTESIAN_POINT('Ctrl Pts',(-0.994121836661116,1.,-1.66001553809916));
#30620=CARTESIAN_POINT('Ctrl Pts',(-0.998389654952317,-1.,-1.66430758030304));
#30621=CARTESIAN_POINT('Ctrl Pts',(-0.998389654952317,1.,-1.66430758030304));
#30622=CARTESIAN_POINT('Ctrl Pts',(-1.00265091003682,-1.,-1.66846059277231));
#30623=CARTESIAN_POINT('Ctrl Pts',(-1.00265091003682,1.,-1.66846059277231));
#30624=CARTESIAN_POINT('Ctrl Pts',(-1.00692206696387,-1.,-1.67250335383248));
#30625=CARTESIAN_POINT('Ctrl Pts',(-1.00692206696387,1.,-1.67250335383248));
#30626=CARTESIAN_POINT('Ctrl Pts',(-1.01123236493507,-1.,-1.67648246776457));
#30627=CARTESIAN_POINT('Ctrl Pts',(-1.01123236493507,1.,-1.67648246776457));
#30628=CARTESIAN_POINT('Ctrl Pts',(-1.01561026162787,-1.,-1.6804428989482));
#30629=CARTESIAN_POINT('Ctrl Pts',(-1.01561026162787,1.,-1.6804428989482));
#30630=CARTESIAN_POINT('Ctrl Pts',(-1.02006795074222,-1.,-1.68440578021739));
#30631=CARTESIAN_POINT('Ctrl Pts',(-1.02006795074222,1.,-1.68440578021739));
#30632=CARTESIAN_POINT('Ctrl Pts',(-1.02460180535272,-1.,-1.68836910178475));
#30633=CARTESIAN_POINT('Ctrl Pts',(-1.02460180535272,1.,-1.68836910178475));
#30634=CARTESIAN_POINT('Ctrl Pts',(-1.02919977579155,-1.,-1.69231840863471));
#30635=CARTESIAN_POINT('Ctrl Pts',(-1.02919977579155,1.,-1.69231840863471));
#30636=CARTESIAN_POINT('Ctrl Pts',(-1.03384646003587,-1.,-1.69623414782769));
#30637=CARTESIAN_POINT('Ctrl Pts',(-1.03384646003587,1.,-1.69623414782769));
#30638=CARTESIAN_POINT('Ctrl Pts',(-1.03852922490782,-1.,-1.70010052930951));
#30639=CARTESIAN_POINT('Ctrl Pts',(-1.03852922490782,1.,-1.70010052930951));
#30640=CARTESIAN_POINT('Ctrl Pts',(-1.04324363334546,-1.,-1.70391338707969));
#30641=CARTESIAN_POINT('Ctrl Pts',(-1.04324363334546,1.,-1.70391338707969));
#30642=CARTESIAN_POINT('Ctrl Pts',(-1.0479908540499,-1.,-1.70767646263641));
#30643=CARTESIAN_POINT('Ctrl Pts',(-1.0479908540499,1.,-1.70767646263641));
#30644=CARTESIAN_POINT('Ctrl Pts',(-1.05277517202854,-1.,-1.71139783543986));
#30645=CARTESIAN_POINT('Ctrl Pts',(-1.05277517202854,1.,-1.71139783543986));
#30646=CARTESIAN_POINT('Ctrl Pts',(-1.05760163192481,-1.,-1.71508654427022));
#30647=CARTESIAN_POINT('Ctrl Pts',(-1.05760163192481,1.,-1.71508654427022));
#30648=CARTESIAN_POINT('Ctrl Pts',(-1.0624732468065,-1.,-1.71874858456908));
#30649=CARTESIAN_POINT('Ctrl Pts',(-1.0624732468065,1.,-1.71874858456908));
#30650=CARTESIAN_POINT('Ctrl Pts',(-1.06738966975463,-1.,-1.72238500928456));
#30651=CARTESIAN_POINT('Ctrl Pts',(-1.06738966975463,1.,-1.72238500928456));
#30652=CARTESIAN_POINT('Ctrl Pts',(-1.07234866990252,-1.,-1.72599406198489));
#30653=CARTESIAN_POINT('Ctrl Pts',(-1.07234866990252,1.,-1.72599406198489));
#30654=CARTESIAN_POINT('Ctrl Pts',(-1.0773470373727,-1.,-1.72957248977424));
#30655=CARTESIAN_POINT('Ctrl Pts',(-1.0773470373727,1.,-1.72957248977424));
#30656=CARTESIAN_POINT('Ctrl Pts',(-1.08238162784749,-1.,-1.73311705663407));
#30657=CARTESIAN_POINT('Ctrl Pts',(-1.08238162784749,1.,-1.73311705663407));
#30658=CARTESIAN_POINT('Ctrl Pts',(-1.08745056285429,-1.,-1.73662628326093));
#30659=CARTESIAN_POINT('Ctrl Pts',(-1.08745056285429,1.,-1.73662628326093));
#30660=CARTESIAN_POINT('Ctrl Pts',(-1.09255329056496,-1.,-1.74010053962252));
#30661=CARTESIAN_POINT('Ctrl Pts',(-1.09255329056496,1.,-1.74010053962252));
#30662=CARTESIAN_POINT('Ctrl Pts',(-1.09768999241229,-1.,-1.74354119236212));
#30663=CARTESIAN_POINT('Ctrl Pts',(-1.09768999241229,1.,-1.74354119236212));
#30664=CARTESIAN_POINT('Ctrl Pts',(-1.10286118991144,-1.,-1.74695004214924));
#30665=CARTESIAN_POINT('Ctrl Pts',(-1.10286118991144,1.,-1.74695004214924));
#30666=CARTESIAN_POINT('Ctrl Pts',(-1.10806728183003,-1.,-1.75032866075914));
#30667=CARTESIAN_POINT('Ctrl Pts',(-1.10806728183003,1.,-1.75032866075914));
#30668=CARTESIAN_POINT('Ctrl Pts',(-1.11330807582542,-1.,-1.75367772094617));
#30669=CARTESIAN_POINT('Ctrl Pts',(-1.11330807582542,1.,-1.75367772094617));
#30670=CARTESIAN_POINT('Ctrl Pts',(-1.11858293216752,-1.,-1.75699720772089));
#30671=CARTESIAN_POINT('Ctrl Pts',(-1.11858293216752,1.,-1.75699720772089));
#30672=CARTESIAN_POINT('Ctrl Pts',(-1.12389096855078,-1.,-1.76028671825084));
#30673=CARTESIAN_POINT('Ctrl Pts',(-1.12389096855078,1.,-1.76028671825084));
#30674=CARTESIAN_POINT('Ctrl Pts',(-1.12923123555076,-1.,-1.76354571966171));
#30675=CARTESIAN_POINT('Ctrl Pts',(-1.12923123555076,1.,-1.76354571966171));
#30676=CARTESIAN_POINT('Ctrl Pts',(-1.13460291804635,-1.,-1.76677384551883));
#30677=CARTESIAN_POINT('Ctrl Pts',(-1.13460291804635,1.,-1.76677384551883));
#30678=CARTESIAN_POINT('Ctrl Pts',(-1.14000548337,-1.,-1.76997111386806));
#30679=CARTESIAN_POINT('Ctrl Pts',(-1.14000548337,1.,-1.76997111386806));
#30680=CARTESIAN_POINT('Ctrl Pts',(-1.14543858226948,-1.,-1.77313777896234));
#30681=CARTESIAN_POINT('Ctrl Pts',(-1.14543858226948,1.,-1.77313777896234));
#30682=CARTESIAN_POINT('Ctrl Pts',(-1.15090197841531,-1.,-1.77627422557034));
#30683=CARTESIAN_POINT('Ctrl Pts',(-1.15090197841531,1.,-1.77627422557034));
#30684=CARTESIAN_POINT('Ctrl Pts',(-1.15639547194689,-1.,-1.77938085564261));
#30685=CARTESIAN_POINT('Ctrl Pts',(-1.15639547194689,1.,-1.77938085564261));
#30686=CARTESIAN_POINT('Ctrl Pts',(-1.16191881298458,-1.,-1.78245795880949));
#30687=CARTESIAN_POINT('Ctrl Pts',(-1.16191881298458,1.,-1.78245795880949));
#30688=CARTESIAN_POINT('Ctrl Pts',(-1.16747166312239,-1.,-1.78550566040349));
#30689=CARTESIAN_POINT('Ctrl Pts',(-1.16747166312239,1.,-1.78550566040349));
#30690=CARTESIAN_POINT('Ctrl Pts',(-1.17305363177265,-1.,-1.78852398877523));
#30691=CARTESIAN_POINT('Ctrl Pts',(-1.17305363177265,1.,-1.78852398877523));
#30692=CARTESIAN_POINT('Ctrl Pts',(-1.17866429440781,-1.,-1.79151291552646));
#30693=CARTESIAN_POINT('Ctrl Pts',(-1.17866429440781,1.,-1.79151291552646));
#30694=CARTESIAN_POINT('Ctrl Pts',(-1.18430321697471,-1.,-1.79447240321572));
#30695=CARTESIAN_POINT('Ctrl Pts',(-1.18430321697471,1.,-1.79447240321572));
#30696=CARTESIAN_POINT('Ctrl Pts',(-1.1899699793456,-1.,-1.79740245923649));
#30697=CARTESIAN_POINT('Ctrl Pts',(-1.1899699793456,1.,-1.79740245923649));
#30698=CARTESIAN_POINT('Ctrl Pts',(-1.19566418930405,-1.,-1.80030314370121));
#30699=CARTESIAN_POINT('Ctrl Pts',(-1.19566418930405,1.,-1.80030314370121));
#30700=CARTESIAN_POINT('Ctrl Pts',(-1.2013854893912,-1.,-1.8031745483882));
#30701=CARTESIAN_POINT('Ctrl Pts',(-1.2013854893912,1.,-1.8031745483882));
#30702=CARTESIAN_POINT('Ctrl Pts',(-1.20713356605519,-1.,-1.80601678480772));
#30703=CARTESIAN_POINT('Ctrl Pts',(-1.20713356605519,1.,-1.80601678480772));
#30704=CARTESIAN_POINT('Ctrl Pts',(-1.2129081570818,-1.,-1.80882996916931));
#30705=CARTESIAN_POINT('Ctrl Pts',(-1.2129081570818,1.,-1.80882996916931));
#30706=CARTESIAN_POINT('Ctrl Pts',(-1.2187090610323,-1.,-1.81161420806172));
#30707=CARTESIAN_POINT('Ctrl Pts',(-1.2187090610323,1.,-1.81161420806172));
#30708=CARTESIAN_POINT('Ctrl Pts',(-1.22453613304507,-1.,-1.81436959209778));
#30709=CARTESIAN_POINT('Ctrl Pts',(-1.22453613304507,1.,-1.81436959209778));
#30710=CARTESIAN_POINT('Ctrl Pts',(-1.22921864890975,-1.,-1.81655087183054));
#30711=CARTESIAN_POINT('Ctrl Pts',(-1.22921864890975,1.,-1.81655087183054));
#30712=CARTESIAN_POINT('Ctrl Pts',(-1.23274224526804,-1.,-1.81817389920914));
#30713=CARTESIAN_POINT('Ctrl Pts',(-1.23274224526804,1.,-1.81817389920914));
#30714=CARTESIAN_POINT('Ctrl Pts',(-1.23509651170384,-1.,-1.81925017193531));
#30715=CARTESIAN_POINT('Ctrl Pts',(-1.23509651170384,1.,-1.81925017193531));
#30716=CARTESIAN_POINT('Ctrl Pts',(-1.23627494547115,-1.,-1.81978687191668));
#30717=CARTESIAN_POINT('Ctrl Pts',(-1.23627494547115,1.,-1.81978687191668));
#30718=CARTESIAN_POINT('',(-0.892032620296855,1.,-1.5055822144029));
#30719=CARTESIAN_POINT('Ctrl Pts',(-0.892032620296855,1.,-1.5055822144029));
#30720=CARTESIAN_POINT('Ctrl Pts',(-0.894452006967538,1.,-1.50980486807181));
#30721=CARTESIAN_POINT('Ctrl Pts',(-0.89918504749193,1.,-1.51805569591479));
#30722=CARTESIAN_POINT('Ctrl Pts',(-0.905967409640499,1.,-1.52984849890434));
#30723=CARTESIAN_POINT('Ctrl Pts',(-0.91437591904658,1.,-1.54440491152808));
#30724=CARTESIAN_POINT('Ctrl Pts',(-0.923832188966322,1.,-1.56065988582509));
#30725=CARTESIAN_POINT('Ctrl Pts',(-0.932246680128849,1.,-1.57499388385561));
#30726=CARTESIAN_POINT('Ctrl Pts',(-0.939646377909319,1.,-1.58744937489796));
#30727=CARTESIAN_POINT('Ctrl Pts',(-0.946078063325796,1.,-1.59810042045408));
#30728=CARTESIAN_POINT('Ctrl Pts',(-0.951613284361248,1.,-1.60706069897794));
#30729=CARTESIAN_POINT('Ctrl Pts',(-0.956354422921573,1.,-1.61449324337233));
#30730=CARTESIAN_POINT('Ctrl Pts',(-0.960438326099958,1.,-1.62061638139929));
#30731=CARTESIAN_POINT('Ctrl Pts',(-0.964046107037821,1.,-1.6257193066974));
#30732=CARTESIAN_POINT('Ctrl Pts',(-0.967387853228041,1.,-1.63013849959083));
#30733=CARTESIAN_POINT('Ctrl Pts',(-0.970669715996356,1.,-1.63420665729609));
#30734=CARTESIAN_POINT('Ctrl Pts',(-0.974066058287501,1.,-1.63820952658157));
#30735=CARTESIAN_POINT('Ctrl Pts',(-0.977689794120297,1.,-1.64233990826831));
#30736=CARTESIAN_POINT('Ctrl Pts',(-0.981562530940574,1.,-1.64665139190834));
#30737=CARTESIAN_POINT('Ctrl Pts',(-0.985642622921626,1.,-1.6511001661277));
#30738=CARTESIAN_POINT('Ctrl Pts',(-0.98985562785445,1.,-1.65559044289746));
#30739=CARTESIAN_POINT('Ctrl Pts',(-0.994121836661116,1.,-1.66001553809916));
#30740=CARTESIAN_POINT('Ctrl Pts',(-0.998389654952317,1.,-1.66430758030304));
#30741=CARTESIAN_POINT('Ctrl Pts',(-1.00265091003682,1.,-1.66846059277231));
#30742=CARTESIAN_POINT('Ctrl Pts',(-1.00692206696387,1.,-1.67250335383248));
#30743=CARTESIAN_POINT('Ctrl Pts',(-1.01123236493507,1.,-1.67648246776457));
#30744=CARTESIAN_POINT('Ctrl Pts',(-1.01561026162787,1.,-1.6804428989482));
#30745=CARTESIAN_POINT('Ctrl Pts',(-1.02006795074222,1.,-1.68440578021739));
#30746=CARTESIAN_POINT('Ctrl Pts',(-1.02460180535272,1.,-1.68836910178475));
#30747=CARTESIAN_POINT('Ctrl Pts',(-1.02919977579155,1.,-1.69231840863471));
#30748=CARTESIAN_POINT('Ctrl Pts',(-1.03384646003587,1.,-1.69623414782769));
#30749=CARTESIAN_POINT('Ctrl Pts',(-1.03852922490782,1.,-1.70010052930951));
#30750=CARTESIAN_POINT('Ctrl Pts',(-1.04324363334546,1.,-1.70391338707969));
#30751=CARTESIAN_POINT('Ctrl Pts',(-1.0479908540499,1.,-1.70767646263641));
#30752=CARTESIAN_POINT('Ctrl Pts',(-1.05277517202854,1.,-1.71139783543986));
#30753=CARTESIAN_POINT('Ctrl Pts',(-1.05760163192481,1.,-1.71508654427022));
#30754=CARTESIAN_POINT('Ctrl Pts',(-1.0624732468065,1.,-1.71874858456908));
#30755=CARTESIAN_POINT('Ctrl Pts',(-1.06738966975463,1.,-1.72238500928456));
#30756=CARTESIAN_POINT('Ctrl Pts',(-1.07234866990252,1.,-1.72599406198489));
#30757=CARTESIAN_POINT('Ctrl Pts',(-1.0773470373727,1.,-1.72957248977424));
#30758=CARTESIAN_POINT('Ctrl Pts',(-1.08238162784749,1.,-1.73311705663407));
#30759=CARTESIAN_POINT('Ctrl Pts',(-1.08745056285429,1.,-1.73662628326093));
#30760=CARTESIAN_POINT('Ctrl Pts',(-1.09255329056496,1.,-1.74010053962252));
#30761=CARTESIAN_POINT('Ctrl Pts',(-1.09768999241229,1.,-1.74354119236212));
#30762=CARTESIAN_POINT('Ctrl Pts',(-1.10286118991144,1.,-1.74695004214924));
#30763=CARTESIAN_POINT('Ctrl Pts',(-1.10806728183003,1.,-1.75032866075914));
#30764=CARTESIAN_POINT('Ctrl Pts',(-1.11330807582542,1.,-1.75367772094617));
#30765=CARTESIAN_POINT('Ctrl Pts',(-1.11858293216752,1.,-1.75699720772089));
#30766=CARTESIAN_POINT('Ctrl Pts',(-1.12389096855078,1.,-1.76028671825084));
#30767=CARTESIAN_POINT('Ctrl Pts',(-1.12923123555076,1.,-1.76354571966171));
#30768=CARTESIAN_POINT('Ctrl Pts',(-1.13460291804635,1.,-1.76677384551883));
#30769=CARTESIAN_POINT('Ctrl Pts',(-1.14000548337,1.,-1.76997111386806));
#30770=CARTESIAN_POINT('Ctrl Pts',(-1.14543858226948,1.,-1.77313777896234));
#30771=CARTESIAN_POINT('Ctrl Pts',(-1.15090197841531,1.,-1.77627422557034));
#30772=CARTESIAN_POINT('Ctrl Pts',(-1.15639547194689,1.,-1.77938085564261));
#30773=CARTESIAN_POINT('Ctrl Pts',(-1.16191881298458,1.,-1.78245795880949));
#30774=CARTESIAN_POINT('Ctrl Pts',(-1.16747166312239,1.,-1.78550566040349));
#30775=CARTESIAN_POINT('Ctrl Pts',(-1.17305363177265,1.,-1.78852398877523));
#30776=CARTESIAN_POINT('Ctrl Pts',(-1.17866429440781,1.,-1.79151291552646));
#30777=CARTESIAN_POINT('Ctrl Pts',(-1.18430321697471,1.,-1.79447240321572));
#30778=CARTESIAN_POINT('Ctrl Pts',(-1.1899699793456,1.,-1.79740245923649));
#30779=CARTESIAN_POINT('Ctrl Pts',(-1.19566418930405,1.,-1.80030314370121));
#30780=CARTESIAN_POINT('Ctrl Pts',(-1.2013854893912,1.,-1.8031745483882));
#30781=CARTESIAN_POINT('Ctrl Pts',(-1.20713356605519,1.,-1.80601678480772));
#30782=CARTESIAN_POINT('Ctrl Pts',(-1.2129081570818,1.,-1.80882996916931));
#30783=CARTESIAN_POINT('Ctrl Pts',(-1.2187090610323,1.,-1.81161420806172));
#30784=CARTESIAN_POINT('Ctrl Pts',(-1.22453613304507,1.,-1.81436959209778));
#30785=CARTESIAN_POINT('Ctrl Pts',(-1.22921864890975,1.,-1.81655087183054));
#30786=CARTESIAN_POINT('Ctrl Pts',(-1.23274224526804,1.,-1.81817389920914));
#30787=CARTESIAN_POINT('Ctrl Pts',(-1.23509651170384,1.,-1.81925017193531));
#30788=CARTESIAN_POINT('Ctrl Pts',(-1.23627494547115,1.,-1.81978687191668));
#30789=CARTESIAN_POINT('',(-0.892032620296856,0.,-1.5055822144029));
#30790=CARTESIAN_POINT('Origin',(0.,0.,0.));
#30791=CARTESIAN_POINT('',(-0.693717979106305,1.,-1.60662857109684));
#30792=CARTESIAN_POINT('Origin',(0.,1.,0.));
#30793=CARTESIAN_POINT('',(-0.693717979106306,0.,-1.60662857109684));
#30794=CARTESIAN_POINT('Ctrl Pts',(-0.745574324794401,-1.,-2.0698113262342));
#30795=CARTESIAN_POINT('Ctrl Pts',(-0.745574324794401,1.,-2.0698113262342));
#30796=CARTESIAN_POINT('Ctrl Pts',(-0.745832791378367,-1.,-2.06854248895728));
#30797=CARTESIAN_POINT('Ctrl Pts',(-0.745832791378367,1.,-2.06854248895728));
#30798=CARTESIAN_POINT('Ctrl Pts',(-0.7463458715442,-1.,-2.06600523016815));
#30799=CARTESIAN_POINT('Ctrl Pts',(-0.7463458715442,1.,-2.06600523016815));
#30800=CARTESIAN_POINT('Ctrl Pts',(-0.747103932787919,-1.,-2.06220058927826));
#30801=CARTESIAN_POINT('Ctrl Pts',(-0.747103932787919,1.,-2.06220058927826));
#30802=CARTESIAN_POINT('Ctrl Pts',(-0.748091554183802,-1.,-2.05713023031006));
#30803=CARTESIAN_POINT('Ctrl Pts',(-0.748091554183802,1.,-2.05713023031006));
#30804=CARTESIAN_POINT('Ctrl Pts',(-0.749287468665046,-1.,-2.05079645592154));
#30805=CARTESIAN_POINT('Ctrl Pts',(-0.749287468665046,1.,-2.05079645592154));
#30806=CARTESIAN_POINT('Ctrl Pts',(-0.750444657875576,-1.,-2.04446689147979));
#30807=CARTESIAN_POINT('Ctrl Pts',(-0.750444657875576,1.,-2.04446689147979));
#30808=CARTESIAN_POINT('Ctrl Pts',(-0.751562963361115,-1.,-2.03814160092099));
#30809=CARTESIAN_POINT('Ctrl Pts',(-0.751562963361115,1.,-2.03814160092099));
#30810=CARTESIAN_POINT('Ctrl Pts',(-0.752642180487211,-1.,-2.03182068456221));
#30811=CARTESIAN_POINT('Ctrl Pts',(-0.752642180487211,1.,-2.03182068456221));
#30812=CARTESIAN_POINT('Ctrl Pts',(-0.753682061112768,-1.,-2.02550428623313));
#30813=CARTESIAN_POINT('Ctrl Pts',(-0.753682061112768,1.,-2.02550428623313));
#30814=CARTESIAN_POINT('Ctrl Pts',(-0.754682330722816,-1.,-2.01919259405809));
#30815=CARTESIAN_POINT('Ctrl Pts',(-0.754682330722816,1.,-2.01919259405809));
#30816=CARTESIAN_POINT('Ctrl Pts',(-0.755642704957865,-1.,-2.01288584328084));
#30817=CARTESIAN_POINT('Ctrl Pts',(-0.755642704957865,1.,-2.01288584328084));
#30818=CARTESIAN_POINT('Ctrl Pts',(-0.75656290464667,-1.,-2.0065843158773));
#30819=CARTESIAN_POINT('Ctrl Pts',(-0.75656290464667,1.,-2.0065843158773));
#30820=CARTESIAN_POINT('Ctrl Pts',(-0.757442676862724,-1.,-2.00028834739178));
#30821=CARTESIAN_POINT('Ctrl Pts',(-0.757442676862724,1.,-2.00028834739178));
#30822=CARTESIAN_POINT('Ctrl Pts',(-0.758281796766761,-1.,-1.99399831098817));
#30823=CARTESIAN_POINT('Ctrl Pts',(-0.758281796766761,1.,-1.99399831098817));
#30824=CARTESIAN_POINT('Ctrl Pts',(-0.759080037802488,-1.,-1.98771456680874));
#30825=CARTESIAN_POINT('Ctrl Pts',(-0.759080037802488,1.,-1.98771456680874));
#30826=CARTESIAN_POINT('Ctrl Pts',(-0.75983714745219,-1.,-1.98143741418172));
#30827=CARTESIAN_POINT('Ctrl Pts',(-0.75983714745219,1.,-1.98143741418172));
#30828=CARTESIAN_POINT('Ctrl Pts',(-0.760552825409757,-1.,-1.97516705321494));
#30829=CARTESIAN_POINT('Ctrl Pts',(-0.760552825409757,1.,-1.97516705321494));
#30830=CARTESIAN_POINT('Ctrl Pts',(-0.76122669048382,-1.,-1.96890351582499));
#30831=CARTESIAN_POINT('Ctrl Pts',(-0.76122669048382,1.,-1.96890351582499));
#30832=CARTESIAN_POINT('Ctrl Pts',(-0.761858300014423,-1.,-1.96264672744186));
#30833=CARTESIAN_POINT('Ctrl Pts',(-0.761858300014423,1.,-1.96264672744186));
#30834=CARTESIAN_POINT('Ctrl Pts',(-0.762447203806179,-1.,-1.95639665309869));
#30835=CARTESIAN_POINT('Ctrl Pts',(-0.762447203806179,1.,-1.95639665309869));
#30836=CARTESIAN_POINT('Ctrl Pts',(-0.762992990878769,-1.,-1.95015342590024));
#30837=CARTESIAN_POINT('Ctrl Pts',(-0.762992990878769,1.,-1.95015342590024));
#30838=CARTESIAN_POINT('Ctrl Pts',(-0.763495333538629,-1.,-1.9439174661764));
#30839=CARTESIAN_POINT('Ctrl Pts',(-0.763495333538629,1.,-1.9439174661764));
#30840=CARTESIAN_POINT('Ctrl Pts',(-0.763954049121458,-1.,-1.93768964875886));
#30841=CARTESIAN_POINT('Ctrl Pts',(-0.763954049121458,1.,-1.93768964875886));
#30842=CARTESIAN_POINT('Ctrl Pts',(-0.764369010673941,-1.,-1.93147105496382));
#30843=CARTESIAN_POINT('Ctrl Pts',(-0.764369010673941,1.,-1.93147105496382));
#30844=CARTESIAN_POINT('Ctrl Pts',(-0.764740025488211,-1.,-1.92526263537048));
#30845=CARTESIAN_POINT('Ctrl Pts',(-0.764740025488211,1.,-1.92526263537048));
#30846=CARTESIAN_POINT('Ctrl Pts',(-0.765066729667088,-1.,-1.91906491634196));
#30847=CARTESIAN_POINT('Ctrl Pts',(-0.765066729667088,1.,-1.91906491634196));
#30848=CARTESIAN_POINT('Ctrl Pts',(-0.765348465884722,-1.,-1.91287765805169));
#30849=CARTESIAN_POINT('Ctrl Pts',(-0.765348465884722,1.,-1.91287765805169));
#30850=CARTESIAN_POINT('Ctrl Pts',(-0.765584196937919,-1.,-1.90669961402356));
#30851=CARTESIAN_POINT('Ctrl Pts',(-0.765584196937919,1.,-1.90669961402356));
#30852=CARTESIAN_POINT('Ctrl Pts',(-0.765772772593386,-1.,-1.90052930393596));
#30853=CARTESIAN_POINT('Ctrl Pts',(-0.765772772593386,1.,-1.90052930393596));
#30854=CARTESIAN_POINT('Ctrl Pts',(-0.765913193856978,-1.,-1.89436577771388));
#30855=CARTESIAN_POINT('Ctrl Pts',(-0.765913193856978,1.,-1.89436577771388));
#30856=CARTESIAN_POINT('Ctrl Pts',(-0.766004837062091,-1.,-1.88820926433409));
#30857=CARTESIAN_POINT('Ctrl Pts',(-0.766004837062091,1.,-1.88820926433409));
#30858=CARTESIAN_POINT('Ctrl Pts',(-0.766047794851865,-1.,-1.88206215302561));
#30859=CARTESIAN_POINT('Ctrl Pts',(-0.766047794851865,1.,-1.88206215302561));
#30860=CARTESIAN_POINT('Ctrl Pts',(-0.766042837036744,-1.,-1.87592888967883));
#30861=CARTESIAN_POINT('Ctrl Pts',(-0.766042837036744,1.,-1.87592888967883));
#30862=CARTESIAN_POINT('Ctrl Pts',(-0.765990708546091,-1.,-1.86981398314341));
#30863=CARTESIAN_POINT('Ctrl Pts',(-0.765990708546091,1.,-1.86981398314341));
#30864=CARTESIAN_POINT('Ctrl Pts',(-0.765891519092547,-1.,-1.86372027063312));
#30865=CARTESIAN_POINT('Ctrl Pts',(-0.765891519092547,1.,-1.86372027063312));
#30866=CARTESIAN_POINT('Ctrl Pts',(-0.765744212909318,-1.,-1.85764741390394));
#30867=CARTESIAN_POINT('Ctrl Pts',(-0.765744212909318,1.,-1.85764741390394));
#30868=CARTESIAN_POINT('Ctrl Pts',(-0.765545710619062,-1.,-1.85158945130063));
#30869=CARTESIAN_POINT('Ctrl Pts',(-0.765545710619062,1.,-1.85158945130063));
#30870=CARTESIAN_POINT('Ctrl Pts',(-0.765291664862029,-1.,-1.84553698875924));
#30871=CARTESIAN_POINT('Ctrl Pts',(-0.765291664862029,1.,-1.84553698875924));
#30872=CARTESIAN_POINT('Ctrl Pts',(-0.764978057881737,-1.,-1.83948181064835));
#30873=CARTESIAN_POINT('Ctrl Pts',(-0.764978057881737,1.,-1.83948181064835));
#30874=CARTESIAN_POINT('Ctrl Pts',(-0.764602549687853,-1.,-1.83342077227142));
#30875=CARTESIAN_POINT('Ctrl Pts',(-0.764602549687853,1.,-1.83342077227142));
#30876=CARTESIAN_POINT('Ctrl Pts',(-0.764165902605995,-1.,-1.82735991200065));
#30877=CARTESIAN_POINT('Ctrl Pts',(-0.764165902605995,1.,-1.82735991200065));
#30878=CARTESIAN_POINT('Ctrl Pts',(-0.763673465462726,-1.,-1.82131873145266));
#30879=CARTESIAN_POINT('Ctrl Pts',(-0.763673465462726,1.,-1.82131873145266));
#30880=CARTESIAN_POINT('Ctrl Pts',(-0.763132003836634,-1.,-1.8153211840553));
#30881=CARTESIAN_POINT('Ctrl Pts',(-0.763132003836634,1.,-1.8153211840553));
#30882=CARTESIAN_POINT('Ctrl Pts',(-0.762546129463938,-1.,-1.80938551463965));
#30883=CARTESIAN_POINT('Ctrl Pts',(-0.762546129463938,1.,-1.80938551463965));
#30884=CARTESIAN_POINT('Ctrl Pts',(-0.761915336443547,-1.,-1.80351583877342));
#30885=CARTESIAN_POINT('Ctrl Pts',(-0.761915336443547,1.,-1.80351583877342));
#30886=CARTESIAN_POINT('Ctrl Pts',(-0.761229695230558,-1.,-1.79768986997783));
#30887=CARTESIAN_POINT('Ctrl Pts',(-0.761229695230558,1.,-1.79768986997783));
#30888=CARTESIAN_POINT('Ctrl Pts',(-0.760469555880749,-1.,-1.7918581561088));
#30889=CARTESIAN_POINT('Ctrl Pts',(-0.760469555880749,1.,-1.7918581561088));
#30890=CARTESIAN_POINT('Ctrl Pts',(-0.759614401110189,-1.,-1.78596964884604));
#30891=CARTESIAN_POINT('Ctrl Pts',(-0.759614401110189,1.,-1.78596964884604));
#30892=CARTESIAN_POINT('Ctrl Pts',(-0.758650626677518,-1.,-1.77999411220945));
#30893=CARTESIAN_POINT('Ctrl Pts',(-0.758650626677518,1.,-1.77999411220945));
#30894=CARTESIAN_POINT('Ctrl Pts',(-0.757578264077029,-1.,-1.77394167108292));
#30895=CARTESIAN_POINT('Ctrl Pts',(-0.757578264077029,1.,-1.77394167108292));
#30896=CARTESIAN_POINT('Ctrl Pts',(-0.75642189602781,-1.,-1.76789396002998));
#30897=CARTESIAN_POINT('Ctrl Pts',(-0.75642189602781,1.,-1.76789396002998));
#30898=CARTESIAN_POINT('Ctrl Pts',(-0.755220979974461,-1.,-1.76197817240128));
#30899=CARTESIAN_POINT('Ctrl Pts',(-0.755220979974461,1.,-1.76197817240128));
#30900=CARTESIAN_POINT('Ctrl Pts',(-0.754009254027829,-1.,-1.75631083600019));
#30901=CARTESIAN_POINT('Ctrl Pts',(-0.754009254027829,1.,-1.75631083600019));
#30902=CARTESIAN_POINT('Ctrl Pts',(-0.752797683531314,-1.,-1.75095139468794));
#30903=CARTESIAN_POINT('Ctrl Pts',(-0.752797683531314,1.,-1.75095139468794));
#30904=CARTESIAN_POINT('Ctrl Pts',(-0.751555614164482,-1.,-1.74585086852502));
#30905=CARTESIAN_POINT('Ctrl Pts',(-0.751555614164482,1.,-1.74585086852502));
#30906=CARTESIAN_POINT('Ctrl Pts',(-0.750193435981249,-1.,-1.74080458267114));
#30907=CARTESIAN_POINT('Ctrl Pts',(-0.750193435981249,1.,-1.74080458267114));
#30908=CARTESIAN_POINT('Ctrl Pts',(-0.74858246295687,-1.,-1.7355035168033));
#30909=CARTESIAN_POINT('Ctrl Pts',(-0.74858246295687,1.,-1.7355035168033));
#30910=CARTESIAN_POINT('Ctrl Pts',(-0.746574710097752,-1.,-1.72958533647714));
#30911=CARTESIAN_POINT('Ctrl Pts',(-0.746574710097752,1.,-1.72958533647714));
#30912=CARTESIAN_POINT('Ctrl Pts',(-0.744021445433093,-1.,-1.72268229916769));
#30913=CARTESIAN_POINT('Ctrl Pts',(-0.744021445433093,1.,-1.72268229916769));
#30914=CARTESIAN_POINT('Ctrl Pts',(-0.74079516202821,-1.,-1.71447789751001));
#30915=CARTESIAN_POINT('Ctrl Pts',(-0.74079516202821,1.,-1.71447789751001));
#30916=CARTESIAN_POINT('Ctrl Pts',(-0.736799665716932,-1.,-1.70473309004249));
#30917=CARTESIAN_POINT('Ctrl Pts',(-0.736799665716932,1.,-1.70473309004249));
#30918=CARTESIAN_POINT('Ctrl Pts',(-0.731963238685357,-1.,-1.69326921972915));
#30919=CARTESIAN_POINT('Ctrl Pts',(-0.731963238685357,1.,-1.69326921972915));
#30920=CARTESIAN_POINT('Ctrl Pts',(-0.726235967982445,-1.,-1.67996158451922));
#30921=CARTESIAN_POINT('Ctrl Pts',(-0.726235967982445,1.,-1.67996158451922));
#30922=CARTESIAN_POINT('Ctrl Pts',(-0.71958543378795,-1.,-1.66472880551777));
#30923=CARTESIAN_POINT('Ctrl Pts',(-0.71958543378795,1.,-1.66472880551777));
#30924=CARTESIAN_POINT('Ctrl Pts',(-0.711993139340447,-1.,-1.64752408828442));
#30925=CARTESIAN_POINT('Ctrl Pts',(-0.711993139340447,1.,-1.64752408828442));
#30926=CARTESIAN_POINT('Ctrl Pts',(-0.705159151977294,-1.,-1.6321654166204));
#30927=CARTESIAN_POINT('Ctrl Pts',(-0.705159151977294,1.,-1.6321654166204));
#30928=CARTESIAN_POINT('Ctrl Pts',(-0.699605146398837,-1.,-1.61974673471117));
#30929=CARTESIAN_POINT('Ctrl Pts',(-0.699605146398837,1.,-1.61974673471117));
#30930=CARTESIAN_POINT('Ctrl Pts',(-0.69571209787897,-1.,-1.61106790957619));
#30931=CARTESIAN_POINT('Ctrl Pts',(-0.69571209787897,1.,-1.61106790957619));
#30932=CARTESIAN_POINT('Ctrl Pts',(-0.693717979106305,-1.,-1.60662857109684));
#30933=CARTESIAN_POINT('Ctrl Pts',(-0.693717979106305,1.,-1.60662857109684));
#30934=CARTESIAN_POINT('',(-0.745574324794401,1.,-2.0698113262342));
#30935=CARTESIAN_POINT('Ctrl Pts',(-0.745574324794401,1.,-2.0698113262342));
#30936=CARTESIAN_POINT('Ctrl Pts',(-0.745832791378367,1.,-2.06854248895728));
#30937=CARTESIAN_POINT('Ctrl Pts',(-0.7463458715442,1.,-2.06600523016815));
#30938=CARTESIAN_POINT('Ctrl Pts',(-0.747103932787919,1.,-2.06220058927826));
#30939=CARTESIAN_POINT('Ctrl Pts',(-0.748091554183802,1.,-2.05713023031006));
#30940=CARTESIAN_POINT('Ctrl Pts',(-0.749287468665046,1.,-2.05079645592154));
#30941=CARTESIAN_POINT('Ctrl Pts',(-0.750444657875576,1.,-2.04446689147979));
#30942=CARTESIAN_POINT('Ctrl Pts',(-0.751562963361115,1.,-2.03814160092099));
#30943=CARTESIAN_POINT('Ctrl Pts',(-0.752642180487211,1.,-2.03182068456221));
#30944=CARTESIAN_POINT('Ctrl Pts',(-0.753682061112768,1.,-2.02550428623313));
#30945=CARTESIAN_POINT('Ctrl Pts',(-0.754682330722816,1.,-2.01919259405809));
#30946=CARTESIAN_POINT('Ctrl Pts',(-0.755642704957865,1.,-2.01288584328084));
#30947=CARTESIAN_POINT('Ctrl Pts',(-0.75656290464667,1.,-2.0065843158773));
#30948=CARTESIAN_POINT('Ctrl Pts',(-0.757442676862724,1.,-2.00028834739178));
#30949=CARTESIAN_POINT('Ctrl Pts',(-0.758281796766761,1.,-1.99399831098817));
#30950=CARTESIAN_POINT('Ctrl Pts',(-0.759080037802488,1.,-1.98771456680874));
#30951=CARTESIAN_POINT('Ctrl Pts',(-0.75983714745219,1.,-1.98143741418172));
#30952=CARTESIAN_POINT('Ctrl Pts',(-0.760552825409757,1.,-1.97516705321494));
#30953=CARTESIAN_POINT('Ctrl Pts',(-0.76122669048382,1.,-1.96890351582499));
#30954=CARTESIAN_POINT('Ctrl Pts',(-0.761858300014423,1.,-1.96264672744186));
#30955=CARTESIAN_POINT('Ctrl Pts',(-0.762447203806179,1.,-1.95639665309869));
#30956=CARTESIAN_POINT('Ctrl Pts',(-0.762992990878769,1.,-1.95015342590024));
#30957=CARTESIAN_POINT('Ctrl Pts',(-0.763495333538629,1.,-1.9439174661764));
#30958=CARTESIAN_POINT('Ctrl Pts',(-0.763954049121458,1.,-1.93768964875886));
#30959=CARTESIAN_POINT('Ctrl Pts',(-0.764369010673941,1.,-1.93147105496382));
#30960=CARTESIAN_POINT('Ctrl Pts',(-0.764740025488211,1.,-1.92526263537048));
#30961=CARTESIAN_POINT('Ctrl Pts',(-0.765066729667088,1.,-1.91906491634196));
#30962=CARTESIAN_POINT('Ctrl Pts',(-0.765348465884722,1.,-1.91287765805169));
#30963=CARTESIAN_POINT('Ctrl Pts',(-0.765584196937919,1.,-1.90669961402356));
#30964=CARTESIAN_POINT('Ctrl Pts',(-0.765772772593386,1.,-1.90052930393596));
#30965=CARTESIAN_POINT('Ctrl Pts',(-0.765913193856978,1.,-1.89436577771388));
#30966=CARTESIAN_POINT('Ctrl Pts',(-0.766004837062091,1.,-1.88820926433409));
#30967=CARTESIAN_POINT('Ctrl Pts',(-0.766047794851865,1.,-1.88206215302561));
#30968=CARTESIAN_POINT('Ctrl Pts',(-0.766042837036744,1.,-1.87592888967883));
#30969=CARTESIAN_POINT('Ctrl Pts',(-0.765990708546091,1.,-1.86981398314341));
#30970=CARTESIAN_POINT('Ctrl Pts',(-0.765891519092547,1.,-1.86372027063312));
#30971=CARTESIAN_POINT('Ctrl Pts',(-0.765744212909318,1.,-1.85764741390394));
#30972=CARTESIAN_POINT('Ctrl Pts',(-0.765545710619062,1.,-1.85158945130063));
#30973=CARTESIAN_POINT('Ctrl Pts',(-0.765291664862029,1.,-1.84553698875924));
#30974=CARTESIAN_POINT('Ctrl Pts',(-0.764978057881737,1.,-1.83948181064835));
#30975=CARTESIAN_POINT('Ctrl Pts',(-0.764602549687853,1.,-1.83342077227142));
#30976=CARTESIAN_POINT('Ctrl Pts',(-0.764165902605995,1.,-1.82735991200065));
#30977=CARTESIAN_POINT('Ctrl Pts',(-0.763673465462726,1.,-1.82131873145266));
#30978=CARTESIAN_POINT('Ctrl Pts',(-0.763132003836634,1.,-1.8153211840553));
#30979=CARTESIAN_POINT('Ctrl Pts',(-0.762546129463938,1.,-1.80938551463965));
#30980=CARTESIAN_POINT('Ctrl Pts',(-0.761915336443547,1.,-1.80351583877342));
#30981=CARTESIAN_POINT('Ctrl Pts',(-0.761229695230558,1.,-1.79768986997783));
#30982=CARTESIAN_POINT('Ctrl Pts',(-0.760469555880749,1.,-1.7918581561088));
#30983=CARTESIAN_POINT('Ctrl Pts',(-0.759614401110189,1.,-1.78596964884604));
#30984=CARTESIAN_POINT('Ctrl Pts',(-0.758650626677518,1.,-1.77999411220945));
#30985=CARTESIAN_POINT('Ctrl Pts',(-0.757578264077029,1.,-1.77394167108292));
#30986=CARTESIAN_POINT('Ctrl Pts',(-0.75642189602781,1.,-1.76789396002998));
#30987=CARTESIAN_POINT('Ctrl Pts',(-0.755220979974461,1.,-1.76197817240128));
#30988=CARTESIAN_POINT('Ctrl Pts',(-0.754009254027829,1.,-1.75631083600019));
#30989=CARTESIAN_POINT('Ctrl Pts',(-0.752797683531314,1.,-1.75095139468794));
#30990=CARTESIAN_POINT('Ctrl Pts',(-0.751555614164482,1.,-1.74585086852502));
#30991=CARTESIAN_POINT('Ctrl Pts',(-0.750193435981249,1.,-1.74080458267114));
#30992=CARTESIAN_POINT('Ctrl Pts',(-0.74858246295687,1.,-1.7355035168033));
#30993=CARTESIAN_POINT('Ctrl Pts',(-0.746574710097752,1.,-1.72958533647714));
#30994=CARTESIAN_POINT('Ctrl Pts',(-0.744021445433093,1.,-1.72268229916769));
#30995=CARTESIAN_POINT('Ctrl Pts',(-0.74079516202821,1.,-1.71447789751001));
#30996=CARTESIAN_POINT('Ctrl Pts',(-0.736799665716932,1.,-1.70473309004249));
#30997=CARTESIAN_POINT('Ctrl Pts',(-0.731963238685357,1.,-1.69326921972915));
#30998=CARTESIAN_POINT('Ctrl Pts',(-0.726235967982445,1.,-1.67996158451922));
#30999=CARTESIAN_POINT('Ctrl Pts',(-0.71958543378795,1.,-1.66472880551777));
#31000=CARTESIAN_POINT('Ctrl Pts',(-0.711993139340447,1.,-1.64752408828442));
#31001=CARTESIAN_POINT('Ctrl Pts',(-0.705159151977294,1.,-1.6321654166204));
#31002=CARTESIAN_POINT('Ctrl Pts',(-0.699605146398837,1.,-1.61974673471117));
#31003=CARTESIAN_POINT('Ctrl Pts',(-0.69571209787897,1.,-1.61106790957619));
#31004=CARTESIAN_POINT('Ctrl Pts',(-0.693717979106305,1.,-1.60662857109684));
#31005=CARTESIAN_POINT('',(-0.745574324794401,0.,-2.0698113262342));
#31006=CARTESIAN_POINT('Origin',(-0.61342227326009,0.,-2.11275013067528));
#31007=CARTESIAN_POINT('',(-0.61342227326009,1.,-2.11275013067528));
#31008=CARTESIAN_POINT('',(-0.745574324794401,1.,-2.0698113262342));
#31009=CARTESIAN_POINT('',(-0.61342227326009,0.,-2.11275013067528));
#31010=CARTESIAN_POINT('Ctrl Pts',(-0.383122945602004,-1.,-1.7075470150345));
#31011=CARTESIAN_POINT('Ctrl Pts',(-0.383122945602004,1.,-1.7075470150345));
#31012=CARTESIAN_POINT('Ctrl Pts',(-0.384119047315542,-1.,-1.71231062891958));
#31013=CARTESIAN_POINT('Ctrl Pts',(-0.384119047315542,1.,-1.71231062891958));
#31014=CARTESIAN_POINT('Ctrl Pts',(-0.38607079032701,-1.,-1.72162022246158));
#31015=CARTESIAN_POINT('Ctrl Pts',(-0.38607079032701,1.,-1.72162022246158));
#31016=CARTESIAN_POINT('Ctrl Pts',(-0.388877023509191,-1.,-1.7349317097561));
#31017=CARTESIAN_POINT('Ctrl Pts',(-0.388877023509191,1.,-1.7349317097561));
#31018=CARTESIAN_POINT('Ctrl Pts',(-0.392375812294307,-1.,-1.75137405313962));
#31019=CARTESIAN_POINT('Ctrl Pts',(-0.392375812294307,1.,-1.75137405313962));
#31020=CARTESIAN_POINT('Ctrl Pts',(-0.39634619612042,-1.,-1.7697556004756));
#31021=CARTESIAN_POINT('Ctrl Pts',(-0.39634619612042,1.,-1.7697556004756));
#31022=CARTESIAN_POINT('Ctrl Pts',(-0.39991940378308,-1.,-1.78598826347533));
#31023=CARTESIAN_POINT('Ctrl Pts',(-0.39991940378308,1.,-1.78598826347533));
#31024=CARTESIAN_POINT('Ctrl Pts',(-0.403107976170441,-1.,-1.80012077176221));
#31025=CARTESIAN_POINT('Ctrl Pts',(-0.403107976170441,1.,-1.80012077176221));
#31026=CARTESIAN_POINT('Ctrl Pts',(-0.405933518411838,-1.,-1.81223801813988));
#31027=CARTESIAN_POINT('Ctrl Pts',(-0.405933518411838,1.,-1.81223801813988));
#31028=CARTESIAN_POINT('Ctrl Pts',(-0.408428948108533,-1.,-1.8224702267854));
#31029=CARTESIAN_POINT('Ctrl Pts',(-0.408428948108533,1.,-1.8224702267854));
#31030=CARTESIAN_POINT('Ctrl Pts',(-0.410641256301675,-1.,-1.83100408895216));
#31031=CARTESIAN_POINT('Ctrl Pts',(-0.410641256301675,1.,-1.83100408895216));
#31032=CARTESIAN_POINT('Ctrl Pts',(-0.412633125322162,-1.,-1.83808953475839));
#31033=CARTESIAN_POINT('Ctrl Pts',(-0.412633125322162,1.,-1.83808953475839));
#31034=CARTESIAN_POINT('Ctrl Pts',(-0.41448743825434,-1.,-1.8440575707371));
#31035=CARTESIAN_POINT('Ctrl Pts',(-0.41448743825434,1.,-1.8440575707371));
#31036=CARTESIAN_POINT('Ctrl Pts',(-0.416300022038864,-1.,-1.84929312929882));
#31037=CARTESIAN_POINT('Ctrl Pts',(-0.416300022038864,1.,-1.84929312929882));
#31038=CARTESIAN_POINT('Ctrl Pts',(-0.418164129143534,-1.,-1.85417632856234));
#31039=CARTESIAN_POINT('Ctrl Pts',(-0.418164129143534,1.,-1.85417632856234));
#31040=CARTESIAN_POINT('Ctrl Pts',(-0.420157287975619,-1.,-1.85903281096686));
#31041=CARTESIAN_POINT('Ctrl Pts',(-0.420157287975619,1.,-1.85903281096686));
#31042=CARTESIAN_POINT('Ctrl Pts',(-0.422327307418275,-1.,-1.86408083334028));
#31043=CARTESIAN_POINT('Ctrl Pts',(-0.422327307418275,1.,-1.86408083334028));
#31044=CARTESIAN_POINT('Ctrl Pts',(-0.424678177291359,-1.,-1.86937803944323));
#31045=CARTESIAN_POINT('Ctrl Pts',(-0.424678177291359,1.,-1.86937803944323));
#31046=CARTESIAN_POINT('Ctrl Pts',(-0.427183828519102,-1.,-1.87486989291484));
#31047=CARTESIAN_POINT('Ctrl Pts',(-0.427183828519102,1.,-1.87486989291484));
#31048=CARTESIAN_POINT('Ctrl Pts',(-0.429803062482344,-1.,-1.88044229001832));
#31049=CARTESIAN_POINT('Ctrl Pts',(-0.429803062482344,1.,-1.88044229001832));
#31050=CARTESIAN_POINT('Ctrl Pts',(-0.432493038548748,-1.,-1.88596913666793));
#31051=CARTESIAN_POINT('Ctrl Pts',(-0.432493038548748,1.,-1.88596913666793));
#31052=CARTESIAN_POINT('Ctrl Pts',(-0.435225660963383,-1.,-1.89136993975504));
#31053=CARTESIAN_POINT('Ctrl Pts',(-0.435225660963383,1.,-1.89136993975504));
#31054=CARTESIAN_POINT('Ctrl Pts',(-0.437995003948244,-1.,-1.89663648956466));
#31055=CARTESIAN_POINT('Ctrl Pts',(-0.437995003948244,1.,-1.89663648956466));
#31056=CARTESIAN_POINT('Ctrl Pts',(-0.440807833704038,-1.,-1.90180124389086));
#31057=CARTESIAN_POINT('Ctrl Pts',(-0.440807833704038,1.,-1.90180124389086));
#31058=CARTESIAN_POINT('Ctrl Pts',(-0.443677556849151,-1.,-1.90691756144898));
#31059=CARTESIAN_POINT('Ctrl Pts',(-0.443677556849151,1.,-1.90691756144898));
#31060=CARTESIAN_POINT('Ctrl Pts',(-0.446617343485711,-1.,-1.9120369998112));
#31061=CARTESIAN_POINT('Ctrl Pts',(-0.446617343485711,1.,-1.9120369998112));
#31062=CARTESIAN_POINT('Ctrl Pts',(-0.449632260106662,-1.,-1.91718342555755));
#31063=CARTESIAN_POINT('Ctrl Pts',(-0.449632260106662,1.,-1.91718342555755));
#31064=CARTESIAN_POINT('Ctrl Pts',(-0.452719478359432,-1.,-1.92235380648502));
#31065=CARTESIAN_POINT('Ctrl Pts',(-0.452719478359432,1.,-1.92235380648502));
#31066=CARTESIAN_POINT('Ctrl Pts',(-0.455872005174371,-1.,-1.92753067150476));
#31067=CARTESIAN_POINT('Ctrl Pts',(-0.455872005174371,1.,-1.92753067150476));
#31068=CARTESIAN_POINT('Ctrl Pts',(-0.459081234547926,-1.,-1.93269066517934));
#31069=CARTESIAN_POINT('Ctrl Pts',(-0.459081234547926,1.,-1.93269066517934));
#31070=CARTESIAN_POINT('Ctrl Pts',(-0.462340031009056,-1.,-1.93781486640821));
#31071=CARTESIAN_POINT('Ctrl Pts',(-0.462340031009056,1.,-1.93781486640821));
#31072=CARTESIAN_POINT('Ctrl Pts',(-0.46564546202603,-1.,-1.9428979419619));
#31073=CARTESIAN_POINT('Ctrl Pts',(-0.46564546202603,1.,-1.9428979419619));
#31074=CARTESIAN_POINT('Ctrl Pts',(-0.468997482913135,-1.,-1.94794381136514));
#31075=CARTESIAN_POINT('Ctrl Pts',(-0.468997482913135,1.,-1.94794381136514));
#31076=CARTESIAN_POINT('Ctrl Pts',(-0.472397672264072,-1.,-1.95296148278133));
#31077=CARTESIAN_POINT('Ctrl Pts',(-0.472397672264072,1.,-1.95296148278133));
#31078=CARTESIAN_POINT('Ctrl Pts',(-0.475848034683176,-1.,-1.95796111148177));
#31079=CARTESIAN_POINT('Ctrl Pts',(-0.475848034683176,1.,-1.95796111148177));
#31080=CARTESIAN_POINT('Ctrl Pts',(-0.479349583074855,-1.,-1.96294933055943));
#31081=CARTESIAN_POINT('Ctrl Pts',(-0.479349583074855,1.,-1.96294933055943));
#31082=CARTESIAN_POINT('Ctrl Pts',(-0.482901662120691,-1.,-1.96792703422362));
#31083=CARTESIAN_POINT('Ctrl Pts',(-0.482901662120691,1.,-1.96792703422362));
#31084=CARTESIAN_POINT('Ctrl Pts',(-0.486502692907659,-1.,-1.97289186263272));
#31085=CARTESIAN_POINT('Ctrl Pts',(-0.486502692907659,1.,-1.97289186263272));
#31086=CARTESIAN_POINT('Ctrl Pts',(-0.490150627860952,-1.,-1.97783973019229));
#31087=CARTESIAN_POINT('Ctrl Pts',(-0.490150627860952,1.,-1.97783973019229));
#31088=CARTESIAN_POINT('Ctrl Pts',(-0.493843476541495,-1.,-1.98276658761821));
#31089=CARTESIAN_POINT('Ctrl Pts',(-0.493843476541495,1.,-1.98276658761821));
#31090=CARTESIAN_POINT('Ctrl Pts',(-0.497579909545574,-1.,-1.98767044752932));
#31091=CARTESIAN_POINT('Ctrl Pts',(-0.497579909545574,1.,-1.98767044752932));
#31092=CARTESIAN_POINT('Ctrl Pts',(-0.501359287727146,-1.,-1.99255149126155));
#31093=CARTESIAN_POINT('Ctrl Pts',(-0.501359287727146,1.,-1.99255149126155));
#31094=CARTESIAN_POINT('Ctrl Pts',(-0.505181361323026,-1.,-1.99741107463572));
#31095=CARTESIAN_POINT('Ctrl Pts',(-0.505181361323026,1.,-1.99741107463572));
#31096=CARTESIAN_POINT('Ctrl Pts',(-0.509046069886157,-1.,-2.00225107134734));
#31097=CARTESIAN_POINT('Ctrl Pts',(-0.509046069886157,1.,-2.00225107134734));
#31098=CARTESIAN_POINT('Ctrl Pts',(-0.512953306961792,-1.,-2.00707309946949));
#31099=CARTESIAN_POINT('Ctrl Pts',(-0.512953306961792,1.,-2.00707309946949));
#31100=CARTESIAN_POINT('Ctrl Pts',(-0.516902681728687,-1.,-2.01187773939242));
#31101=CARTESIAN_POINT('Ctrl Pts',(-0.516902681728687,1.,-2.01187773939242));
#31102=CARTESIAN_POINT('Ctrl Pts',(-0.52089359039937,-1.,-2.01666477917286));
#31103=CARTESIAN_POINT('Ctrl Pts',(-0.52089359039937,1.,-2.01666477917286));
#31104=CARTESIAN_POINT('Ctrl Pts',(-0.524925318333476,-1.,-2.02143356304698));
#31105=CARTESIAN_POINT('Ctrl Pts',(-0.524925318333476,1.,-2.02143356304698));
#31106=CARTESIAN_POINT('Ctrl Pts',(-0.528997127241914,-1.,-2.0261832908329));
#31107=CARTESIAN_POINT('Ctrl Pts',(-0.528997127241914,1.,-2.0261832908329));
#31108=CARTESIAN_POINT('Ctrl Pts',(-0.533108355132977,-1.,-2.03091336214426));
#31109=CARTESIAN_POINT('Ctrl Pts',(-0.533108355132977,1.,-2.03091336214426));
#31110=CARTESIAN_POINT('Ctrl Pts',(-0.537258489833262,-1.,-2.03562362954037));
#31111=CARTESIAN_POINT('Ctrl Pts',(-0.537258489833262,1.,-2.03562362954037));
#31112=CARTESIAN_POINT('Ctrl Pts',(-0.541447120615659,-1.,-2.04031422690527));
#31113=CARTESIAN_POINT('Ctrl Pts',(-0.541447120615659,1.,-2.04031422690527));
#31114=CARTESIAN_POINT('Ctrl Pts',(-0.54567390381743,-1.,-2.04498544714588));
#31115=CARTESIAN_POINT('Ctrl Pts',(-0.54567390381743,1.,-2.04498544714588));
#31116=CARTESIAN_POINT('Ctrl Pts',(-0.549938525150295,-1.,-2.04963761077958));
#31117=CARTESIAN_POINT('Ctrl Pts',(-0.549938525150295,1.,-2.04963761077958));
#31118=CARTESIAN_POINT('Ctrl Pts',(-0.554240657463906,-1.,-2.05427091604413));
#31119=CARTESIAN_POINT('Ctrl Pts',(-0.554240657463906,1.,-2.05427091604413));
#31120=CARTESIAN_POINT('Ctrl Pts',(-0.558579940185151,-1.,-2.05888537756462));
#31121=CARTESIAN_POINT('Ctrl Pts',(-0.558579940185151,1.,-2.05888537756462));
#31122=CARTESIAN_POINT('Ctrl Pts',(-0.562955993082261,-1.,-2.06348090160589));
#31123=CARTESIAN_POINT('Ctrl Pts',(-0.562955993082261,1.,-2.06348090160589));
#31124=CARTESIAN_POINT('Ctrl Pts',(-0.567368421181087,-1.,-2.06805732997334));
#31125=CARTESIAN_POINT('Ctrl Pts',(-0.567368421181087,1.,-2.06805732997334));
#31126=CARTESIAN_POINT('Ctrl Pts',(-0.571816823242603,-1.,-2.07261449292824));
#31127=CARTESIAN_POINT('Ctrl Pts',(-0.571816823242603,1.,-2.07261449292824));
#31128=CARTESIAN_POINT('Ctrl Pts',(-0.576300797416844,-1.,-2.07715226767559));
#31129=CARTESIAN_POINT('Ctrl Pts',(-0.576300797416844,1.,-2.07715226767559));
#31130=CARTESIAN_POINT('Ctrl Pts',(-0.580819952108063,-1.,-2.08167059018418));
#31131=CARTESIAN_POINT('Ctrl Pts',(-0.580819952108063,1.,-2.08167059018418));
#31132=CARTESIAN_POINT('Ctrl Pts',(-0.585373918991617,-1.,-2.08616943727951));
#31133=CARTESIAN_POINT('Ctrl Pts',(-0.585373918991617,1.,-2.08616943727951));
#31134=CARTESIAN_POINT('Ctrl Pts',(-0.589962365403406,-1.,-2.09064881812129));
#31135=CARTESIAN_POINT('Ctrl Pts',(-0.589962365403406,1.,-2.09064881812129));
#31136=CARTESIAN_POINT('Ctrl Pts',(-0.594585006052162,-1.,-2.0951087622027));
#31137=CARTESIAN_POINT('Ctrl Pts',(-0.594585006052162,1.,-2.0951087622027));
#31138=CARTESIAN_POINT('Ctrl Pts',(-0.599241616420533,-1.,-2.0995493086477));
#31139=CARTESIAN_POINT('Ctrl Pts',(-0.599241616420533,1.,-2.0995493086477));
#31140=CARTESIAN_POINT('Ctrl Pts',(-0.60393203073603,-1.,-2.10397049886949));
#31141=CARTESIAN_POINT('Ctrl Pts',(-0.60393203073603,1.,-2.10397049886949));
#31142=CARTESIAN_POINT('Ctrl Pts',(-0.607711315454876,-1.,-2.1074919961518));
#31143=CARTESIAN_POINT('Ctrl Pts',(-0.607711315454876,1.,-2.1074919961518));
#31144=CARTESIAN_POINT('Ctrl Pts',(-0.610560911689899,-1.,-2.11012443807238));
#31145=CARTESIAN_POINT('Ctrl Pts',(-0.610560911689899,1.,-2.11012443807238));
#31146=CARTESIAN_POINT('Ctrl Pts',(-0.6124673655618,-1.,-2.11187554259986));
#31147=CARTESIAN_POINT('Ctrl Pts',(-0.6124673655618,1.,-2.11187554259986));
#31148=CARTESIAN_POINT('Ctrl Pts',(-0.61342227326009,-1.,-2.11275013067528));
#31149=CARTESIAN_POINT('Ctrl Pts',(-0.61342227326009,1.,-2.11275013067528));
#31150=CARTESIAN_POINT('',(-0.383122945602004,1.,-1.7075470150345));
#31151=CARTESIAN_POINT('Ctrl Pts',(-0.383122945602004,1.,-1.7075470150345));
#31152=CARTESIAN_POINT('Ctrl Pts',(-0.384119047315542,1.,-1.71231062891958));
#31153=CARTESIAN_POINT('Ctrl Pts',(-0.38607079032701,1.,-1.72162022246158));
#31154=CARTESIAN_POINT('Ctrl Pts',(-0.388877023509191,1.,-1.7349317097561));
#31155=CARTESIAN_POINT('Ctrl Pts',(-0.392375812294307,1.,-1.75137405313962));
#31156=CARTESIAN_POINT('Ctrl Pts',(-0.39634619612042,1.,-1.7697556004756));
#31157=CARTESIAN_POINT('Ctrl Pts',(-0.39991940378308,1.,-1.78598826347533));
#31158=CARTESIAN_POINT('Ctrl Pts',(-0.403107976170441,1.,-1.80012077176221));
#31159=CARTESIAN_POINT('Ctrl Pts',(-0.405933518411838,1.,-1.81223801813988));
#31160=CARTESIAN_POINT('Ctrl Pts',(-0.408428948108533,1.,-1.8224702267854));
#31161=CARTESIAN_POINT('Ctrl Pts',(-0.410641256301675,1.,-1.83100408895216));
#31162=CARTESIAN_POINT('Ctrl Pts',(-0.412633125322162,1.,-1.83808953475839));
#31163=CARTESIAN_POINT('Ctrl Pts',(-0.41448743825434,1.,-1.8440575707371));
#31164=CARTESIAN_POINT('Ctrl Pts',(-0.416300022038864,1.,-1.84929312929882));
#31165=CARTESIAN_POINT('Ctrl Pts',(-0.418164129143534,1.,-1.85417632856234));
#31166=CARTESIAN_POINT('Ctrl Pts',(-0.420157287975619,1.,-1.85903281096686));
#31167=CARTESIAN_POINT('Ctrl Pts',(-0.422327307418275,1.,-1.86408083334028));
#31168=CARTESIAN_POINT('Ctrl Pts',(-0.424678177291359,1.,-1.86937803944323));
#31169=CARTESIAN_POINT('Ctrl Pts',(-0.427183828519102,1.,-1.87486989291484));
#31170=CARTESIAN_POINT('Ctrl Pts',(-0.429803062482344,1.,-1.88044229001832));
#31171=CARTESIAN_POINT('Ctrl Pts',(-0.432493038548748,1.,-1.88596913666793));
#31172=CARTESIAN_POINT('Ctrl Pts',(-0.435225660963383,1.,-1.89136993975504));
#31173=CARTESIAN_POINT('Ctrl Pts',(-0.437995003948244,1.,-1.89663648956466));
#31174=CARTESIAN_POINT('Ctrl Pts',(-0.440807833704038,1.,-1.90180124389086));
#31175=CARTESIAN_POINT('Ctrl Pts',(-0.443677556849151,1.,-1.90691756144898));
#31176=CARTESIAN_POINT('Ctrl Pts',(-0.446617343485711,1.,-1.9120369998112));
#31177=CARTESIAN_POINT('Ctrl Pts',(-0.449632260106662,1.,-1.91718342555755));
#31178=CARTESIAN_POINT('Ctrl Pts',(-0.452719478359432,1.,-1.92235380648502));
#31179=CARTESIAN_POINT('Ctrl Pts',(-0.455872005174371,1.,-1.92753067150476));
#31180=CARTESIAN_POINT('Ctrl Pts',(-0.459081234547926,1.,-1.93269066517934));
#31181=CARTESIAN_POINT('Ctrl Pts',(-0.462340031009056,1.,-1.93781486640821));
#31182=CARTESIAN_POINT('Ctrl Pts',(-0.46564546202603,1.,-1.9428979419619));
#31183=CARTESIAN_POINT('Ctrl Pts',(-0.468997482913135,1.,-1.94794381136514));
#31184=CARTESIAN_POINT('Ctrl Pts',(-0.472397672264072,1.,-1.95296148278133));
#31185=CARTESIAN_POINT('Ctrl Pts',(-0.475848034683176,1.,-1.95796111148177));
#31186=CARTESIAN_POINT('Ctrl Pts',(-0.479349583074855,1.,-1.96294933055943));
#31187=CARTESIAN_POINT('Ctrl Pts',(-0.482901662120691,1.,-1.96792703422362));
#31188=CARTESIAN_POINT('Ctrl Pts',(-0.486502692907659,1.,-1.97289186263272));
#31189=CARTESIAN_POINT('Ctrl Pts',(-0.490150627860952,1.,-1.97783973019229));
#31190=CARTESIAN_POINT('Ctrl Pts',(-0.493843476541495,1.,-1.98276658761821));
#31191=CARTESIAN_POINT('Ctrl Pts',(-0.497579909545574,1.,-1.98767044752932));
#31192=CARTESIAN_POINT('Ctrl Pts',(-0.501359287727146,1.,-1.99255149126155));
#31193=CARTESIAN_POINT('Ctrl Pts',(-0.505181361323026,1.,-1.99741107463572));
#31194=CARTESIAN_POINT('Ctrl Pts',(-0.509046069886157,1.,-2.00225107134734));
#31195=CARTESIAN_POINT('Ctrl Pts',(-0.512953306961792,1.,-2.00707309946949));
#31196=CARTESIAN_POINT('Ctrl Pts',(-0.516902681728687,1.,-2.01187773939242));
#31197=CARTESIAN_POINT('Ctrl Pts',(-0.52089359039937,1.,-2.01666477917286));
#31198=CARTESIAN_POINT('Ctrl Pts',(-0.524925318333476,1.,-2.02143356304698));
#31199=CARTESIAN_POINT('Ctrl Pts',(-0.528997127241914,1.,-2.0261832908329));
#31200=CARTESIAN_POINT('Ctrl Pts',(-0.533108355132977,1.,-2.03091336214426));
#31201=CARTESIAN_POINT('Ctrl Pts',(-0.537258489833262,1.,-2.03562362954037));
#31202=CARTESIAN_POINT('Ctrl Pts',(-0.541447120615659,1.,-2.04031422690527));
#31203=CARTESIAN_POINT('Ctrl Pts',(-0.54567390381743,1.,-2.04498544714588));
#31204=CARTESIAN_POINT('Ctrl Pts',(-0.549938525150295,1.,-2.04963761077958));
#31205=CARTESIAN_POINT('Ctrl Pts',(-0.554240657463906,1.,-2.05427091604413));
#31206=CARTESIAN_POINT('Ctrl Pts',(-0.558579940185151,1.,-2.05888537756462));
#31207=CARTESIAN_POINT('Ctrl Pts',(-0.562955993082261,1.,-2.06348090160589));
#31208=CARTESIAN_POINT('Ctrl Pts',(-0.567368421181087,1.,-2.06805732997334));
#31209=CARTESIAN_POINT('Ctrl Pts',(-0.571816823242603,1.,-2.07261449292824));
#31210=CARTESIAN_POINT('Ctrl Pts',(-0.576300797416844,1.,-2.07715226767559));
#31211=CARTESIAN_POINT('Ctrl Pts',(-0.580819952108063,1.,-2.08167059018418));
#31212=CARTESIAN_POINT('Ctrl Pts',(-0.585373918991617,1.,-2.08616943727951));
#31213=CARTESIAN_POINT('Ctrl Pts',(-0.589962365403406,1.,-2.09064881812129));
#31214=CARTESIAN_POINT('Ctrl Pts',(-0.594585006052162,1.,-2.0951087622027));
#31215=CARTESIAN_POINT('Ctrl Pts',(-0.599241616420533,1.,-2.0995493086477));
#31216=CARTESIAN_POINT('Ctrl Pts',(-0.60393203073603,1.,-2.10397049886949));
#31217=CARTESIAN_POINT('Ctrl Pts',(-0.607711315454876,1.,-2.1074919961518));
#31218=CARTESIAN_POINT('Ctrl Pts',(-0.610560911689899,1.,-2.11012443807238));
#31219=CARTESIAN_POINT('Ctrl Pts',(-0.6124673655618,1.,-2.11187554259986));
#31220=CARTESIAN_POINT('Ctrl Pts',(-0.61342227326009,1.,-2.11275013067528));
#31221=CARTESIAN_POINT('',(-0.383122945602003,0.,-1.7075470150345));
#31222=CARTESIAN_POINT('Origin',(0.,0.,0.));
#31223=CARTESIAN_POINT('',(-0.163289472382896,1.,-1.74236521665491));
#31224=CARTESIAN_POINT('Origin',(0.,1.,0.));
#31225=CARTESIAN_POINT('',(-0.163289472382896,0.,-1.74236521665491));
#31226=CARTESIAN_POINT('Ctrl Pts',(-0.0694764450219581,-1.,-2.19890268624765));
#31227=CARTESIAN_POINT('Ctrl Pts',(-0.0694764450219581,1.,-2.19890268624765));
#31228=CARTESIAN_POINT('Ctrl Pts',(-0.070114353632549,-1.,-2.19777582085423));
#31229=CARTESIAN_POINT('Ctrl Pts',(-0.070114353632549,1.,-2.19777582085423));
#31230=CARTESIAN_POINT('Ctrl Pts',(-0.0713863779526154,-1.,-2.19552129484002));
#31231=CARTESIAN_POINT('Ctrl Pts',(-0.0713863779526154,1.,-2.19552129484002));
#31232=CARTESIAN_POINT('Ctrl Pts',(-0.0732830357306725,-1.,-2.19213712013662));
#31233=CARTESIAN_POINT('Ctrl Pts',(-0.0732830357306725,1.,-2.19213712013662));
#31234=CARTESIAN_POINT('Ctrl Pts',(-0.0757891465836148,-1.,-2.1876201139953));
#31235=CARTESIAN_POINT('Ctrl Pts',(-0.0757891465836148,1.,-2.1876201139953));
#31236=CARTESIAN_POINT('Ctrl Pts',(-0.0788837727685243,-1.,-2.18196589448887));
#31237=CARTESIAN_POINT('Ctrl Pts',(-0.0788837727685243,1.,-2.18196589448887));
#31238=CARTESIAN_POINT('Ctrl Pts',(-0.0819402680872765,-1.,-2.176303712113));
#31239=CARTESIAN_POINT('Ctrl Pts',(-0.0819402680872765,1.,-2.176303712113));
#31240=CARTESIAN_POINT('Ctrl Pts',(-0.0849584620835372,-1.,-2.17063357870952));
#31241=CARTESIAN_POINT('Ctrl Pts',(-0.0849584620835372,1.,-2.17063357870952));
#31242=CARTESIAN_POINT('Ctrl Pts',(-0.0879381291386923,-1.,-2.16495552645014));
#31243=CARTESIAN_POINT('Ctrl Pts',(-0.0879381291386923,1.,-2.16495552645014));
#31244=CARTESIAN_POINT('Ctrl Pts',(-0.0908789888107265,-1.,-2.15926961544516));
#31245=CARTESIAN_POINT('Ctrl Pts',(-0.0908789888107265,1.,-2.15926961544516));
#31246=CARTESIAN_POINT('Ctrl Pts',(-0.0937807218867643,-1.,-2.1535759397817));
#31247=CARTESIAN_POINT('Ctrl Pts',(-0.0937807218867643,1.,-2.1535759397817));
#31248=CARTESIAN_POINT('Ctrl Pts',(-0.0966429852305459,-1.,-2.14787463531795));
#31249=CARTESIAN_POINT('Ctrl Pts',(-0.0966429852305459,1.,-2.14787463531795));
#31250=CARTESIAN_POINT('Ctrl Pts',(-0.0994654261990915,-1.,-2.14216588396025));
#31251=CARTESIAN_POINT('Ctrl Pts',(-0.0994654261990915,1.,-2.14216588396025));
#31252=CARTESIAN_POINT('Ctrl Pts',(-0.1022477005561,-1.,-2.13644992667165));
#31253=CARTESIAN_POINT('Ctrl Pts',(-0.1022477005561,1.,-2.13644992667165));
#31254=CARTESIAN_POINT('Ctrl Pts',(-0.104989479152739,-1.,-2.13072704887293));
#31255=CARTESIAN_POINT('Ctrl Pts',(-0.104989479152739,1.,-2.13072704887293));
#31256=CARTESIAN_POINT('Ctrl Pts',(-0.10769043523109,-1.,-2.12499752307));
#31257=CARTESIAN_POINT('Ctrl Pts',(-0.10769043523109,1.,-2.12499752307));
#31258=CARTESIAN_POINT('Ctrl Pts',(-0.110350236135025,-1.,-2.11926155590865));
#31259=CARTESIAN_POINT('Ctrl Pts',(-0.110350236135025,1.,-2.11926155590865));
#31260=CARTESIAN_POINT('Ctrl Pts',(-0.112968534419737,-1.,-2.11351924490306));
#31261=CARTESIAN_POINT('Ctrl Pts',(-0.112968534419737,1.,-2.11351924490306));
#31262=CARTESIAN_POINT('Ctrl Pts',(-0.115544957687926,-1.,-2.10777050261309));
#31263=CARTESIAN_POINT('Ctrl Pts',(-0.115544957687926,1.,-2.10777050261309));
#31264=CARTESIAN_POINT('Ctrl Pts',(-0.118079107988355,-1.,-2.102015121329));
#31265=CARTESIAN_POINT('Ctrl Pts',(-0.118079107988355,1.,-2.102015121329));
#31266=CARTESIAN_POINT('Ctrl Pts',(-0.120570567965122,-1.,-2.0962529286773));
#31267=CARTESIAN_POINT('Ctrl Pts',(-0.120570567965122,1.,-2.0962529286773));
#31268=CARTESIAN_POINT('Ctrl Pts',(-0.123018905621083,-1.,-2.09048392424825));
#31269=CARTESIAN_POINT('Ctrl Pts',(-0.123018905621083,1.,-2.09048392424825));
#31270=CARTESIAN_POINT('Ctrl Pts',(-0.125423679412061,-1.,-2.08470840653643));
#31271=CARTESIAN_POINT('Ctrl Pts',(-0.125423679412061,1.,-2.08470840653643));
#31272=CARTESIAN_POINT('Ctrl Pts',(-0.12778444527612,-1.,-2.07892715110987));
#31273=CARTESIAN_POINT('Ctrl Pts',(-0.12778444527612,1.,-2.07892715110987));
#31274=CARTESIAN_POINT('Ctrl Pts',(-0.130100748328403,-1.,-2.07314114713063));
#31275=CARTESIAN_POINT('Ctrl Pts',(-0.130100748328403,1.,-2.07314114713063));
#31276=CARTESIAN_POINT('Ctrl Pts',(-0.13237211154771,-1.,-2.06735123910326));
#31277=CARTESIAN_POINT('Ctrl Pts',(-0.13237211154771,1.,-2.06735123910326));
#31278=CARTESIAN_POINT('Ctrl Pts',(-0.134598026192106,-1.,-2.06155781517842));
#31279=CARTESIAN_POINT('Ctrl Pts',(-0.134598026192106,1.,-2.06155781517842));
#31280=CARTESIAN_POINT('Ctrl Pts',(-0.136777941218044,-1.,-2.05576044414264));
#31281=CARTESIAN_POINT('Ctrl Pts',(-0.136777941218044,1.,-2.05576044414264));
#31282=CARTESIAN_POINT('Ctrl Pts',(-0.138911255368966,-1.,-2.04995762001328));
#31283=CARTESIAN_POINT('Ctrl Pts',(-0.138911255368966,1.,-2.04995762001328));
#31284=CARTESIAN_POINT('Ctrl Pts',(-0.140997332152546,-1.,-2.04414757947916));
#31285=CARTESIAN_POINT('Ctrl Pts',(-0.140997332152546,1.,-2.04414757947916));
#31286=CARTESIAN_POINT('Ctrl Pts',(-0.143035515058209,-1.,-2.03832911025912));
#31287=CARTESIAN_POINT('Ctrl Pts',(-0.143035515058209,1.,-2.03832911025912));
#31288=CARTESIAN_POINT('Ctrl Pts',(-0.145025140186057,-1.,-2.03250223739942));
#31289=CARTESIAN_POINT('Ctrl Pts',(-0.145025140186057,1.,-2.03250223739942));
#31290=CARTESIAN_POINT('Ctrl Pts',(-0.146965557332583,-1.,-2.02666926182017));
#31291=CARTESIAN_POINT('Ctrl Pts',(-0.146965557332583,1.,-2.02666926182017));
#31292=CARTESIAN_POINT('Ctrl Pts',(-0.148856124775337,-1.,-2.02083464969894));
#31293=CARTESIAN_POINT('Ctrl Pts',(-0.148856124775337,1.,-2.02083464969894));
#31294=CARTESIAN_POINT('Ctrl Pts',(-0.150696157673078,-1.,-2.01500291940238));
#31295=CARTESIAN_POINT('Ctrl Pts',(-0.150696157673078,1.,-2.01500291940238));
#31296=CARTESIAN_POINT('Ctrl Pts',(-0.15248488362145,-1.,-2.00917680318424));
#31297=CARTESIAN_POINT('Ctrl Pts',(-0.15248488362145,1.,-2.00917680318424));
#31298=CARTESIAN_POINT('Ctrl Pts',(-0.154221403049722,-1.,-2.00335565310543));
#31299=CARTESIAN_POINT('Ctrl Pts',(-0.154221403049722,1.,-2.00335565310543));
#31300=CARTESIAN_POINT('Ctrl Pts',(-0.155904629548783,-1.,-1.99753284771497));
#31301=CARTESIAN_POINT('Ctrl Pts',(-0.155904629548783,1.,-1.99753284771497));
#31302=CARTESIAN_POINT('Ctrl Pts',(-0.157533331459227,-1.,-1.99169810931908));
#31303=CARTESIAN_POINT('Ctrl Pts',(-0.157533331459227,1.,-1.99169810931908));
#31304=CARTESIAN_POINT('Ctrl Pts',(-0.159106226437299,-1.,-1.98584238283292));
#31305=CARTESIAN_POINT('Ctrl Pts',(-0.159106226437299,1.,-1.98584238283292));
#31306=CARTESIAN_POINT('Ctrl Pts',(-0.160622060784611,-1.,-1.97996195437559));
#31307=CARTESIAN_POINT('Ctrl Pts',(-0.160622060784611,1.,-1.97996195437559));
#31308=CARTESIAN_POINT('Ctrl Pts',(-0.162079693556289,-1.,-1.97406280235188));
#31309=CARTESIAN_POINT('Ctrl Pts',(-0.162079693556289,1.,-1.97406280235188));
#31310=CARTESIAN_POINT('Ctrl Pts',(-0.163478185457734,-1.,-1.96816512677967));
#31311=CARTESIAN_POINT('Ctrl Pts',(-0.163478185457734,1.,-1.96816512677967));
#31312=CARTESIAN_POINT('Ctrl Pts',(-0.164816568920269,-1.,-1.96229379940136));
#31313=CARTESIAN_POINT('Ctrl Pts',(-0.164816568920269,1.,-1.96229379940136));
#31314=CARTESIAN_POINT('Ctrl Pts',(-0.166093592002812,-1.,-1.9564675971873));
#31315=CARTESIAN_POINT('Ctrl Pts',(-0.166093592002812,1.,-1.9564675971873));
#31316=CARTESIAN_POINT('Ctrl Pts',(-0.167307501784475,-1.,-1.95069027794294));
#31317=CARTESIAN_POINT('Ctrl Pts',(-0.167307501784475,1.,-1.95069027794294));
#31318=CARTESIAN_POINT('Ctrl Pts',(-0.168455741607556,-1.,-1.94493757756931));
#31319=CARTESIAN_POINT('Ctrl Pts',(-0.168455741607556,1.,-1.94493757756931));
#31320=CARTESIAN_POINT('Ctrl Pts',(-0.169534904817491,-1.,-1.93915639211581));
#31321=CARTESIAN_POINT('Ctrl Pts',(-0.169534904817491,1.,-1.93915639211581));
#31322=CARTESIAN_POINT('Ctrl Pts',(-0.170541253116202,-1.,-1.93329183155539));
#31323=CARTESIAN_POINT('Ctrl Pts',(-0.170541253116202,1.,-1.93329183155539));
#31324=CARTESIAN_POINT('Ctrl Pts',(-0.171471191532988,-1.,-1.92731093582036));
#31325=CARTESIAN_POINT('Ctrl Pts',(-0.171471191532988,1.,-1.92731093582036));
#31326=CARTESIAN_POINT('Ctrl Pts',(-0.172321621259514,-1.,-1.9212233439798));
#31327=CARTESIAN_POINT('Ctrl Pts',(-0.172321621259514,1.,-1.9212233439798));
#31328=CARTESIAN_POINT('Ctrl Pts',(-0.173090695383496,-1.,-1.91511429159527));
#31329=CARTESIAN_POINT('Ctrl Pts',(-0.173090695383496,1.,-1.91511429159527));
#31330=CARTESIAN_POINT('Ctrl Pts',(-0.173776635257817,-1.,-1.90911693975267));
#31331=CARTESIAN_POINT('Ctrl Pts',(-0.173776635257817,1.,-1.90911693975267));
#31332=CARTESIAN_POINT('Ctrl Pts',(-0.174375518661085,-1.,-1.90335253862834));
#31333=CARTESIAN_POINT('Ctrl Pts',(-0.174375518661085,1.,-1.90335253862834));
#31334=CARTESIAN_POINT('Ctrl Pts',(-0.174879405091263,-1.,-1.89788101117132));
#31335=CARTESIAN_POINT('Ctrl Pts',(-0.174879405091263,1.,-1.89788101117132));
#31336=CARTESIAN_POINT('Ctrl Pts',(-0.175274276190844,-1.,-1.892646301985));
#31337=CARTESIAN_POINT('Ctrl Pts',(-0.175274276190844,1.,-1.892646301985));
#31338=CARTESIAN_POINT('Ctrl Pts',(-0.175538155840648,-1.,-1.88742606273259));
#31339=CARTESIAN_POINT('Ctrl Pts',(-0.175538155840648,1.,-1.88742606273259));
#31340=CARTESIAN_POINT('Ctrl Pts',(-0.175644148889699,-1.,-1.88188663145367));
#31341=CARTESIAN_POINT('Ctrl Pts',(-0.175644148889699,1.,-1.88188663145367));
#31342=CARTESIAN_POINT('Ctrl Pts',(-0.175563480746485,-1.,-1.87563767773588));
#31343=CARTESIAN_POINT('Ctrl Pts',(-0.175563480746485,1.,-1.87563767773588));
#31344=CARTESIAN_POINT('Ctrl Pts',(-0.175268337590758,-1.,-1.86828349694799));
#31345=CARTESIAN_POINT('Ctrl Pts',(-0.175268337590758,1.,-1.86828349694799));
#31346=CARTESIAN_POINT('Ctrl Pts',(-0.17473525927603,-1.,-1.85948367088837));
#31347=CARTESIAN_POINT('Ctrl Pts',(-0.17473525927603,1.,-1.85948367088837));
#31348=CARTESIAN_POINT('Ctrl Pts',(-0.173946627587731,-1.,-1.8489811319852));
#31349=CARTESIAN_POINT('Ctrl Pts',(-0.173946627587731,1.,-1.8489811319852));
#31350=CARTESIAN_POINT('Ctrl Pts',(-0.1728894428919,-1.,-1.83658380527692));
#31351=CARTESIAN_POINT('Ctrl Pts',(-0.1728894428919,1.,-1.83658380527692));
#31352=CARTESIAN_POINT('Ctrl Pts',(-0.171554770204119,-1.,-1.82215766811545));
#31353=CARTESIAN_POINT('Ctrl Pts',(-0.171554770204119,1.,-1.82215766811545));
#31354=CARTESIAN_POINT('Ctrl Pts',(-0.169936923904608,-1.,-1.80561530629706));
#31355=CARTESIAN_POINT('Ctrl Pts',(-0.169936923904608,1.,-1.80561530629706));
#31356=CARTESIAN_POINT('Ctrl Pts',(-0.168032772805197,-1.,-1.7869064998507));
#31357=CARTESIAN_POINT('Ctrl Pts',(-0.168032772805197,1.,-1.7869064998507));
#31358=CARTESIAN_POINT('Ctrl Pts',(-0.1662793551464,-1.,-1.77018771684844));
#31359=CARTESIAN_POINT('Ctrl Pts',(-0.1662793551464,1.,-1.77018771684844));
#31360=CARTESIAN_POINT('Ctrl Pts',(-0.164834765707158,-1.,-1.75666056638427));
#31361=CARTESIAN_POINT('Ctrl Pts',(-0.164834765707158,1.,-1.75666056638427));
#31362=CARTESIAN_POINT('Ctrl Pts',(-0.163814161002002,-1.,-1.7472034950333));
#31363=CARTESIAN_POINT('Ctrl Pts',(-0.163814161002002,1.,-1.7472034950333));
#31364=CARTESIAN_POINT('Ctrl Pts',(-0.163289472382896,-1.,-1.74236521665491));
#31365=CARTESIAN_POINT('Ctrl Pts',(-0.163289472382896,1.,-1.74236521665491));
#31366=CARTESIAN_POINT('',(-0.0694764450219581,1.,-2.19890268624765));
#31367=CARTESIAN_POINT('Ctrl Pts',(-0.0694764450219581,1.,-2.19890268624765));
#31368=CARTESIAN_POINT('Ctrl Pts',(-0.070114353632549,1.,-2.19777582085423));
#31369=CARTESIAN_POINT('Ctrl Pts',(-0.0713863779526154,1.,-2.19552129484002));
#31370=CARTESIAN_POINT('Ctrl Pts',(-0.0732830357306725,1.,-2.19213712013662));
#31371=CARTESIAN_POINT('Ctrl Pts',(-0.0757891465836148,1.,-2.1876201139953));
#31372=CARTESIAN_POINT('Ctrl Pts',(-0.0788837727685243,1.,-2.18196589448887));
#31373=CARTESIAN_POINT('Ctrl Pts',(-0.0819402680872765,1.,-2.176303712113));
#31374=CARTESIAN_POINT('Ctrl Pts',(-0.0849584620835372,1.,-2.17063357870952));
#31375=CARTESIAN_POINT('Ctrl Pts',(-0.0879381291386923,1.,-2.16495552645014));
#31376=CARTESIAN_POINT('Ctrl Pts',(-0.0908789888107265,1.,-2.15926961544516));
#31377=CARTESIAN_POINT('Ctrl Pts',(-0.0937807218867643,1.,-2.1535759397817));
#31378=CARTESIAN_POINT('Ctrl Pts',(-0.0966429852305459,1.,-2.14787463531795));
#31379=CARTESIAN_POINT('Ctrl Pts',(-0.0994654261990915,1.,-2.14216588396025));
#31380=CARTESIAN_POINT('Ctrl Pts',(-0.1022477005561,1.,-2.13644992667165));
#31381=CARTESIAN_POINT('Ctrl Pts',(-0.104989479152739,1.,-2.13072704887293));
#31382=CARTESIAN_POINT('Ctrl Pts',(-0.10769043523109,1.,-2.12499752307));
#31383=CARTESIAN_POINT('Ctrl Pts',(-0.110350236135025,1.,-2.11926155590865));
#31384=CARTESIAN_POINT('Ctrl Pts',(-0.112968534419737,1.,-2.11351924490306));
#31385=CARTESIAN_POINT('Ctrl Pts',(-0.115544957687926,1.,-2.10777050261309));
#31386=CARTESIAN_POINT('Ctrl Pts',(-0.118079107988355,1.,-2.102015121329));
#31387=CARTESIAN_POINT('Ctrl Pts',(-0.120570567965122,1.,-2.0962529286773));
#31388=CARTESIAN_POINT('Ctrl Pts',(-0.123018905621083,1.,-2.09048392424825));
#31389=CARTESIAN_POINT('Ctrl Pts',(-0.125423679412061,1.,-2.08470840653643));
#31390=CARTESIAN_POINT('Ctrl Pts',(-0.12778444527612,1.,-2.07892715110987));
#31391=CARTESIAN_POINT('Ctrl Pts',(-0.130100748328403,1.,-2.07314114713063));
#31392=CARTESIAN_POINT('Ctrl Pts',(-0.13237211154771,1.,-2.06735123910326));
#31393=CARTESIAN_POINT('Ctrl Pts',(-0.134598026192106,1.,-2.06155781517842));
#31394=CARTESIAN_POINT('Ctrl Pts',(-0.136777941218044,1.,-2.05576044414264));
#31395=CARTESIAN_POINT('Ctrl Pts',(-0.138911255368966,1.,-2.04995762001328));
#31396=CARTESIAN_POINT('Ctrl Pts',(-0.140997332152546,1.,-2.04414757947916));
#31397=CARTESIAN_POINT('Ctrl Pts',(-0.143035515058209,1.,-2.03832911025912));
#31398=CARTESIAN_POINT('Ctrl Pts',(-0.145025140186057,1.,-2.03250223739942));
#31399=CARTESIAN_POINT('Ctrl Pts',(-0.146965557332583,1.,-2.02666926182017));
#31400=CARTESIAN_POINT('Ctrl Pts',(-0.148856124775337,1.,-2.02083464969894));
#31401=CARTESIAN_POINT('Ctrl Pts',(-0.150696157673078,1.,-2.01500291940238));
#31402=CARTESIAN_POINT('Ctrl Pts',(-0.15248488362145,1.,-2.00917680318424));
#31403=CARTESIAN_POINT('Ctrl Pts',(-0.154221403049722,1.,-2.00335565310543));
#31404=CARTESIAN_POINT('Ctrl Pts',(-0.155904629548783,1.,-1.99753284771497));
#31405=CARTESIAN_POINT('Ctrl Pts',(-0.157533331459227,1.,-1.99169810931908));
#31406=CARTESIAN_POINT('Ctrl Pts',(-0.159106226437299,1.,-1.98584238283292));
#31407=CARTESIAN_POINT('Ctrl Pts',(-0.160622060784611,1.,-1.97996195437559));
#31408=CARTESIAN_POINT('Ctrl Pts',(-0.162079693556289,1.,-1.97406280235188));
#31409=CARTESIAN_POINT('Ctrl Pts',(-0.163478185457734,1.,-1.96816512677967));
#31410=CARTESIAN_POINT('Ctrl Pts',(-0.164816568920269,1.,-1.96229379940136));
#31411=CARTESIAN_POINT('Ctrl Pts',(-0.166093592002812,1.,-1.9564675971873));
#31412=CARTESIAN_POINT('Ctrl Pts',(-0.167307501784475,1.,-1.95069027794294));
#31413=CARTESIAN_POINT('Ctrl Pts',(-0.168455741607556,1.,-1.94493757756931));
#31414=CARTESIAN_POINT('Ctrl Pts',(-0.169534904817491,1.,-1.93915639211581));
#31415=CARTESIAN_POINT('Ctrl Pts',(-0.170541253116202,1.,-1.93329183155539));
#31416=CARTESIAN_POINT('Ctrl Pts',(-0.171471191532988,1.,-1.92731093582036));
#31417=CARTESIAN_POINT('Ctrl Pts',(-0.172321621259514,1.,-1.9212233439798));
#31418=CARTESIAN_POINT('Ctrl Pts',(-0.173090695383496,1.,-1.91511429159527));
#31419=CARTESIAN_POINT('Ctrl Pts',(-0.173776635257817,1.,-1.90911693975267));
#31420=CARTESIAN_POINT('Ctrl Pts',(-0.174375518661085,1.,-1.90335253862834));
#31421=CARTESIAN_POINT('Ctrl Pts',(-0.174879405091263,1.,-1.89788101117132));
#31422=CARTESIAN_POINT('Ctrl Pts',(-0.175274276190844,1.,-1.892646301985));
#31423=CARTESIAN_POINT('Ctrl Pts',(-0.175538155840648,1.,-1.88742606273259));
#31424=CARTESIAN_POINT('Ctrl Pts',(-0.175644148889699,1.,-1.88188663145367));
#31425=CARTESIAN_POINT('Ctrl Pts',(-0.175563480746485,1.,-1.87563767773588));
#31426=CARTESIAN_POINT('Ctrl Pts',(-0.175268337590758,1.,-1.86828349694799));
#31427=CARTESIAN_POINT('Ctrl Pts',(-0.17473525927603,1.,-1.85948367088837));
#31428=CARTESIAN_POINT('Ctrl Pts',(-0.173946627587731,1.,-1.8489811319852));
#31429=CARTESIAN_POINT('Ctrl Pts',(-0.1728894428919,1.,-1.83658380527692));
#31430=CARTESIAN_POINT('Ctrl Pts',(-0.171554770204119,1.,-1.82215766811545));
#31431=CARTESIAN_POINT('Ctrl Pts',(-0.169936923904608,1.,-1.80561530629706));
#31432=CARTESIAN_POINT('Ctrl Pts',(-0.168032772805197,1.,-1.7869064998507));
#31433=CARTESIAN_POINT('Ctrl Pts',(-0.1662793551464,1.,-1.77018771684844));
#31434=CARTESIAN_POINT('Ctrl Pts',(-0.164834765707158,1.,-1.75666056638427));
#31435=CARTESIAN_POINT('Ctrl Pts',(-0.163814161002002,1.,-1.7472034950333));
#31436=CARTESIAN_POINT('Ctrl Pts',(-0.163289472382896,1.,-1.74236521665491));
#31437=CARTESIAN_POINT('',(-0.0694764450219581,0.,-2.19890268624765));
#31438=CARTESIAN_POINT('Origin',(0.0694764450219584,0.,-2.19890268624765));
#31439=CARTESIAN_POINT('',(0.0694764450219584,1.,-2.19890268624765));
#31440=CARTESIAN_POINT('',(-0.0694764450219581,1.,-2.19890268624765));
#31441=CARTESIAN_POINT('',(0.0694764450219584,0.,-2.19890268624765));
#31442=CARTESIAN_POINT('Ctrl Pts',(0.163289472382896,-1.,-1.74236521665491));
#31443=CARTESIAN_POINT('Ctrl Pts',(0.163289472382896,1.,-1.74236521665491));
#31444=CARTESIAN_POINT('Ctrl Pts',(0.163814161002474,-1.,-1.74720349503904));
#31445=CARTESIAN_POINT('Ctrl Pts',(0.163814161002474,1.,-1.74720349503904));
#31446=CARTESIAN_POINT('Ctrl Pts',(0.164834765708484,-1.,-1.75666056640041));
#31447=CARTESIAN_POINT('Ctrl Pts',(0.164834765708484,1.,-1.75666056640041));
#31448=CARTESIAN_POINT('Ctrl Pts',(0.166279355148738,-1.,-1.77018771687692));
#31449=CARTESIAN_POINT('Ctrl Pts',(0.166279355148738,1.,-1.77018771687692));
#31450=CARTESIAN_POINT('Ctrl Pts',(0.16803277280837,-1.,-1.78690649988931));
#31451=CARTESIAN_POINT('Ctrl Pts',(0.16803277280837,1.,-1.78690649988931));
#31452=CARTESIAN_POINT('Ctrl Pts',(0.169936923908078,-1.,-1.80561530633924));
#31453=CARTESIAN_POINT('Ctrl Pts',(0.169936923908078,1.,-1.80561530633924));
#31454=CARTESIAN_POINT('Ctrl Pts',(0.171554770207306,-1.,-1.82215766815414));
#31455=CARTESIAN_POINT('Ctrl Pts',(0.171554770207306,1.,-1.82215766815414));
#31456=CARTESIAN_POINT('Ctrl Pts',(0.17288944289442,-1.,-1.83658380530747));
#31457=CARTESIAN_POINT('Ctrl Pts',(0.17288944289442,1.,-1.83658380530747));
#31458=CARTESIAN_POINT('Ctrl Pts',(0.173946627589401,-1.,-1.84898113200543));
#31459=CARTESIAN_POINT('Ctrl Pts',(0.173946627589401,1.,-1.84898113200543));
#31460=CARTESIAN_POINT('Ctrl Pts',(0.174735259276856,-1.,-1.85948367089838));
#31461=CARTESIAN_POINT('Ctrl Pts',(0.174735259276856,1.,-1.85948367089838));
#31462=CARTESIAN_POINT('Ctrl Pts',(0.175268337590901,-1.,-1.86828349694972));
#31463=CARTESIAN_POINT('Ctrl Pts',(0.175268337590901,1.,-1.86828349694972));
#31464=CARTESIAN_POINT('Ctrl Pts',(0.175563480746205,-1.,-1.87563767773249));
#31465=CARTESIAN_POINT('Ctrl Pts',(0.175563480746205,1.,-1.87563767773249));
#31466=CARTESIAN_POINT('Ctrl Pts',(0.175644148889271,-1.,-1.88188663144846));
#31467=CARTESIAN_POINT('Ctrl Pts',(0.175644148889271,1.,-1.88188663144846));
#31468=CARTESIAN_POINT('Ctrl Pts',(0.175538155840286,-1.,-1.88742606272818));
#31469=CARTESIAN_POINT('Ctrl Pts',(0.175538155840286,1.,-1.88742606272818));
#31470=CARTESIAN_POINT('Ctrl Pts',(0.175274276190664,-1.,-1.89264630198279));
#31471=CARTESIAN_POINT('Ctrl Pts',(0.175274276190664,1.,-1.89264630198279));
#31472=CARTESIAN_POINT('Ctrl Pts',(0.174879405091277,-1.,-1.89788101117148));
#31473=CARTESIAN_POINT('Ctrl Pts',(0.174879405091277,1.,-1.89788101117148));
#31474=CARTESIAN_POINT('Ctrl Pts',(0.174375518661222,-1.,-1.90335253863003));
#31475=CARTESIAN_POINT('Ctrl Pts',(0.174375518661222,1.,-1.90335253863003));
#31476=CARTESIAN_POINT('Ctrl Pts',(0.173776635257984,-1.,-1.90911693975475));
#31477=CARTESIAN_POINT('Ctrl Pts',(0.173776635257984,1.,-1.90911693975475));
#31478=CARTESIAN_POINT('Ctrl Pts',(0.173090695383619,-1.,-1.91511429159681));
#31479=CARTESIAN_POINT('Ctrl Pts',(0.173090695383619,1.,-1.91511429159681));
#31480=CARTESIAN_POINT('Ctrl Pts',(0.172321621259557,-1.,-1.92122334398034));
#31481=CARTESIAN_POINT('Ctrl Pts',(0.172321621259557,1.,-1.92122334398034));
#31482=CARTESIAN_POINT('Ctrl Pts',(0.17147119153296,-1.,-1.92731093582));
#31483=CARTESIAN_POINT('Ctrl Pts',(0.17147119153296,1.,-1.92731093582));
#31484=CARTESIAN_POINT('Ctrl Pts',(0.170541253116136,-1.,-1.93329183155455));
#31485=CARTESIAN_POINT('Ctrl Pts',(0.170541253116136,1.,-1.93329183155455));
#31486=CARTESIAN_POINT('Ctrl Pts',(0.169534904817425,-1.,-1.93915639211497));
#31487=CARTESIAN_POINT('Ctrl Pts',(0.169534904817425,1.,-1.93915639211497));
#31488=CARTESIAN_POINT('Ctrl Pts',(0.168455741607516,-1.,-1.94493757756879));
#31489=CARTESIAN_POINT('Ctrl Pts',(0.168455741607516,1.,-1.94493757756879));
#31490=CARTESIAN_POINT('Ctrl Pts',(0.167307501784469,-1.,-1.95069027794286));
#31491=CARTESIAN_POINT('Ctrl Pts',(0.167307501784469,1.,-1.95069027794286));
#31492=CARTESIAN_POINT('Ctrl Pts',(0.166093592002833,-1.,-1.95646759718755));
#31493=CARTESIAN_POINT('Ctrl Pts',(0.166093592002833,1.,-1.95646759718755));
#31494=CARTESIAN_POINT('Ctrl Pts',(0.1648165689203,-1.,-1.96229379940174));
#31495=CARTESIAN_POINT('Ctrl Pts',(0.1648165689203,1.,-1.96229379940174));
#31496=CARTESIAN_POINT('Ctrl Pts',(0.16347818545776,-1.,-1.96816512678));
#31497=CARTESIAN_POINT('Ctrl Pts',(0.16347818545776,1.,-1.96816512678));
#31498=CARTESIAN_POINT('Ctrl Pts',(0.162079693556302,-1.,-1.97406280235204));
#31499=CARTESIAN_POINT('Ctrl Pts',(0.162079693556302,1.,-1.97406280235204));
#31500=CARTESIAN_POINT('Ctrl Pts',(0.16062206078461,-1.,-1.97996195437557));
#31501=CARTESIAN_POINT('Ctrl Pts',(0.16062206078461,1.,-1.97996195437557));
#31502=CARTESIAN_POINT('Ctrl Pts',(0.159106226437288,-1.,-1.98584238283279));
#31503=CARTESIAN_POINT('Ctrl Pts',(0.159106226437288,1.,-1.98584238283279));
#31504=CARTESIAN_POINT('Ctrl Pts',(0.157533331459215,-1.,-1.99169810931893));
#31505=CARTESIAN_POINT('Ctrl Pts',(0.157533331459215,1.,-1.99169810931893));
#31506=CARTESIAN_POINT('Ctrl Pts',(0.155904629548774,-1.,-1.99753284771487));
#31507=CARTESIAN_POINT('Ctrl Pts',(0.155904629548774,1.,-1.99753284771487));
#31508=CARTESIAN_POINT('Ctrl Pts',(0.154221403049719,-1.,-2.00335565310539));
#31509=CARTESIAN_POINT('Ctrl Pts',(0.154221403049719,1.,-2.00335565310539));
#31510=CARTESIAN_POINT('Ctrl Pts',(0.152484883621452,-1.,-2.00917680318426));
#31511=CARTESIAN_POINT('Ctrl Pts',(0.152484883621452,1.,-2.00917680318426));
#31512=CARTESIAN_POINT('Ctrl Pts',(0.150696157673084,-1.,-2.01500291940243));
#31513=CARTESIAN_POINT('Ctrl Pts',(0.150696157673084,1.,-2.01500291940243));
#31514=CARTESIAN_POINT('Ctrl Pts',(0.148856124775343,-1.,-2.02083464969897));
#31515=CARTESIAN_POINT('Ctrl Pts',(0.148856124775343,1.,-2.02083464969897));
#31516=CARTESIAN_POINT('Ctrl Pts',(0.146965557332586,-1.,-2.02666926182017));
#31517=CARTESIAN_POINT('Ctrl Pts',(0.146965557332586,1.,-2.02666926182017));
#31518=CARTESIAN_POINT('Ctrl Pts',(0.145025140186058,-1.,-2.03250223739941));
#31519=CARTESIAN_POINT('Ctrl Pts',(0.145025140186058,1.,-2.03250223739941));
#31520=CARTESIAN_POINT('Ctrl Pts',(0.143035515058208,-1.,-2.03832911025913));
#31521=CARTESIAN_POINT('Ctrl Pts',(0.143035515058208,1.,-2.03832911025913));
#31522=CARTESIAN_POINT('Ctrl Pts',(0.140997332152545,-1.,-2.04414757947919));
#31523=CARTESIAN_POINT('Ctrl Pts',(0.140997332152545,1.,-2.04414757947919));
#31524=CARTESIAN_POINT('Ctrl Pts',(0.138911255368966,-1.,-2.04995762001333));
#31525=CARTESIAN_POINT('Ctrl Pts',(0.138911255368966,1.,-2.04995762001333));
#31526=CARTESIAN_POINT('Ctrl Pts',(0.136777941218044,-1.,-2.0557604441427));
#31527=CARTESIAN_POINT('Ctrl Pts',(0.136777941218044,1.,-2.0557604441427));
#31528=CARTESIAN_POINT('Ctrl Pts',(0.134598026192107,-1.,-2.06155781517844));
#31529=CARTESIAN_POINT('Ctrl Pts',(0.134598026192107,1.,-2.06155781517844));
#31530=CARTESIAN_POINT('Ctrl Pts',(0.13237211154771,-1.,-2.06735123910319));
#31531=CARTESIAN_POINT('Ctrl Pts',(0.13237211154771,1.,-2.06735123910319));
#31532=CARTESIAN_POINT('Ctrl Pts',(0.1301007483284,-1.,-2.07314114713047));
#31533=CARTESIAN_POINT('Ctrl Pts',(0.1301007483284,1.,-2.07314114713047));
#31534=CARTESIAN_POINT('Ctrl Pts',(0.127784445276116,-1.,-2.07892715110967));
#31535=CARTESIAN_POINT('Ctrl Pts',(0.127784445276116,1.,-2.07892715110967));
#31536=CARTESIAN_POINT('Ctrl Pts',(0.125423679412058,-1.,-2.08470840653628));
#31537=CARTESIAN_POINT('Ctrl Pts',(0.125423679412058,1.,-2.08470840653628));
#31538=CARTESIAN_POINT('Ctrl Pts',(0.123018905621083,-1.,-2.09048392424826));
#31539=CARTESIAN_POINT('Ctrl Pts',(0.123018905621083,1.,-2.09048392424826));
#31540=CARTESIAN_POINT('Ctrl Pts',(0.120570567965129,-1.,-2.09625292867756));
#31541=CARTESIAN_POINT('Ctrl Pts',(0.120570567965129,1.,-2.09625292867756));
#31542=CARTESIAN_POINT('Ctrl Pts',(0.118079107988368,-1.,-2.10201512132945));
#31543=CARTESIAN_POINT('Ctrl Pts',(0.118079107988368,1.,-2.10201512132945));
#31544=CARTESIAN_POINT('Ctrl Pts',(0.11554495768794,-1.,-2.10777050261359));
#31545=CARTESIAN_POINT('Ctrl Pts',(0.11554495768794,1.,-2.10777050261359));
#31546=CARTESIAN_POINT('Ctrl Pts',(0.112968534419746,-1.,-2.11351924490335));
#31547=CARTESIAN_POINT('Ctrl Pts',(0.112968534419746,1.,-2.11351924490335));
#31548=CARTESIAN_POINT('Ctrl Pts',(0.11035023613502,-1.,-2.11926155590849));
#31549=CARTESIAN_POINT('Ctrl Pts',(0.11035023613502,1.,-2.11926155590849));
#31550=CARTESIAN_POINT('Ctrl Pts',(0.107690435231068,-1.,-2.12499752306927));
#31551=CARTESIAN_POINT('Ctrl Pts',(0.107690435231068,1.,-2.12499752306927));
#31552=CARTESIAN_POINT('Ctrl Pts',(0.104989479152703,-1.,-2.1307270488718));
#31553=CARTESIAN_POINT('Ctrl Pts',(0.104989479152703,1.,-2.1307270488718));
#31554=CARTESIAN_POINT('Ctrl Pts',(0.102247700556064,-1.,-2.13644992667052));
#31555=CARTESIAN_POINT('Ctrl Pts',(0.102247700556064,1.,-2.13644992667052));
#31556=CARTESIAN_POINT('Ctrl Pts',(0.0994654261990743,-1.,-2.14216588395974));
#31557=CARTESIAN_POINT('Ctrl Pts',(0.0994654261990743,1.,-2.14216588395974));
#31558=CARTESIAN_POINT('Ctrl Pts',(0.0966429852305689,-1.,-2.14787463531864));
#31559=CARTESIAN_POINT('Ctrl Pts',(0.0966429852305689,1.,-2.14787463531864));
#31560=CARTESIAN_POINT('Ctrl Pts',(0.0937807218868345,-1.,-2.15357593978377));
#31561=CARTESIAN_POINT('Ctrl Pts',(0.0937807218868345,1.,-2.15357593978377));
#31562=CARTESIAN_POINT('Ctrl Pts',(0.0908789888108266,-1.,-2.15926961544808));
#31563=CARTESIAN_POINT('Ctrl Pts',(0.0908789888108266,1.,-2.15926961544808));
#31564=CARTESIAN_POINT('Ctrl Pts',(0.0879381291387823,-1.,-2.16495552645275));
#31565=CARTESIAN_POINT('Ctrl Pts',(0.0879381291387823,1.,-2.16495552645275));
#31566=CARTESIAN_POINT('Ctrl Pts',(0.0849584620835643,-1.,-2.17063357871031));
#31567=CARTESIAN_POINT('Ctrl Pts',(0.0849584620835643,1.,-2.17063357871031));
#31568=CARTESIAN_POINT('Ctrl Pts',(0.0819402680871939,-1.,-2.1763037121106));
#31569=CARTESIAN_POINT('Ctrl Pts',(0.0819402680871939,1.,-2.1763037121106));
#31570=CARTESIAN_POINT('Ctrl Pts',(0.0788837727683228,-1.,-2.18196589448304));
#31571=CARTESIAN_POINT('Ctrl Pts',(0.0788837727683228,1.,-2.18196589448304));
#31572=CARTESIAN_POINT('Ctrl Pts',(0.0757891465833411,-1.,-2.1876201139874));
#31573=CARTESIAN_POINT('Ctrl Pts',(0.0757891465833411,1.,-2.1876201139874));
#31574=CARTESIAN_POINT('Ctrl Pts',(0.0732830357304276,-1.,-2.19213712012956));
#31575=CARTESIAN_POINT('Ctrl Pts',(0.0732830357304276,1.,-2.19213712012956));
#31576=CARTESIAN_POINT('Ctrl Pts',(0.0713863779524627,-1.,-2.19552129483562));
#31577=CARTESIAN_POINT('Ctrl Pts',(0.0713863779524627,1.,-2.19552129483562));
#31578=CARTESIAN_POINT('Ctrl Pts',(0.0701143536324926,-1.,-2.19777582085261));
#31579=CARTESIAN_POINT('Ctrl Pts',(0.0701143536324926,1.,-2.19777582085261));
#31580=CARTESIAN_POINT('Ctrl Pts',(0.0694764450219584,-1.,-2.19890268624765));
#31581=CARTESIAN_POINT('Ctrl Pts',(0.0694764450219584,1.,-2.19890268624765));
#31582=CARTESIAN_POINT('',(0.163289472382896,1.,-1.74236521665491));
#31583=CARTESIAN_POINT('Ctrl Pts',(0.163289472382896,1.,-1.74236521665491));
#31584=CARTESIAN_POINT('Ctrl Pts',(0.163814161002474,1.,-1.74720349503904));
#31585=CARTESIAN_POINT('Ctrl Pts',(0.164834765708484,1.,-1.75666056640041));
#31586=CARTESIAN_POINT('Ctrl Pts',(0.166279355148738,1.,-1.77018771687692));
#31587=CARTESIAN_POINT('Ctrl Pts',(0.16803277280837,1.,-1.78690649988931));
#31588=CARTESIAN_POINT('Ctrl Pts',(0.169936923908078,1.,-1.80561530633924));
#31589=CARTESIAN_POINT('Ctrl Pts',(0.171554770207306,1.,-1.82215766815414));
#31590=CARTESIAN_POINT('Ctrl Pts',(0.17288944289442,1.,-1.83658380530747));
#31591=CARTESIAN_POINT('Ctrl Pts',(0.173946627589401,1.,-1.84898113200543));
#31592=CARTESIAN_POINT('Ctrl Pts',(0.174735259276856,1.,-1.85948367089838));
#31593=CARTESIAN_POINT('Ctrl Pts',(0.175268337590901,1.,-1.86828349694972));
#31594=CARTESIAN_POINT('Ctrl Pts',(0.175563480746205,1.,-1.87563767773249));
#31595=CARTESIAN_POINT('Ctrl Pts',(0.175644148889271,1.,-1.88188663144846));
#31596=CARTESIAN_POINT('Ctrl Pts',(0.175538155840286,1.,-1.88742606272818));
#31597=CARTESIAN_POINT('Ctrl Pts',(0.175274276190664,1.,-1.89264630198279));
#31598=CARTESIAN_POINT('Ctrl Pts',(0.174879405091277,1.,-1.89788101117148));
#31599=CARTESIAN_POINT('Ctrl Pts',(0.174375518661222,1.,-1.90335253863003));
#31600=CARTESIAN_POINT('Ctrl Pts',(0.173776635257984,1.,-1.90911693975475));
#31601=CARTESIAN_POINT('Ctrl Pts',(0.173090695383619,1.,-1.91511429159681));
#31602=CARTESIAN_POINT('Ctrl Pts',(0.172321621259557,1.,-1.92122334398034));
#31603=CARTESIAN_POINT('Ctrl Pts',(0.17147119153296,1.,-1.92731093582));
#31604=CARTESIAN_POINT('Ctrl Pts',(0.170541253116136,1.,-1.93329183155455));
#31605=CARTESIAN_POINT('Ctrl Pts',(0.169534904817425,1.,-1.93915639211497));
#31606=CARTESIAN_POINT('Ctrl Pts',(0.168455741607516,1.,-1.94493757756879));
#31607=CARTESIAN_POINT('Ctrl Pts',(0.167307501784469,1.,-1.95069027794286));
#31608=CARTESIAN_POINT('Ctrl Pts',(0.166093592002833,1.,-1.95646759718755));
#31609=CARTESIAN_POINT('Ctrl Pts',(0.1648165689203,1.,-1.96229379940174));
#31610=CARTESIAN_POINT('Ctrl Pts',(0.16347818545776,1.,-1.96816512678));
#31611=CARTESIAN_POINT('Ctrl Pts',(0.162079693556302,1.,-1.97406280235204));
#31612=CARTESIAN_POINT('Ctrl Pts',(0.16062206078461,1.,-1.97996195437557));
#31613=CARTESIAN_POINT('Ctrl Pts',(0.159106226437288,1.,-1.98584238283279));
#31614=CARTESIAN_POINT('Ctrl Pts',(0.157533331459215,1.,-1.99169810931893));
#31615=CARTESIAN_POINT('Ctrl Pts',(0.155904629548774,1.,-1.99753284771487));
#31616=CARTESIAN_POINT('Ctrl Pts',(0.154221403049719,1.,-2.00335565310539));
#31617=CARTESIAN_POINT('Ctrl Pts',(0.152484883621452,1.,-2.00917680318426));
#31618=CARTESIAN_POINT('Ctrl Pts',(0.150696157673084,1.,-2.01500291940243));
#31619=CARTESIAN_POINT('Ctrl Pts',(0.148856124775343,1.,-2.02083464969897));
#31620=CARTESIAN_POINT('Ctrl Pts',(0.146965557332586,1.,-2.02666926182017));
#31621=CARTESIAN_POINT('Ctrl Pts',(0.145025140186058,1.,-2.03250223739941));
#31622=CARTESIAN_POINT('Ctrl Pts',(0.143035515058208,1.,-2.03832911025913));
#31623=CARTESIAN_POINT('Ctrl Pts',(0.140997332152545,1.,-2.04414757947919));
#31624=CARTESIAN_POINT('Ctrl Pts',(0.138911255368966,1.,-2.04995762001333));
#31625=CARTESIAN_POINT('Ctrl Pts',(0.136777941218044,1.,-2.0557604441427));
#31626=CARTESIAN_POINT('Ctrl Pts',(0.134598026192107,1.,-2.06155781517844));
#31627=CARTESIAN_POINT('Ctrl Pts',(0.13237211154771,1.,-2.06735123910319));
#31628=CARTESIAN_POINT('Ctrl Pts',(0.1301007483284,1.,-2.07314114713047));
#31629=CARTESIAN_POINT('Ctrl Pts',(0.127784445276116,1.,-2.07892715110967));
#31630=CARTESIAN_POINT('Ctrl Pts',(0.125423679412058,1.,-2.08470840653628));
#31631=CARTESIAN_POINT('Ctrl Pts',(0.123018905621083,1.,-2.09048392424826));
#31632=CARTESIAN_POINT('Ctrl Pts',(0.120570567965129,1.,-2.09625292867756));
#31633=CARTESIAN_POINT('Ctrl Pts',(0.118079107988368,1.,-2.10201512132945));
#31634=CARTESIAN_POINT('Ctrl Pts',(0.11554495768794,1.,-2.10777050261359));
#31635=CARTESIAN_POINT('Ctrl Pts',(0.112968534419746,1.,-2.11351924490335));
#31636=CARTESIAN_POINT('Ctrl Pts',(0.11035023613502,1.,-2.11926155590849));
#31637=CARTESIAN_POINT('Ctrl Pts',(0.107690435231068,1.,-2.12499752306927));
#31638=CARTESIAN_POINT('Ctrl Pts',(0.104989479152703,1.,-2.1307270488718));
#31639=CARTESIAN_POINT('Ctrl Pts',(0.102247700556064,1.,-2.13644992667052));
#31640=CARTESIAN_POINT('Ctrl Pts',(0.0994654261990743,1.,-2.14216588395974));
#31641=CARTESIAN_POINT('Ctrl Pts',(0.0966429852305689,1.,-2.14787463531864));
#31642=CARTESIAN_POINT('Ctrl Pts',(0.0937807218868345,1.,-2.15357593978377));
#31643=CARTESIAN_POINT('Ctrl Pts',(0.0908789888108266,1.,-2.15926961544808));
#31644=CARTESIAN_POINT('Ctrl Pts',(0.0879381291387823,1.,-2.16495552645275));
#31645=CARTESIAN_POINT('Ctrl Pts',(0.0849584620835643,1.,-2.17063357871031));
#31646=CARTESIAN_POINT('Ctrl Pts',(0.0819402680871939,1.,-2.1763037121106));
#31647=CARTESIAN_POINT('Ctrl Pts',(0.0788837727683228,1.,-2.18196589448304));
#31648=CARTESIAN_POINT('Ctrl Pts',(0.0757891465833411,1.,-2.1876201139874));
#31649=CARTESIAN_POINT('Ctrl Pts',(0.0732830357304276,1.,-2.19213712012956));
#31650=CARTESIAN_POINT('Ctrl Pts',(0.0713863779524627,1.,-2.19552129483562));
#31651=CARTESIAN_POINT('Ctrl Pts',(0.0701143536324926,1.,-2.19777582085261));
#31652=CARTESIAN_POINT('Ctrl Pts',(0.0694764450219584,1.,-2.19890268624765));
#31653=CARTESIAN_POINT('',(0.163289472382896,0.,-1.74236521665491));
#31654=CARTESIAN_POINT('Origin',(0.,0.,0.));
#31655=CARTESIAN_POINT('',(0.383122945602004,1.,-1.7075470150345));
#31656=CARTESIAN_POINT('Origin',(0.,1.,0.));
#31657=CARTESIAN_POINT('',(0.383122945602004,0.,-1.7075470150345));
#31658=CARTESIAN_POINT('Ctrl Pts',(0.61342227326009,-1.,-2.11275013067528));
#31659=CARTESIAN_POINT('Ctrl Pts',(0.61342227326009,1.,-2.11275013067528));
#31660=CARTESIAN_POINT('Ctrl Pts',(0.61246736556225,-1.,-2.11187554260142));
#31661=CARTESIAN_POINT('Ctrl Pts',(0.61246736556225,1.,-2.11187554260142));
#31662=CARTESIAN_POINT('Ctrl Pts',(0.610560911691113,-1.,-2.11012443807661));
#31663=CARTESIAN_POINT('Ctrl Pts',(0.610560911691113,1.,-2.11012443807661));
#31664=CARTESIAN_POINT('Ctrl Pts',(0.607711315456826,-1.,-2.10749199615859));
#31665=CARTESIAN_POINT('Ctrl Pts',(0.607711315456826,1.,-2.10749199615859));
#31666=CARTESIAN_POINT('Ctrl Pts',(0.603932030738212,-1.,-2.10397049887709));
#31667=CARTESIAN_POINT('Ctrl Pts',(0.603932030738212,1.,-2.10397049887709));
#31668=CARTESIAN_POINT('Ctrl Pts',(0.599241616422144,-1.,-2.09954930865331));
#31669=CARTESIAN_POINT('Ctrl Pts',(0.599241616422144,1.,-2.09954930865331));
#31670=CARTESIAN_POINT('Ctrl Pts',(0.594585006052823,-1.,-2.09510876220501));
#31671=CARTESIAN_POINT('Ctrl Pts',(0.594585006052823,1.,-2.09510876220501));
#31672=CARTESIAN_POINT('Ctrl Pts',(0.589962365403189,-1.,-2.09064881812053));
#31673=CARTESIAN_POINT('Ctrl Pts',(0.589962365403189,1.,-2.09064881812053));
#31674=CARTESIAN_POINT('Ctrl Pts',(0.585373918990895,-1.,-2.086169437277));
#31675=CARTESIAN_POINT('Ctrl Pts',(0.585373918990895,1.,-2.086169437277));
#31676=CARTESIAN_POINT('Ctrl Pts',(0.580819952107256,-1.,-2.08167059018138));
#31677=CARTESIAN_POINT('Ctrl Pts',(0.580819952107256,1.,-2.08167059018138));
#31678=CARTESIAN_POINT('Ctrl Pts',(0.576300797416274,-1.,-2.07715226767361));
#31679=CARTESIAN_POINT('Ctrl Pts',(0.576300797416274,1.,-2.07715226767361));
#31680=CARTESIAN_POINT('Ctrl Pts',(0.571816823242411,-1.,-2.07261449292758));
#31681=CARTESIAN_POINT('Ctrl Pts',(0.571816823242411,1.,-2.07261449292758));
#31682=CARTESIAN_POINT('Ctrl Pts',(0.567368421181229,-1.,-2.06805732997383));
#31683=CARTESIAN_POINT('Ctrl Pts',(0.567368421181229,1.,-2.06805732997383));
#31684=CARTESIAN_POINT('Ctrl Pts',(0.562955993082574,-1.,-2.06348090160697));
#31685=CARTESIAN_POINT('Ctrl Pts',(0.562955993082574,1.,-2.06348090160697));
#31686=CARTESIAN_POINT('Ctrl Pts',(0.558579940185467,-1.,-2.05888537756571));
#31687=CARTESIAN_POINT('Ctrl Pts',(0.558579940185467,1.,-2.05888537756571));
#31688=CARTESIAN_POINT('Ctrl Pts',(0.554240657464109,-1.,-2.05427091604482));
#31689=CARTESIAN_POINT('Ctrl Pts',(0.554240657464109,1.,-2.05427091604482));
#31690=CARTESIAN_POINT('Ctrl Pts',(0.549938525150342,-1.,-2.04963761077974));
#31691=CARTESIAN_POINT('Ctrl Pts',(0.549938525150342,1.,-2.04963761077974));
#31692=CARTESIAN_POINT('Ctrl Pts',(0.545673903817348,-1.,-2.0449854471456));
#31693=CARTESIAN_POINT('Ctrl Pts',(0.545673903817348,1.,-2.0449854471456));
#31694=CARTESIAN_POINT('Ctrl Pts',(0.54144712061552,-1.,-2.0403142269048));
#31695=CARTESIAN_POINT('Ctrl Pts',(0.54144712061552,1.,-2.0403142269048));
#31696=CARTESIAN_POINT('Ctrl Pts',(0.537258489833134,-1.,-2.03562362953993));
#31697=CARTESIAN_POINT('Ctrl Pts',(0.537258489833134,1.,-2.03562362953993));
#31698=CARTESIAN_POINT('Ctrl Pts',(0.533108355132905,-1.,-2.03091336214401));
#31699=CARTESIAN_POINT('Ctrl Pts',(0.533108355132905,1.,-2.03091336214401));
#31700=CARTESIAN_POINT('Ctrl Pts',(0.52899712724191,-1.,-2.02618329083289));
#31701=CARTESIAN_POINT('Ctrl Pts',(0.52899712724191,1.,-2.02618329083289));
#31702=CARTESIAN_POINT('Ctrl Pts',(0.524925318333518,-1.,-2.02143356304712));
#31703=CARTESIAN_POINT('Ctrl Pts',(0.524925318333518,1.,-2.02143356304712));
#31704=CARTESIAN_POINT('Ctrl Pts',(0.520893590399428,-1.,-2.01666477917306));
#31705=CARTESIAN_POINT('Ctrl Pts',(0.520893590399428,1.,-2.01666477917306));
#31706=CARTESIAN_POINT('Ctrl Pts',(0.516902681728733,-1.,-2.01187773939257));
#31707=CARTESIAN_POINT('Ctrl Pts',(0.516902681728733,1.,-2.01187773939257));
#31708=CARTESIAN_POINT('Ctrl Pts',(0.512953306961813,-1.,-2.00707309946955));
#31709=CARTESIAN_POINT('Ctrl Pts',(0.512953306961813,1.,-2.00707309946955));
#31710=CARTESIAN_POINT('Ctrl Pts',(0.509046069886152,-1.,-2.00225107134733));
#31711=CARTESIAN_POINT('Ctrl Pts',(0.509046069886152,1.,-2.00225107134733));
#31712=CARTESIAN_POINT('Ctrl Pts',(0.505181361323011,-1.,-1.99741107463567));
#31713=CARTESIAN_POINT('Ctrl Pts',(0.505181361323011,1.,-1.99741107463567));
#31714=CARTESIAN_POINT('Ctrl Pts',(0.501359287727129,-1.,-1.9925514912615));
#31715=CARTESIAN_POINT('Ctrl Pts',(0.501359287727129,1.,-1.9925514912615));
#31716=CARTESIAN_POINT('Ctrl Pts',(0.497579909545564,-1.,-1.98767044752929));
#31717=CARTESIAN_POINT('Ctrl Pts',(0.497579909545564,1.,-1.98767044752929));
#31718=CARTESIAN_POINT('Ctrl Pts',(0.493843476541492,-1.,-1.9827665876182));
#31719=CARTESIAN_POINT('Ctrl Pts',(0.493843476541492,1.,-1.9827665876182));
#31720=CARTESIAN_POINT('Ctrl Pts',(0.490150627860955,-1.,-1.97783973019229));
#31721=CARTESIAN_POINT('Ctrl Pts',(0.490150627860955,1.,-1.97783973019229));
#31722=CARTESIAN_POINT('Ctrl Pts',(0.486502692907661,-1.,-1.97289186263272));
#31723=CARTESIAN_POINT('Ctrl Pts',(0.486502692907661,1.,-1.97289186263272));
#31724=CARTESIAN_POINT('Ctrl Pts',(0.482901662120686,-1.,-1.96792703422358));
#31725=CARTESIAN_POINT('Ctrl Pts',(0.482901662120686,1.,-1.96792703422358));
#31726=CARTESIAN_POINT('Ctrl Pts',(0.479349583074846,-1.,-1.96294933055938));
#31727=CARTESIAN_POINT('Ctrl Pts',(0.479349583074846,1.,-1.96294933055938));
#31728=CARTESIAN_POINT('Ctrl Pts',(0.475848034683171,-1.,-1.95796111148175));
#31729=CARTESIAN_POINT('Ctrl Pts',(0.475848034683171,1.,-1.95796111148175));
#31730=CARTESIAN_POINT('Ctrl Pts',(0.472397672264079,-1.,-1.95296148278136));
#31731=CARTESIAN_POINT('Ctrl Pts',(0.472397672264079,1.,-1.95296148278136));
#31732=CARTESIAN_POINT('Ctrl Pts',(0.468997482913158,-1.,-1.94794381136524));
#31733=CARTESIAN_POINT('Ctrl Pts',(0.468997482913158,1.,-1.94794381136524));
#31734=CARTESIAN_POINT('Ctrl Pts',(0.465645462026064,-1.,-1.94289794196205));
#31735=CARTESIAN_POINT('Ctrl Pts',(0.465645462026064,1.,-1.94289794196205));
#31736=CARTESIAN_POINT('Ctrl Pts',(0.462340031009087,-1.,-1.93781486640834));
#31737=CARTESIAN_POINT('Ctrl Pts',(0.462340031009087,1.,-1.93781486640834));
#31738=CARTESIAN_POINT('Ctrl Pts',(0.459081234547931,-1.,-1.93269066517936));
#31739=CARTESIAN_POINT('Ctrl Pts',(0.459081234547931,1.,-1.93269066517936));
#31740=CARTESIAN_POINT('Ctrl Pts',(0.455872005174335,-1.,-1.92753067150461));
#31741=CARTESIAN_POINT('Ctrl Pts',(0.455872005174335,1.,-1.92753067150461));
#31742=CARTESIAN_POINT('Ctrl Pts',(0.452719478359356,-1.,-1.9223538064847));
#31743=CARTESIAN_POINT('Ctrl Pts',(0.452719478359356,1.,-1.9223538064847));
#31744=CARTESIAN_POINT('Ctrl Pts',(0.449632260106572,-1.,-1.91718342555717));
#31745=CARTESIAN_POINT('Ctrl Pts',(0.449632260106572,1.,-1.91718342555717));
#31746=CARTESIAN_POINT('Ctrl Pts',(0.446617343485651,-1.,-1.91203699981095));
#31747=CARTESIAN_POINT('Ctrl Pts',(0.446617343485651,1.,-1.91203699981095));
#31748=CARTESIAN_POINT('Ctrl Pts',(0.44367755684917,-1.,-1.90691756144906));
#31749=CARTESIAN_POINT('Ctrl Pts',(0.44367755684917,1.,-1.90691756144906));
#31750=CARTESIAN_POINT('Ctrl Pts',(0.44080783370416,-1.,-1.90180124389137));
#31751=CARTESIAN_POINT('Ctrl Pts',(0.44080783370416,1.,-1.90180124389137));
#31752=CARTESIAN_POINT('Ctrl Pts',(0.437995003948443,-1.,-1.89663648956549));
#31753=CARTESIAN_POINT('Ctrl Pts',(0.437995003948443,1.,-1.89663648956549));
#31754=CARTESIAN_POINT('Ctrl Pts',(0.43522566096358,-1.,-1.89136993975585));
#31755=CARTESIAN_POINT('Ctrl Pts',(0.43522566096358,1.,-1.89136993975585));
#31756=CARTESIAN_POINT('Ctrl Pts',(0.432493038548833,-1.,-1.88596913666828));
#31757=CARTESIAN_POINT('Ctrl Pts',(0.432493038548833,1.,-1.88596913666828));
#31758=CARTESIAN_POINT('Ctrl Pts',(0.429803062482217,-1.,-1.88044229001779));
#31759=CARTESIAN_POINT('Ctrl Pts',(0.429803062482217,1.,-1.88044229001779));
#31760=CARTESIAN_POINT('Ctrl Pts',(0.427183828518743,-1.,-1.87486989291334));
#31761=CARTESIAN_POINT('Ctrl Pts',(0.427183828518743,1.,-1.87486989291334));
#31762=CARTESIAN_POINT('Ctrl Pts',(0.424678177290876,-1.,-1.8693780394412));
#31763=CARTESIAN_POINT('Ctrl Pts',(0.424678177290876,1.,-1.8693780394412));
#31764=CARTESIAN_POINT('Ctrl Pts',(0.422327307417884,-1.,-1.86408083333863));
#31765=CARTESIAN_POINT('Ctrl Pts',(0.422327307417884,1.,-1.86408083333863));
#31766=CARTESIAN_POINT('Ctrl Pts',(0.420157287975583,-1.,-1.8590328109667));
#31767=CARTESIAN_POINT('Ctrl Pts',(0.420157287975583,1.,-1.8590328109667));
#31768=CARTESIAN_POINT('Ctrl Pts',(0.418164129144045,-1.,-1.8541763285645));
#31769=CARTESIAN_POINT('Ctrl Pts',(0.418164129144045,1.,-1.8541763285645));
#31770=CARTESIAN_POINT('Ctrl Pts',(0.416300022039885,-1.,-1.84929312930314));
#31771=CARTESIAN_POINT('Ctrl Pts',(0.416300022039885,1.,-1.84929312930314));
#31772=CARTESIAN_POINT('Ctrl Pts',(0.414487438255542,-1.,-1.84405757074218));
#31773=CARTESIAN_POINT('Ctrl Pts',(0.414487438255542,1.,-1.84405757074218));
#31774=CARTESIAN_POINT('Ctrl Pts',(0.412633125322945,-1.,-1.8380895347617));
#31775=CARTESIAN_POINT('Ctrl Pts',(0.412633125322945,1.,-1.8380895347617));
#31776=CARTESIAN_POINT('Ctrl Pts',(0.410641256301276,-1.,-1.83100408895047));
#31777=CARTESIAN_POINT('Ctrl Pts',(0.410641256301276,1.,-1.83100408895047));
#31778=CARTESIAN_POINT('Ctrl Pts',(0.408428948106227,-1.,-1.82247022677562));
#31779=CARTESIAN_POINT('Ctrl Pts',(0.408428948106227,1.,-1.82247022677562));
#31780=CARTESIAN_POINT('Ctrl Pts',(0.405933518407175,-1.,-1.81223801812013));
#31781=CARTESIAN_POINT('Ctrl Pts',(0.405933518407175,1.,-1.81223801812013));
#31782=CARTESIAN_POINT('Ctrl Pts',(0.403107976163396,-1.,-1.80012077173238));
#31783=CARTESIAN_POINT('Ctrl Pts',(0.403107976163396,1.,-1.80012077173238));
#31784=CARTESIAN_POINT('Ctrl Pts',(0.399919403774155,-1.,-1.78598826343754));
#31785=CARTESIAN_POINT('Ctrl Pts',(0.399919403774155,1.,-1.78598826343754));
#31786=CARTESIAN_POINT('Ctrl Pts',(0.396346196110688,-1.,-1.76975560043442));
#31787=CARTESIAN_POINT('Ctrl Pts',(0.396346196110688,1.,-1.76975560043442));
#31788=CARTESIAN_POINT('Ctrl Pts',(0.392375812285395,-1.,-1.75137405310193));
#31789=CARTESIAN_POINT('Ctrl Pts',(0.392375812285395,1.,-1.75137405310193));
#31790=CARTESIAN_POINT('Ctrl Pts',(0.388877023502615,-1.,-1.73493170972829));
#31791=CARTESIAN_POINT('Ctrl Pts',(0.388877023502615,1.,-1.73493170972829));
#31792=CARTESIAN_POINT('Ctrl Pts',(0.386070790323281,-1.,-1.72162022244582));
#31793=CARTESIAN_POINT('Ctrl Pts',(0.386070790323281,1.,-1.72162022244582));
#31794=CARTESIAN_POINT('Ctrl Pts',(0.384119047314215,-1.,-1.71231062891398));
#31795=CARTESIAN_POINT('Ctrl Pts',(0.384119047314215,1.,-1.71231062891398));
#31796=CARTESIAN_POINT('Ctrl Pts',(0.383122945602004,-1.,-1.7075470150345));
#31797=CARTESIAN_POINT('Ctrl Pts',(0.383122945602004,1.,-1.7075470150345));
#31798=CARTESIAN_POINT('',(0.61342227326009,1.,-2.11275013067528));
#31799=CARTESIAN_POINT('Ctrl Pts',(0.61342227326009,1.,-2.11275013067528));
#31800=CARTESIAN_POINT('Ctrl Pts',(0.61246736556225,1.,-2.11187554260142));
#31801=CARTESIAN_POINT('Ctrl Pts',(0.610560911691113,1.,-2.11012443807661));
#31802=CARTESIAN_POINT('Ctrl Pts',(0.607711315456826,1.,-2.10749199615859));
#31803=CARTESIAN_POINT('Ctrl Pts',(0.603932030738212,1.,-2.10397049887709));
#31804=CARTESIAN_POINT('Ctrl Pts',(0.599241616422144,1.,-2.09954930865331));
#31805=CARTESIAN_POINT('Ctrl Pts',(0.594585006052823,1.,-2.09510876220501));
#31806=CARTESIAN_POINT('Ctrl Pts',(0.589962365403189,1.,-2.09064881812053));
#31807=CARTESIAN_POINT('Ctrl Pts',(0.585373918990895,1.,-2.086169437277));
#31808=CARTESIAN_POINT('Ctrl Pts',(0.580819952107256,1.,-2.08167059018138));
#31809=CARTESIAN_POINT('Ctrl Pts',(0.576300797416274,1.,-2.07715226767361));
#31810=CARTESIAN_POINT('Ctrl Pts',(0.571816823242411,1.,-2.07261449292758));
#31811=CARTESIAN_POINT('Ctrl Pts',(0.567368421181229,1.,-2.06805732997383));
#31812=CARTESIAN_POINT('Ctrl Pts',(0.562955993082574,1.,-2.06348090160697));
#31813=CARTESIAN_POINT('Ctrl Pts',(0.558579940185467,1.,-2.05888537756571));
#31814=CARTESIAN_POINT('Ctrl Pts',(0.554240657464109,1.,-2.05427091604482));
#31815=CARTESIAN_POINT('Ctrl Pts',(0.549938525150342,1.,-2.04963761077974));
#31816=CARTESIAN_POINT('Ctrl Pts',(0.545673903817348,1.,-2.0449854471456));
#31817=CARTESIAN_POINT('Ctrl Pts',(0.54144712061552,1.,-2.0403142269048));
#31818=CARTESIAN_POINT('Ctrl Pts',(0.537258489833134,1.,-2.03562362953993));
#31819=CARTESIAN_POINT('Ctrl Pts',(0.533108355132905,1.,-2.03091336214401));
#31820=CARTESIAN_POINT('Ctrl Pts',(0.52899712724191,1.,-2.02618329083289));
#31821=CARTESIAN_POINT('Ctrl Pts',(0.524925318333518,1.,-2.02143356304712));
#31822=CARTESIAN_POINT('Ctrl Pts',(0.520893590399428,1.,-2.01666477917306));
#31823=CARTESIAN_POINT('Ctrl Pts',(0.516902681728733,1.,-2.01187773939257));
#31824=CARTESIAN_POINT('Ctrl Pts',(0.512953306961813,1.,-2.00707309946955));
#31825=CARTESIAN_POINT('Ctrl Pts',(0.509046069886152,1.,-2.00225107134733));
#31826=CARTESIAN_POINT('Ctrl Pts',(0.505181361323011,1.,-1.99741107463567));
#31827=CARTESIAN_POINT('Ctrl Pts',(0.501359287727129,1.,-1.9925514912615));
#31828=CARTESIAN_POINT('Ctrl Pts',(0.497579909545564,1.,-1.98767044752929));
#31829=CARTESIAN_POINT('Ctrl Pts',(0.493843476541492,1.,-1.9827665876182));
#31830=CARTESIAN_POINT('Ctrl Pts',(0.490150627860955,1.,-1.97783973019229));
#31831=CARTESIAN_POINT('Ctrl Pts',(0.486502692907661,1.,-1.97289186263272));
#31832=CARTESIAN_POINT('Ctrl Pts',(0.482901662120686,1.,-1.96792703422358));
#31833=CARTESIAN_POINT('Ctrl Pts',(0.479349583074846,1.,-1.96294933055938));
#31834=CARTESIAN_POINT('Ctrl Pts',(0.475848034683171,1.,-1.95796111148175));
#31835=CARTESIAN_POINT('Ctrl Pts',(0.472397672264079,1.,-1.95296148278136));
#31836=CARTESIAN_POINT('Ctrl Pts',(0.468997482913158,1.,-1.94794381136524));
#31837=CARTESIAN_POINT('Ctrl Pts',(0.465645462026064,1.,-1.94289794196205));
#31838=CARTESIAN_POINT('Ctrl Pts',(0.462340031009087,1.,-1.93781486640834));
#31839=CARTESIAN_POINT('Ctrl Pts',(0.459081234547931,1.,-1.93269066517936));
#31840=CARTESIAN_POINT('Ctrl Pts',(0.455872005174335,1.,-1.92753067150461));
#31841=CARTESIAN_POINT('Ctrl Pts',(0.452719478359356,1.,-1.9223538064847));
#31842=CARTESIAN_POINT('Ctrl Pts',(0.449632260106572,1.,-1.91718342555717));
#31843=CARTESIAN_POINT('Ctrl Pts',(0.446617343485651,1.,-1.91203699981095));
#31844=CARTESIAN_POINT('Ctrl Pts',(0.44367755684917,1.,-1.90691756144906));
#31845=CARTESIAN_POINT('Ctrl Pts',(0.44080783370416,1.,-1.90180124389137));
#31846=CARTESIAN_POINT('Ctrl Pts',(0.437995003948443,1.,-1.89663648956549));
#31847=CARTESIAN_POINT('Ctrl Pts',(0.43522566096358,1.,-1.89136993975585));
#31848=CARTESIAN_POINT('Ctrl Pts',(0.432493038548833,1.,-1.88596913666828));
#31849=CARTESIAN_POINT('Ctrl Pts',(0.429803062482217,1.,-1.88044229001779));
#31850=CARTESIAN_POINT('Ctrl Pts',(0.427183828518743,1.,-1.87486989291334));
#31851=CARTESIAN_POINT('Ctrl Pts',(0.424678177290876,1.,-1.8693780394412));
#31852=CARTESIAN_POINT('Ctrl Pts',(0.422327307417884,1.,-1.86408083333863));
#31853=CARTESIAN_POINT('Ctrl Pts',(0.420157287975583,1.,-1.8590328109667));
#31854=CARTESIAN_POINT('Ctrl Pts',(0.418164129144045,1.,-1.8541763285645));
#31855=CARTESIAN_POINT('Ctrl Pts',(0.416300022039885,1.,-1.84929312930314));
#31856=CARTESIAN_POINT('Ctrl Pts',(0.414487438255542,1.,-1.84405757074218));
#31857=CARTESIAN_POINT('Ctrl Pts',(0.412633125322945,1.,-1.8380895347617));
#31858=CARTESIAN_POINT('Ctrl Pts',(0.410641256301276,1.,-1.83100408895047));
#31859=CARTESIAN_POINT('Ctrl Pts',(0.408428948106227,1.,-1.82247022677562));
#31860=CARTESIAN_POINT('Ctrl Pts',(0.405933518407175,1.,-1.81223801812013));
#31861=CARTESIAN_POINT('Ctrl Pts',(0.403107976163396,1.,-1.80012077173238));
#31862=CARTESIAN_POINT('Ctrl Pts',(0.399919403774155,1.,-1.78598826343754));
#31863=CARTESIAN_POINT('Ctrl Pts',(0.396346196110688,1.,-1.76975560043442));
#31864=CARTESIAN_POINT('Ctrl Pts',(0.392375812285395,1.,-1.75137405310193));
#31865=CARTESIAN_POINT('Ctrl Pts',(0.388877023502615,1.,-1.73493170972829));
#31866=CARTESIAN_POINT('Ctrl Pts',(0.386070790323281,1.,-1.72162022244582));
#31867=CARTESIAN_POINT('Ctrl Pts',(0.384119047314215,1.,-1.71231062891398));
#31868=CARTESIAN_POINT('Ctrl Pts',(0.383122945602004,1.,-1.7075470150345));
#31869=CARTESIAN_POINT('',(0.61342227326009,0.,-2.11275013067528));
#31870=CARTESIAN_POINT('Origin',(0.745574324794401,0.,-2.0698113262342));
#31871=CARTESIAN_POINT('',(0.745574324794401,1.,-2.0698113262342));
#31872=CARTESIAN_POINT('',(0.61342227326009,1.,-2.11275013067528));
#31873=CARTESIAN_POINT('',(0.745574324794401,0.,-2.0698113262342));
#31874=CARTESIAN_POINT('Ctrl Pts',(0.693717979106306,-1.,-1.60662857109684));
#31875=CARTESIAN_POINT('Ctrl Pts',(0.693717979106306,1.,-1.60662857109684));
#31876=CARTESIAN_POINT('Ctrl Pts',(0.695712097881194,-1.,-1.61106790958151));
#31877=CARTESIAN_POINT('Ctrl Pts',(0.695712097881194,1.,-1.61106790958151));
#31878=CARTESIAN_POINT('Ctrl Pts',(0.699605146405088,-1.,-1.61974673472612));
#31879=CARTESIAN_POINT('Ctrl Pts',(0.699605146405088,1.,-1.61974673472612));
#31880=CARTESIAN_POINT('Ctrl Pts',(0.705159151988319,-1.,-1.63216541664676));
#31881=CARTESIAN_POINT('Ctrl Pts',(0.705159151988319,1.,-1.63216541664676));
#31882=CARTESIAN_POINT('Ctrl Pts',(0.711993139355394,-1.,-1.64752408832016));
#31883=CARTESIAN_POINT('Ctrl Pts',(0.711993139355394,1.,-1.64752408832016));
#31884=CARTESIAN_POINT('Ctrl Pts',(0.719585433804282,-1.,-1.6647288055568));
#31885=CARTESIAN_POINT('Ctrl Pts',(0.719585433804282,1.,-1.6647288055568));
#31886=CARTESIAN_POINT('Ctrl Pts',(0.726235967997433,-1.,-1.67996158455503));
#31887=CARTESIAN_POINT('Ctrl Pts',(0.726235967997433,1.,-1.67996158455503));
#31888=CARTESIAN_POINT('Ctrl Pts',(0.731963238697195,-1.,-1.69326921975743));
#31889=CARTESIAN_POINT('Ctrl Pts',(0.731963238697195,1.,-1.69326921975743));
#31890=CARTESIAN_POINT('Ctrl Pts',(0.736799665724771,-1.,-1.70473309006121));
#31891=CARTESIAN_POINT('Ctrl Pts',(0.736799665724771,1.,-1.70473309006121));
#31892=CARTESIAN_POINT('Ctrl Pts',(0.740795162032087,-1.,-1.71447789751927));
#31893=CARTESIAN_POINT('Ctrl Pts',(0.740795162032087,1.,-1.71447789751927));
#31894=CARTESIAN_POINT('Ctrl Pts',(0.744021445433764,-1.,-1.7226822991693));
#31895=CARTESIAN_POINT('Ctrl Pts',(0.744021445433764,1.,-1.7226822991693));
#31896=CARTESIAN_POINT('Ctrl Pts',(0.746574710096436,-1.,-1.72958533647399));
#31897=CARTESIAN_POINT('Ctrl Pts',(0.746574710096436,1.,-1.72958533647399));
#31898=CARTESIAN_POINT('Ctrl Pts',(0.748582462954854,-1.,-1.73550351679848));
#31899=CARTESIAN_POINT('Ctrl Pts',(0.748582462954854,1.,-1.73550351679848));
#31900=CARTESIAN_POINT('Ctrl Pts',(0.75019343597954,-1.,-1.74080458266705));
#31901=CARTESIAN_POINT('Ctrl Pts',(0.75019343597954,1.,-1.74080458266705));
#31902=CARTESIAN_POINT('Ctrl Pts',(0.751555614163629,-1.,-1.74585086852298));
#31903=CARTESIAN_POINT('Ctrl Pts',(0.751555614163629,1.,-1.74585086852298));
#31904=CARTESIAN_POINT('Ctrl Pts',(0.752797683531377,-1.,-1.75095139468809));
#31905=CARTESIAN_POINT('Ctrl Pts',(0.752797683531377,1.,-1.75095139468809));
#31906=CARTESIAN_POINT('Ctrl Pts',(0.75400925402848,-1.,-1.75631083600175));
#31907=CARTESIAN_POINT('Ctrl Pts',(0.75400925402848,1.,-1.75631083600175));
#31908=CARTESIAN_POINT('Ctrl Pts',(0.755220979975262,-1.,-1.7619781724032));
#31909=CARTESIAN_POINT('Ctrl Pts',(0.755220979975262,1.,-1.7619781724032));
#31910=CARTESIAN_POINT('Ctrl Pts',(0.756421896028403,-1.,-1.76789396003141));
#31911=CARTESIAN_POINT('Ctrl Pts',(0.756421896028403,1.,-1.76789396003141));
#31912=CARTESIAN_POINT('Ctrl Pts',(0.757578264077238,-1.,-1.77394167108342));
#31913=CARTESIAN_POINT('Ctrl Pts',(0.757578264077238,1.,-1.77394167108342));
#31914=CARTESIAN_POINT('Ctrl Pts',(0.75865062667738,-1.,-1.77999411220912));
#31915=CARTESIAN_POINT('Ctrl Pts',(0.75865062667738,1.,-1.77999411220912));
#31916=CARTESIAN_POINT('Ctrl Pts',(0.759614401109868,-1.,-1.78596964884527));
#31917=CARTESIAN_POINT('Ctrl Pts',(0.759614401109868,1.,-1.78596964884527));
#31918=CARTESIAN_POINT('Ctrl Pts',(0.760469555880425,-1.,-1.79185815610802));
#31919=CARTESIAN_POINT('Ctrl Pts',(0.760469555880425,1.,-1.79185815610802));
#31920=CARTESIAN_POINT('Ctrl Pts',(0.761229695230359,-1.,-1.79768986997735));
#31921=CARTESIAN_POINT('Ctrl Pts',(0.761229695230359,1.,-1.79768986997735));
#31922=CARTESIAN_POINT('Ctrl Pts',(0.761915336443515,-1.,-1.80351583877334));
#31923=CARTESIAN_POINT('Ctrl Pts',(0.761915336443515,1.,-1.80351583877334));
#31924=CARTESIAN_POINT('Ctrl Pts',(0.762546129464036,-1.,-1.80938551463989));
#31925=CARTESIAN_POINT('Ctrl Pts',(0.762546129464036,1.,-1.80938551463989));
#31926=CARTESIAN_POINT('Ctrl Pts',(0.763132003836783,-1.,-1.81532118405566));
#31927=CARTESIAN_POINT('Ctrl Pts',(0.763132003836783,1.,-1.81532118405566));
#31928=CARTESIAN_POINT('Ctrl Pts',(0.763673465462854,-1.,-1.82131873145297));
#31929=CARTESIAN_POINT('Ctrl Pts',(0.763673465462854,1.,-1.82131873145297));
#31930=CARTESIAN_POINT('Ctrl Pts',(0.764165902606055,-1.,-1.8273599120008));
#31931=CARTESIAN_POINT('Ctrl Pts',(0.764165902606055,1.,-1.8273599120008));
#31932=CARTESIAN_POINT('Ctrl Pts',(0.764602549687845,-1.,-1.8334207722714));
#31933=CARTESIAN_POINT('Ctrl Pts',(0.764602549687845,1.,-1.8334207722714));
#31934=CARTESIAN_POINT('Ctrl Pts',(0.764978057881687,-1.,-1.83948181064823));
#31935=CARTESIAN_POINT('Ctrl Pts',(0.764978057881687,1.,-1.83948181064823));
#31936=CARTESIAN_POINT('Ctrl Pts',(0.765291664861971,-1.,-1.84553698875911));
#31937=CARTESIAN_POINT('Ctrl Pts',(0.765291664861971,1.,-1.84553698875911));
#31938=CARTESIAN_POINT('Ctrl Pts',(0.765545710619023,-1.,-1.85158945130054));
#31939=CARTESIAN_POINT('Ctrl Pts',(0.765545710619023,1.,-1.85158945130054));
#31940=CARTESIAN_POINT('Ctrl Pts',(0.765744212909305,-1.,-1.85764741390391));
#31941=CARTESIAN_POINT('Ctrl Pts',(0.765744212909305,1.,-1.85764741390391));
#31942=CARTESIAN_POINT('Ctrl Pts',(0.765891519092557,-1.,-1.86372027063315));
#31943=CARTESIAN_POINT('Ctrl Pts',(0.765891519092557,1.,-1.86372027063315));
#31944=CARTESIAN_POINT('Ctrl Pts',(0.765990708546111,-1.,-1.86981398314345));
#31945=CARTESIAN_POINT('Ctrl Pts',(0.765990708546111,1.,-1.86981398314345));
#31946=CARTESIAN_POINT('Ctrl Pts',(0.766042837036759,-1.,-1.87592888967886));
#31947=CARTESIAN_POINT('Ctrl Pts',(0.766042837036759,1.,-1.87592888967886));
#31948=CARTESIAN_POINT('Ctrl Pts',(0.766047794851868,-1.,-1.88206215302561));
#31949=CARTESIAN_POINT('Ctrl Pts',(0.766047794851868,1.,-1.88206215302561));
#31950=CARTESIAN_POINT('Ctrl Pts',(0.76600483706209,-1.,-1.88820926433409));
#31951=CARTESIAN_POINT('Ctrl Pts',(0.76600483706209,1.,-1.88820926433409));
#31952=CARTESIAN_POINT('Ctrl Pts',(0.765913193856979,-1.,-1.89436577771389));
#31953=CARTESIAN_POINT('Ctrl Pts',(0.765913193856979,1.,-1.89436577771389));
#31954=CARTESIAN_POINT('Ctrl Pts',(0.765772772593395,-1.,-1.90052930393599));
#31955=CARTESIAN_POINT('Ctrl Pts',(0.765772772593395,1.,-1.90052930393599));
#31956=CARTESIAN_POINT('Ctrl Pts',(0.765584196937936,-1.,-1.90669961402362));
#31957=CARTESIAN_POINT('Ctrl Pts',(0.765584196937936,1.,-1.90669961402362));
#31958=CARTESIAN_POINT('Ctrl Pts',(0.765348465884739,-1.,-1.91287765805174));
#31959=CARTESIAN_POINT('Ctrl Pts',(0.765348465884739,1.,-1.91287765805174));
#31960=CARTESIAN_POINT('Ctrl Pts',(0.765066729667095,-1.,-1.91906491634197));
#31961=CARTESIAN_POINT('Ctrl Pts',(0.765066729667095,1.,-1.91906491634197));
#31962=CARTESIAN_POINT('Ctrl Pts',(0.764740025488189,-1.,-1.92526263537041));
#31963=CARTESIAN_POINT('Ctrl Pts',(0.764740025488189,1.,-1.92526263537041));
#31964=CARTESIAN_POINT('Ctrl Pts',(0.764369010673889,-1.,-1.93147105496367));
#31965=CARTESIAN_POINT('Ctrl Pts',(0.764369010673889,1.,-1.93147105496367));
#31966=CARTESIAN_POINT('Ctrl Pts',(0.763954049121393,-1.,-1.93768964875867));
#31967=CARTESIAN_POINT('Ctrl Pts',(0.763954049121393,1.,-1.93768964875867));
#31968=CARTESIAN_POINT('Ctrl Pts',(0.76349533353858,-1.,-1.94391746617626));
#31969=CARTESIAN_POINT('Ctrl Pts',(0.76349533353858,1.,-1.94391746617626));
#31970=CARTESIAN_POINT('Ctrl Pts',(0.762992990878774,-1.,-1.95015342590025));
#31971=CARTESIAN_POINT('Ctrl Pts',(0.762992990878774,1.,-1.95015342590025));
#31972=CARTESIAN_POINT('Ctrl Pts',(0.762447203806263,-1.,-1.95639665309893));
#31973=CARTESIAN_POINT('Ctrl Pts',(0.762447203806263,1.,-1.95639665309893));
#31974=CARTESIAN_POINT('Ctrl Pts',(0.761858300014575,-1.,-1.96264672744229));
#31975=CARTESIAN_POINT('Ctrl Pts',(0.761858300014575,1.,-1.96264672744229));
#31976=CARTESIAN_POINT('Ctrl Pts',(0.761226690483986,-1.,-1.96890351582545));
#31977=CARTESIAN_POINT('Ctrl Pts',(0.761226690483986,1.,-1.96890351582545));
#31978=CARTESIAN_POINT('Ctrl Pts',(0.760552825409855,-1.,-1.97516705321521));
#31979=CARTESIAN_POINT('Ctrl Pts',(0.760552825409855,1.,-1.97516705321521));
#31980=CARTESIAN_POINT('Ctrl Pts',(0.759837147452135,-1.,-1.98143741418156));
#31981=CARTESIAN_POINT('Ctrl Pts',(0.759837147452135,1.,-1.98143741418156));
#31982=CARTESIAN_POINT('Ctrl Pts',(0.759080037802242,-1.,-1.98771456680806));
#31983=CARTESIAN_POINT('Ctrl Pts',(0.759080037802242,1.,-1.98771456680806));
#31984=CARTESIAN_POINT('Ctrl Pts',(0.758281796766377,-1.,-1.9939983109871));
#31985=CARTESIAN_POINT('Ctrl Pts',(0.758281796766377,1.,-1.9939983109871));
#31986=CARTESIAN_POINT('Ctrl Pts',(0.757442676862341,-1.,-2.00028834739072));
#31987=CARTESIAN_POINT('Ctrl Pts',(0.757442676862341,1.,-2.00028834739072));
#31988=CARTESIAN_POINT('Ctrl Pts',(0.756562904646496,-1.,-2.00658431587682));
#31989=CARTESIAN_POINT('Ctrl Pts',(0.756562904646496,1.,-2.00658431587682));
#31990=CARTESIAN_POINT('Ctrl Pts',(0.7556427049581,-1.,-2.01288584328149));
#31991=CARTESIAN_POINT('Ctrl Pts',(0.7556427049581,1.,-2.01288584328149));
#31992=CARTESIAN_POINT('Ctrl Pts',(0.75468233072352,-1.,-2.01919259406003));
#31993=CARTESIAN_POINT('Ctrl Pts',(0.75468233072352,1.,-2.01919259406003));
#31994=CARTESIAN_POINT('Ctrl Pts',(0.753682061113765,-1.,-2.02550428623587));
#31995=CARTESIAN_POINT('Ctrl Pts',(0.753682061113765,1.,-2.02550428623587));
#31996=CARTESIAN_POINT('Ctrl Pts',(0.752642180488104,-1.,-2.03182068456467));
#31997=CARTESIAN_POINT('Ctrl Pts',(0.752642180488104,1.,-2.03182068456467));
#31998=CARTESIAN_POINT('Ctrl Pts',(0.751562963361383,-1.,-2.03814160092173));
#31999=CARTESIAN_POINT('Ctrl Pts',(0.751562963361383,1.,-2.03814160092173));
#32000=CARTESIAN_POINT('Ctrl Pts',(0.750444657874758,-1.,-2.04446689147754));
#32001=CARTESIAN_POINT('Ctrl Pts',(0.750444657874758,1.,-2.04446689147754));
#32002=CARTESIAN_POINT('Ctrl Pts',(0.749287468663053,-1.,-2.05079645591606));
#32003=CARTESIAN_POINT('Ctrl Pts',(0.749287468663053,1.,-2.05079645591606));
#32004=CARTESIAN_POINT('Ctrl Pts',(0.748091554181101,-1.,-2.05713023030263));
#32005=CARTESIAN_POINT('Ctrl Pts',(0.748091554181101,1.,-2.05713023030263));
#32006=CARTESIAN_POINT('Ctrl Pts',(0.747103932785504,-1.,-2.06220058927162));
#32007=CARTESIAN_POINT('Ctrl Pts',(0.747103932785504,1.,-2.06220058927162));
#32008=CARTESIAN_POINT('Ctrl Pts',(0.746345871542695,-1.,-2.06600523016401));
#32009=CARTESIAN_POINT('Ctrl Pts',(0.746345871542695,1.,-2.06600523016401));
#32010=CARTESIAN_POINT('Ctrl Pts',(0.74583279137781,-1.,-2.06854248895575));
#32011=CARTESIAN_POINT('Ctrl Pts',(0.74583279137781,1.,-2.06854248895575));
#32012=CARTESIAN_POINT('Ctrl Pts',(0.745574324794401,-1.,-2.0698113262342));
#32013=CARTESIAN_POINT('Ctrl Pts',(0.745574324794401,1.,-2.0698113262342));
#32014=CARTESIAN_POINT('',(0.693717979106306,1.,-1.60662857109684));
#32015=CARTESIAN_POINT('Ctrl Pts',(0.693717979106306,1.,-1.60662857109684));
#32016=CARTESIAN_POINT('Ctrl Pts',(0.695712097881194,1.,-1.61106790958151));
#32017=CARTESIAN_POINT('Ctrl Pts',(0.699605146405088,1.,-1.61974673472612));
#32018=CARTESIAN_POINT('Ctrl Pts',(0.705159151988319,1.,-1.63216541664676));
#32019=CARTESIAN_POINT('Ctrl Pts',(0.711993139355394,1.,-1.64752408832016));
#32020=CARTESIAN_POINT('Ctrl Pts',(0.719585433804282,1.,-1.6647288055568));
#32021=CARTESIAN_POINT('Ctrl Pts',(0.726235967997433,1.,-1.67996158455503));
#32022=CARTESIAN_POINT('Ctrl Pts',(0.731963238697195,1.,-1.69326921975743));
#32023=CARTESIAN_POINT('Ctrl Pts',(0.736799665724771,1.,-1.70473309006121));
#32024=CARTESIAN_POINT('Ctrl Pts',(0.740795162032087,1.,-1.71447789751927));
#32025=CARTESIAN_POINT('Ctrl Pts',(0.744021445433764,1.,-1.7226822991693));
#32026=CARTESIAN_POINT('Ctrl Pts',(0.746574710096436,1.,-1.72958533647399));
#32027=CARTESIAN_POINT('Ctrl Pts',(0.748582462954854,1.,-1.73550351679848));
#32028=CARTESIAN_POINT('Ctrl Pts',(0.75019343597954,1.,-1.74080458266705));
#32029=CARTESIAN_POINT('Ctrl Pts',(0.751555614163629,1.,-1.74585086852298));
#32030=CARTESIAN_POINT('Ctrl Pts',(0.752797683531377,1.,-1.75095139468809));
#32031=CARTESIAN_POINT('Ctrl Pts',(0.75400925402848,1.,-1.75631083600175));
#32032=CARTESIAN_POINT('Ctrl Pts',(0.755220979975262,1.,-1.7619781724032));
#32033=CARTESIAN_POINT('Ctrl Pts',(0.756421896028403,1.,-1.76789396003141));
#32034=CARTESIAN_POINT('Ctrl Pts',(0.757578264077238,1.,-1.77394167108342));
#32035=CARTESIAN_POINT('Ctrl Pts',(0.75865062667738,1.,-1.77999411220912));
#32036=CARTESIAN_POINT('Ctrl Pts',(0.759614401109868,1.,-1.78596964884527));
#32037=CARTESIAN_POINT('Ctrl Pts',(0.760469555880425,1.,-1.79185815610802));
#32038=CARTESIAN_POINT('Ctrl Pts',(0.761229695230359,1.,-1.79768986997735));
#32039=CARTESIAN_POINT('Ctrl Pts',(0.761915336443515,1.,-1.80351583877334));
#32040=CARTESIAN_POINT('Ctrl Pts',(0.762546129464036,1.,-1.80938551463989));
#32041=CARTESIAN_POINT('Ctrl Pts',(0.763132003836783,1.,-1.81532118405566));
#32042=CARTESIAN_POINT('Ctrl Pts',(0.763673465462854,1.,-1.82131873145297));
#32043=CARTESIAN_POINT('Ctrl Pts',(0.764165902606055,1.,-1.8273599120008));
#32044=CARTESIAN_POINT('Ctrl Pts',(0.764602549687845,1.,-1.8334207722714));
#32045=CARTESIAN_POINT('Ctrl Pts',(0.764978057881687,1.,-1.83948181064823));
#32046=CARTESIAN_POINT('Ctrl Pts',(0.765291664861971,1.,-1.84553698875911));
#32047=CARTESIAN_POINT('Ctrl Pts',(0.765545710619023,1.,-1.85158945130054));
#32048=CARTESIAN_POINT('Ctrl Pts',(0.765744212909305,1.,-1.85764741390391));
#32049=CARTESIAN_POINT('Ctrl Pts',(0.765891519092557,1.,-1.86372027063315));
#32050=CARTESIAN_POINT('Ctrl Pts',(0.765990708546111,1.,-1.86981398314345));
#32051=CARTESIAN_POINT('Ctrl Pts',(0.766042837036759,1.,-1.87592888967886));
#32052=CARTESIAN_POINT('Ctrl Pts',(0.766047794851868,1.,-1.88206215302561));
#32053=CARTESIAN_POINT('Ctrl Pts',(0.76600483706209,1.,-1.88820926433409));
#32054=CARTESIAN_POINT('Ctrl Pts',(0.765913193856979,1.,-1.89436577771389));
#32055=CARTESIAN_POINT('Ctrl Pts',(0.765772772593395,1.,-1.90052930393599));
#32056=CARTESIAN_POINT('Ctrl Pts',(0.765584196937936,1.,-1.90669961402362));
#32057=CARTESIAN_POINT('Ctrl Pts',(0.765348465884739,1.,-1.91287765805174));
#32058=CARTESIAN_POINT('Ctrl Pts',(0.765066729667095,1.,-1.91906491634197));
#32059=CARTESIAN_POINT('Ctrl Pts',(0.764740025488189,1.,-1.92526263537041));
#32060=CARTESIAN_POINT('Ctrl Pts',(0.764369010673889,1.,-1.93147105496367));
#32061=CARTESIAN_POINT('Ctrl Pts',(0.763954049121393,1.,-1.93768964875867));
#32062=CARTESIAN_POINT('Ctrl Pts',(0.76349533353858,1.,-1.94391746617626));
#32063=CARTESIAN_POINT('Ctrl Pts',(0.762992990878774,1.,-1.95015342590025));
#32064=CARTESIAN_POINT('Ctrl Pts',(0.762447203806263,1.,-1.95639665309893));
#32065=CARTESIAN_POINT('Ctrl Pts',(0.761858300014575,1.,-1.96264672744229));
#32066=CARTESIAN_POINT('Ctrl Pts',(0.761226690483986,1.,-1.96890351582545));
#32067=CARTESIAN_POINT('Ctrl Pts',(0.760552825409855,1.,-1.97516705321521));
#32068=CARTESIAN_POINT('Ctrl Pts',(0.759837147452135,1.,-1.98143741418156));
#32069=CARTESIAN_POINT('Ctrl Pts',(0.759080037802242,1.,-1.98771456680806));
#32070=CARTESIAN_POINT('Ctrl Pts',(0.758281796766377,1.,-1.9939983109871));
#32071=CARTESIAN_POINT('Ctrl Pts',(0.757442676862341,1.,-2.00028834739072));
#32072=CARTESIAN_POINT('Ctrl Pts',(0.756562904646496,1.,-2.00658431587682));
#32073=CARTESIAN_POINT('Ctrl Pts',(0.7556427049581,1.,-2.01288584328149));
#32074=CARTESIAN_POINT('Ctrl Pts',(0.75468233072352,1.,-2.01919259406003));
#32075=CARTESIAN_POINT('Ctrl Pts',(0.753682061113765,1.,-2.02550428623587));
#32076=CARTESIAN_POINT('Ctrl Pts',(0.752642180488104,1.,-2.03182068456467));
#32077=CARTESIAN_POINT('Ctrl Pts',(0.751562963361383,1.,-2.03814160092173));
#32078=CARTESIAN_POINT('Ctrl Pts',(0.750444657874758,1.,-2.04446689147754));
#32079=CARTESIAN_POINT('Ctrl Pts',(0.749287468663053,1.,-2.05079645591606));
#32080=CARTESIAN_POINT('Ctrl Pts',(0.748091554181101,1.,-2.05713023030263));
#32081=CARTESIAN_POINT('Ctrl Pts',(0.747103932785504,1.,-2.06220058927162));
#32082=CARTESIAN_POINT('Ctrl Pts',(0.746345871542695,1.,-2.06600523016401));
#32083=CARTESIAN_POINT('Ctrl Pts',(0.74583279137781,1.,-2.06854248895575));
#32084=CARTESIAN_POINT('Ctrl Pts',(0.745574324794401,1.,-2.0698113262342));
#32085=CARTESIAN_POINT('',(0.693717979106306,0.,-1.60662857109684));
#32086=CARTESIAN_POINT('Origin',(0.,0.,0.));
#32087=CARTESIAN_POINT('',(0.892032620296855,1.,-1.5055822144029));
#32088=CARTESIAN_POINT('Origin',(0.,1.,0.));
#32089=CARTESIAN_POINT('',(0.892032620296855,0.,-1.5055822144029));
#32090=CARTESIAN_POINT('Ctrl Pts',(1.23627494547115,-1.,-1.81978687191668));
#32091=CARTESIAN_POINT('Ctrl Pts',(1.23627494547115,1.,-1.81978687191668));
#32092=CARTESIAN_POINT('Ctrl Pts',(1.23509651170476,-1.,-1.81925017193666));
#32093=CARTESIAN_POINT('Ctrl Pts',(1.23509651170476,1.,-1.81925017193666));
#32094=CARTESIAN_POINT('Ctrl Pts',(1.2327422452705,-1.,-1.81817389921279));
#32095=CARTESIAN_POINT('Ctrl Pts',(1.2327422452705,1.,-1.81817389921279));
#32096=CARTESIAN_POINT('Ctrl Pts',(1.2292186489137,-1.,-1.8165508718364));
#32097=CARTESIAN_POINT('Ctrl Pts',(1.2292186489137,1.,-1.8165508718364));
#32098=CARTESIAN_POINT('Ctrl Pts',(1.2245361330495,-1.,-1.81436959210434));
#32099=CARTESIAN_POINT('Ctrl Pts',(1.2245361330495,1.,-1.81436959210434));
#32100=CARTESIAN_POINT('Ctrl Pts',(1.21870906103557,-1.,-1.81161420806656));
#32101=CARTESIAN_POINT('Ctrl Pts',(1.21870906103557,1.,-1.81161420806656));
#32102=CARTESIAN_POINT('Ctrl Pts',(1.21290815708314,-1.,-1.80882996917129));
#32103=CARTESIAN_POINT('Ctrl Pts',(1.21290815708314,1.,-1.80882996917129));
#32104=CARTESIAN_POINT('Ctrl Pts',(1.20713356605475,-1.,-1.80601678480707));
#32105=CARTESIAN_POINT('Ctrl Pts',(1.20713356605475,1.,-1.80601678480707));
#32106=CARTESIAN_POINT('Ctrl Pts',(1.20138548938974,-1.,-1.80317454838603));
#32107=CARTESIAN_POINT('Ctrl Pts',(1.20138548938974,1.,-1.80317454838603));
#32108=CARTESIAN_POINT('Ctrl Pts',(1.19566418930242,-1.,-1.80030314369879));
#32109=CARTESIAN_POINT('Ctrl Pts',(1.19566418930242,1.,-1.80030314369879));
#32110=CARTESIAN_POINT('Ctrl Pts',(1.18996997934445,-1.,-1.79740245923478));
#32111=CARTESIAN_POINT('Ctrl Pts',(1.18996997934445,1.,-1.79740245923478));
#32112=CARTESIAN_POINT('Ctrl Pts',(1.18430321697432,-1.,-1.79447240321515));
#32113=CARTESIAN_POINT('Ctrl Pts',(1.18430321697432,1.,-1.79447240321515));
#32114=CARTESIAN_POINT('Ctrl Pts',(1.17866429440809,-1.,-1.79151291552689));
#32115=CARTESIAN_POINT('Ctrl Pts',(1.17866429440809,1.,-1.79151291552689));
#32116=CARTESIAN_POINT('Ctrl Pts',(1.17305363177328,-1.,-1.78852398877617));
#32117=CARTESIAN_POINT('Ctrl Pts',(1.17305363177328,1.,-1.78852398877617));
#32118=CARTESIAN_POINT('Ctrl Pts',(1.16747166312303,-1.,-1.78550566040443));
#32119=CARTESIAN_POINT('Ctrl Pts',(1.16747166312303,1.,-1.78550566040443));
#32120=CARTESIAN_POINT('Ctrl Pts',(1.16191881298499,-1.,-1.78245795881009));
#32121=CARTESIAN_POINT('Ctrl Pts',(1.16191881298499,1.,-1.78245795881009));
#32122=CARTESIAN_POINT('Ctrl Pts',(1.15639547194698,-1.,-1.77938085564275));
#32123=CARTESIAN_POINT('Ctrl Pts',(1.15639547194698,1.,-1.77938085564275));
#32124=CARTESIAN_POINT('Ctrl Pts',(1.15090197841514,-1.,-1.7762742255701));
#32125=CARTESIAN_POINT('Ctrl Pts',(1.15090197841514,1.,-1.7762742255701));
#32126=CARTESIAN_POINT('Ctrl Pts',(1.1454385822692,-1.,-1.77313777896194));
#32127=CARTESIAN_POINT('Ctrl Pts',(1.1454385822692,1.,-1.77313777896194));
#32128=CARTESIAN_POINT('Ctrl Pts',(1.14000548336975,-1.,-1.76997111386769));
#32129=CARTESIAN_POINT('Ctrl Pts',(1.14000548336975,1.,-1.76997111386769));
#32130=CARTESIAN_POINT('Ctrl Pts',(1.1346029180462,-1.,-1.76677384551862));
#32131=CARTESIAN_POINT('Ctrl Pts',(1.1346029180462,1.,-1.76677384551862));
#32132=CARTESIAN_POINT('Ctrl Pts',(1.12923123555075,-1.,-1.7635457196617));
#32133=CARTESIAN_POINT('Ctrl Pts',(1.12923123555075,1.,-1.7635457196617));
#32134=CARTESIAN_POINT('Ctrl Pts',(1.12389096855086,-1.,-1.76028671825096));
#32135=CARTESIAN_POINT('Ctrl Pts',(1.12389096855086,1.,-1.76028671825096));
#32136=CARTESIAN_POINT('Ctrl Pts',(1.11858293216763,-1.,-1.75699720772105));
#32137=CARTESIAN_POINT('Ctrl Pts',(1.11858293216763,1.,-1.75699720772105));
#32138=CARTESIAN_POINT('Ctrl Pts',(1.11330807582551,-1.,-1.7536777209463));
#32139=CARTESIAN_POINT('Ctrl Pts',(1.11330807582551,1.,-1.7536777209463));
#32140=CARTESIAN_POINT('Ctrl Pts',(1.10806728183007,-1.,-1.7503286607592));
#32141=CARTESIAN_POINT('Ctrl Pts',(1.10806728183007,1.,-1.7503286607592));
#32142=CARTESIAN_POINT('Ctrl Pts',(1.10286118991143,-1.,-1.74695004214923));
#32143=CARTESIAN_POINT('Ctrl Pts',(1.10286118991143,1.,-1.74695004214923));
#32144=CARTESIAN_POINT('Ctrl Pts',(1.09768999241225,-1.,-1.74354119236208));
#32145=CARTESIAN_POINT('Ctrl Pts',(1.09768999241225,1.,-1.74354119236208));
#32146=CARTESIAN_POINT('Ctrl Pts',(1.09255329056493,-1.,-1.74010053962247));
#32147=CARTESIAN_POINT('Ctrl Pts',(1.09255329056493,1.,-1.74010053962247));
#32148=CARTESIAN_POINT('Ctrl Pts',(1.08745056285427,-1.,-1.73662628326091));
#32149=CARTESIAN_POINT('Ctrl Pts',(1.08745056285427,1.,-1.73662628326091));
#32150=CARTESIAN_POINT('Ctrl Pts',(1.08238162784749,-1.,-1.73311705663407));
#32151=CARTESIAN_POINT('Ctrl Pts',(1.08238162784749,1.,-1.73311705663407));
#32152=CARTESIAN_POINT('Ctrl Pts',(1.0773470373727,-1.,-1.72957248977424));
#32153=CARTESIAN_POINT('Ctrl Pts',(1.0773470373727,1.,-1.72957248977424));
#32154=CARTESIAN_POINT('Ctrl Pts',(1.07234866990252,-1.,-1.72599406198488));
#32155=CARTESIAN_POINT('Ctrl Pts',(1.07234866990252,1.,-1.72599406198488));
#32156=CARTESIAN_POINT('Ctrl Pts',(1.06738966975462,-1.,-1.72238500928453));
#32157=CARTESIAN_POINT('Ctrl Pts',(1.06738966975462,1.,-1.72238500928453));
#32158=CARTESIAN_POINT('Ctrl Pts',(1.06247324680647,-1.,-1.71874858456904));
#32159=CARTESIAN_POINT('Ctrl Pts',(1.06247324680647,1.,-1.71874858456904));
#32160=CARTESIAN_POINT('Ctrl Pts',(1.05760163192479,-1.,-1.7150865442702));
#32161=CARTESIAN_POINT('Ctrl Pts',(1.05760163192479,1.,-1.7150865442702));
#32162=CARTESIAN_POINT('Ctrl Pts',(1.05277517202855,-1.,-1.71139783543989));
#32163=CARTESIAN_POINT('Ctrl Pts',(1.05277517202855,1.,-1.71139783543989));
#32164=CARTESIAN_POINT('Ctrl Pts',(1.04799085404995,-1.,-1.70767646263649));
#32165=CARTESIAN_POINT('Ctrl Pts',(1.04799085404995,1.,-1.70767646263649));
#32166=CARTESIAN_POINT('Ctrl Pts',(1.04324363334554,-1.,-1.70391338707982));
#32167=CARTESIAN_POINT('Ctrl Pts',(1.04324363334554,1.,-1.70391338707982));
#32168=CARTESIAN_POINT('Ctrl Pts',(1.03852922490789,-1.,-1.70010052930962));
#32169=CARTESIAN_POINT('Ctrl Pts',(1.03852922490789,1.,-1.70010052930962));
#32170=CARTESIAN_POINT('Ctrl Pts',(1.03384646003588,-1.,-1.69623414782771));
#32171=CARTESIAN_POINT('Ctrl Pts',(1.03384646003588,1.,-1.69623414782771));
#32172=CARTESIAN_POINT('Ctrl Pts',(1.02919977579147,-1.,-1.69231840863458));
#32173=CARTESIAN_POINT('Ctrl Pts',(1.02919977579147,1.,-1.69231840863458));
#32174=CARTESIAN_POINT('Ctrl Pts',(1.02460180535255,-1.,-1.68836910178447));
#32175=CARTESIAN_POINT('Ctrl Pts',(1.02460180535255,1.,-1.68836910178447));
#32176=CARTESIAN_POINT('Ctrl Pts',(1.02006795074201,-1.,-1.68440578021706));
#32177=CARTESIAN_POINT('Ctrl Pts',(1.02006795074201,1.,-1.68440578021706));
#32178=CARTESIAN_POINT('Ctrl Pts',(1.01561026162773,-1.,-1.68044289894798));
#32179=CARTESIAN_POINT('Ctrl Pts',(1.01561026162773,1.,-1.68044289894798));
#32180=CARTESIAN_POINT('Ctrl Pts',(1.01123236493511,-1.,-1.67648246776464));
#32181=CARTESIAN_POINT('Ctrl Pts',(1.01123236493511,1.,-1.67648246776464));
#32182=CARTESIAN_POINT('Ctrl Pts',(1.00692206696414,-1.,-1.67250335383293));
#32183=CARTESIAN_POINT('Ctrl Pts',(1.00692206696414,1.,-1.67250335383293));
#32184=CARTESIAN_POINT('Ctrl Pts',(1.00265091003727,-1.,-1.66846059277303));
#32185=CARTESIAN_POINT('Ctrl Pts',(1.00265091003727,1.,-1.66846059277303));
#32186=CARTESIAN_POINT('Ctrl Pts',(0.998389654952757,-1.,-1.66430758030376));
#32187=CARTESIAN_POINT('Ctrl Pts',(0.998389654952757,1.,-1.66430758030376));
#32188=CARTESIAN_POINT('Ctrl Pts',(0.994121836661305,-1.,-1.66001553809947));
#32189=CARTESIAN_POINT('Ctrl Pts',(0.994121836661305,1.,-1.66001553809947));
#32190=CARTESIAN_POINT('Ctrl Pts',(0.989855627854164,-1.,-1.65559044289699));
#32191=CARTESIAN_POINT('Ctrl Pts',(0.989855627854164,1.,-1.65559044289699));
#32192=CARTESIAN_POINT('Ctrl Pts',(0.98564262292082,-1.,-1.65110016612638));
#32193=CARTESIAN_POINT('Ctrl Pts',(0.98564262292082,1.,-1.65110016612638));
#32194=CARTESIAN_POINT('Ctrl Pts',(0.981562530939489,-1.,-1.64665139190656));
#32195=CARTESIAN_POINT('Ctrl Pts',(0.981562530939489,1.,-1.64665139190656));
#32196=CARTESIAN_POINT('Ctrl Pts',(0.977689794119416,-1.,-1.64233990826687));
#32197=CARTESIAN_POINT('Ctrl Pts',(0.977689794119416,1.,-1.64233990826687));
#32198=CARTESIAN_POINT('Ctrl Pts',(0.974066058287418,-1.,-1.63820952658144));
#32199=CARTESIAN_POINT('Ctrl Pts',(0.974066058287418,1.,-1.63820952658144));
#32200=CARTESIAN_POINT('Ctrl Pts',(0.970669715997509,-1.,-1.63420665729798));
#32201=CARTESIAN_POINT('Ctrl Pts',(0.970669715997509,1.,-1.63420665729798));
#32202=CARTESIAN_POINT('Ctrl Pts',(0.967387853230345,-1.,-1.63013849959462));
#32203=CARTESIAN_POINT('Ctrl Pts',(0.967387853230345,1.,-1.63013849959462));
#32204=CARTESIAN_POINT('Ctrl Pts',(0.964046107040535,-1.,-1.62571930670187));
#32205=CARTESIAN_POINT('Ctrl Pts',(0.964046107040535,1.,-1.62571930670187));
#32206=CARTESIAN_POINT('Ctrl Pts',(0.960438326101728,-1.,-1.62061638140221));
#32207=CARTESIAN_POINT('Ctrl Pts',(0.960438326101728,1.,-1.62061638140221));
#32208=CARTESIAN_POINT('Ctrl Pts',(0.95635442292067,-1.,-1.61449324337085));
#32209=CARTESIAN_POINT('Ctrl Pts',(0.95635442292067,1.,-1.61449324337085));
#32210=CARTESIAN_POINT('Ctrl Pts',(0.951613284356035,-1.,-1.60706069896936));
#32211=CARTESIAN_POINT('Ctrl Pts',(0.951613284356035,1.,-1.60706069896936));
#32212=CARTESIAN_POINT('Ctrl Pts',(0.946078063315257,-1.,-1.59810042043673));
#32213=CARTESIAN_POINT('Ctrl Pts',(0.946078063315257,1.,-1.59810042043673));
#32214=CARTESIAN_POINT('Ctrl Pts',(0.939646377893399,-1.,-1.58744937487176));
#32215=CARTESIAN_POINT('Ctrl Pts',(0.939646377893399,1.,-1.58744937487176));
#32216=CARTESIAN_POINT('Ctrl Pts',(0.932246680108685,-1.,-1.57499388382243));
#32217=CARTESIAN_POINT('Ctrl Pts',(0.932246680108685,1.,-1.57499388382243));
#32218=CARTESIAN_POINT('Ctrl Pts',(0.923832188944341,-1.,-1.56065988578893));
#32219=CARTESIAN_POINT('Ctrl Pts',(0.923832188944341,1.,-1.56065988578893));
#32220=CARTESIAN_POINT('Ctrl Pts',(0.914375919026456,-1.,-1.54440491149498));
#32221=CARTESIAN_POINT('Ctrl Pts',(0.914375919026456,1.,-1.54440491149498));
#32222=CARTESIAN_POINT('Ctrl Pts',(0.905967409625651,-1.,-1.52984849887993));
#32223=CARTESIAN_POINT('Ctrl Pts',(0.905967409625651,1.,-1.52984849887993));
#32224=CARTESIAN_POINT('Ctrl Pts',(0.89918504748351,-1.,-1.51805569590094));
#32225=CARTESIAN_POINT('Ctrl Pts',(0.89918504748351,1.,-1.51805569590094));
#32226=CARTESIAN_POINT('Ctrl Pts',(0.894452006964543,-1.,-1.50980486806688));
#32227=CARTESIAN_POINT('Ctrl Pts',(0.894452006964543,1.,-1.50980486806688));
#32228=CARTESIAN_POINT('Ctrl Pts',(0.892032620296855,-1.,-1.5055822144029));
#32229=CARTESIAN_POINT('Ctrl Pts',(0.892032620296855,1.,-1.5055822144029));
#32230=CARTESIAN_POINT('',(1.23627494547115,1.,-1.81978687191668));
#32231=CARTESIAN_POINT('Ctrl Pts',(1.23627494547115,1.,-1.81978687191668));
#32232=CARTESIAN_POINT('Ctrl Pts',(1.23509651170476,1.,-1.81925017193666));
#32233=CARTESIAN_POINT('Ctrl Pts',(1.2327422452705,1.,-1.81817389921279));
#32234=CARTESIAN_POINT('Ctrl Pts',(1.2292186489137,1.,-1.8165508718364));
#32235=CARTESIAN_POINT('Ctrl Pts',(1.2245361330495,1.,-1.81436959210434));
#32236=CARTESIAN_POINT('Ctrl Pts',(1.21870906103557,1.,-1.81161420806656));
#32237=CARTESIAN_POINT('Ctrl Pts',(1.21290815708314,1.,-1.80882996917129));
#32238=CARTESIAN_POINT('Ctrl Pts',(1.20713356605475,1.,-1.80601678480707));
#32239=CARTESIAN_POINT('Ctrl Pts',(1.20138548938974,1.,-1.80317454838603));
#32240=CARTESIAN_POINT('Ctrl Pts',(1.19566418930242,1.,-1.80030314369879));
#32241=CARTESIAN_POINT('Ctrl Pts',(1.18996997934445,1.,-1.79740245923478));
#32242=CARTESIAN_POINT('Ctrl Pts',(1.18430321697432,1.,-1.79447240321515));
#32243=CARTESIAN_POINT('Ctrl Pts',(1.17866429440809,1.,-1.79151291552689));
#32244=CARTESIAN_POINT('Ctrl Pts',(1.17305363177328,1.,-1.78852398877617));
#32245=CARTESIAN_POINT('Ctrl Pts',(1.16747166312303,1.,-1.78550566040443));
#32246=CARTESIAN_POINT('Ctrl Pts',(1.16191881298499,1.,-1.78245795881009));
#32247=CARTESIAN_POINT('Ctrl Pts',(1.15639547194698,1.,-1.77938085564275));
#32248=CARTESIAN_POINT('Ctrl Pts',(1.15090197841514,1.,-1.7762742255701));
#32249=CARTESIAN_POINT('Ctrl Pts',(1.1454385822692,1.,-1.77313777896194));
#32250=CARTESIAN_POINT('Ctrl Pts',(1.14000548336975,1.,-1.76997111386769));
#32251=CARTESIAN_POINT('Ctrl Pts',(1.1346029180462,1.,-1.76677384551862));
#32252=CARTESIAN_POINT('Ctrl Pts',(1.12923123555075,1.,-1.7635457196617));
#32253=CARTESIAN_POINT('Ctrl Pts',(1.12389096855086,1.,-1.76028671825096));
#32254=CARTESIAN_POINT('Ctrl Pts',(1.11858293216763,1.,-1.75699720772105));
#32255=CARTESIAN_POINT('Ctrl Pts',(1.11330807582551,1.,-1.7536777209463));
#32256=CARTESIAN_POINT('Ctrl Pts',(1.10806728183007,1.,-1.7503286607592));
#32257=CARTESIAN_POINT('Ctrl Pts',(1.10286118991143,1.,-1.74695004214923));
#32258=CARTESIAN_POINT('Ctrl Pts',(1.09768999241225,1.,-1.74354119236208));
#32259=CARTESIAN_POINT('Ctrl Pts',(1.09255329056493,1.,-1.74010053962247));
#32260=CARTESIAN_POINT('Ctrl Pts',(1.08745056285427,1.,-1.73662628326091));
#32261=CARTESIAN_POINT('Ctrl Pts',(1.08238162784749,1.,-1.73311705663407));
#32262=CARTESIAN_POINT('Ctrl Pts',(1.0773470373727,1.,-1.72957248977424));
#32263=CARTESIAN_POINT('Ctrl Pts',(1.07234866990252,1.,-1.72599406198488));
#32264=CARTESIAN_POINT('Ctrl Pts',(1.06738966975462,1.,-1.72238500928453));
#32265=CARTESIAN_POINT('Ctrl Pts',(1.06247324680647,1.,-1.71874858456904));
#32266=CARTESIAN_POINT('Ctrl Pts',(1.05760163192479,1.,-1.7150865442702));
#32267=CARTESIAN_POINT('Ctrl Pts',(1.05277517202855,1.,-1.71139783543989));
#32268=CARTESIAN_POINT('Ctrl Pts',(1.04799085404995,1.,-1.70767646263649));
#32269=CARTESIAN_POINT('Ctrl Pts',(1.04324363334554,1.,-1.70391338707982));
#32270=CARTESIAN_POINT('Ctrl Pts',(1.03852922490789,1.,-1.70010052930962));
#32271=CARTESIAN_POINT('Ctrl Pts',(1.03384646003588,1.,-1.69623414782771));
#32272=CARTESIAN_POINT('Ctrl Pts',(1.02919977579147,1.,-1.69231840863458));
#32273=CARTESIAN_POINT('Ctrl Pts',(1.02460180535255,1.,-1.68836910178447));
#32274=CARTESIAN_POINT('Ctrl Pts',(1.02006795074201,1.,-1.68440578021706));
#32275=CARTESIAN_POINT('Ctrl Pts',(1.01561026162773,1.,-1.68044289894798));
#32276=CARTESIAN_POINT('Ctrl Pts',(1.01123236493511,1.,-1.67648246776464));
#32277=CARTESIAN_POINT('Ctrl Pts',(1.00692206696414,1.,-1.67250335383293));
#32278=CARTESIAN_POINT('Ctrl Pts',(1.00265091003727,1.,-1.66846059277303));
#32279=CARTESIAN_POINT('Ctrl Pts',(0.998389654952757,1.,-1.66430758030376));
#32280=CARTESIAN_POINT('Ctrl Pts',(0.994121836661305,1.,-1.66001553809947));
#32281=CARTESIAN_POINT('Ctrl Pts',(0.989855627854164,1.,-1.65559044289699));
#32282=CARTESIAN_POINT('Ctrl Pts',(0.98564262292082,1.,-1.65110016612638));
#32283=CARTESIAN_POINT('Ctrl Pts',(0.981562530939489,1.,-1.64665139190656));
#32284=CARTESIAN_POINT('Ctrl Pts',(0.977689794119416,1.,-1.64233990826687));
#32285=CARTESIAN_POINT('Ctrl Pts',(0.974066058287418,1.,-1.63820952658144));
#32286=CARTESIAN_POINT('Ctrl Pts',(0.970669715997509,1.,-1.63420665729798));
#32287=CARTESIAN_POINT('Ctrl Pts',(0.967387853230345,1.,-1.63013849959462));
#32288=CARTESIAN_POINT('Ctrl Pts',(0.964046107040535,1.,-1.62571930670187));
#32289=CARTESIAN_POINT('Ctrl Pts',(0.960438326101728,1.,-1.62061638140221));
#32290=CARTESIAN_POINT('Ctrl Pts',(0.95635442292067,1.,-1.61449324337085));
#32291=CARTESIAN_POINT('Ctrl Pts',(0.951613284356035,1.,-1.60706069896936));
#32292=CARTESIAN_POINT('Ctrl Pts',(0.946078063315257,1.,-1.59810042043673));
#32293=CARTESIAN_POINT('Ctrl Pts',(0.939646377893399,1.,-1.58744937487176));
#32294=CARTESIAN_POINT('Ctrl Pts',(0.932246680108685,1.,-1.57499388382243));
#32295=CARTESIAN_POINT('Ctrl Pts',(0.923832188944341,1.,-1.56065988578893));
#32296=CARTESIAN_POINT('Ctrl Pts',(0.914375919026456,1.,-1.54440491149498));
#32297=CARTESIAN_POINT('Ctrl Pts',(0.905967409625651,1.,-1.52984849887993));
#32298=CARTESIAN_POINT('Ctrl Pts',(0.89918504748351,1.,-1.51805569590094));
#32299=CARTESIAN_POINT('Ctrl Pts',(0.894452006964543,1.,-1.50980486806688));
#32300=CARTESIAN_POINT('Ctrl Pts',(0.892032620296855,1.,-1.5055822144029));
#32301=CARTESIAN_POINT('',(1.23627494547115,0.,-1.81978687191668));
#32302=CARTESIAN_POINT('Origin',(1.34869019493419,0.,-1.73811241238545));
#32303=CARTESIAN_POINT('',(1.34869019493419,1.,-1.73811241238545));
#32304=CARTESIAN_POINT('',(1.23627494547115,1.,-1.81978687191668));
#32305=CARTESIAN_POINT('',(1.34869019493419,0.,-1.73811241238545));
#32306=CARTESIAN_POINT('Ctrl Pts',(1.15624053661742,-1.,-1.31362392696032));
#32307=CARTESIAN_POINT('Ctrl Pts',(1.15624053661742,1.,-1.31362392696032));
#32308=CARTESIAN_POINT('Ctrl Pts',(1.15950888730809,-1.,-1.31722977216397));
#32309=CARTESIAN_POINT('Ctrl Pts',(1.15950888730809,1.,-1.31722977216397));
#32310=CARTESIAN_POINT('Ctrl Pts',(1.16589330093588,-1.,-1.32428080721772));
#32311=CARTESIAN_POINT('Ctrl Pts',(1.16589330093588,1.,-1.32428080721772));
#32312=CARTESIAN_POINT('Ctrl Pts',(1.17501305789857,-1.,-1.33437539347008));
#32313=CARTESIAN_POINT('Ctrl Pts',(1.17501305789857,1.,-1.33437539347008));
#32314=CARTESIAN_POINT('Ctrl Pts',(1.18625865667441,-1.,-1.34687054001093));
#32315=CARTESIAN_POINT('Ctrl Pts',(1.18625865667441,1.,-1.34687054001093));
#32316=CARTESIAN_POINT('Ctrl Pts',(1.1987959077932,-1.,-1.36088705043885));
#32317=CARTESIAN_POINT('Ctrl Pts',(1.1987959077932,1.,-1.36088705043885));
#32318=CARTESIAN_POINT('Ctrl Pts',(1.20982812925645,-1.,-1.37331915607905));
#32319=CARTESIAN_POINT('Ctrl Pts',(1.20982812925645,1.,-1.37331915607905));
#32320=CARTESIAN_POINT('Ctrl Pts',(1.21938737280852,-1.,-1.38420564527715));
#32321=CARTESIAN_POINT('Ctrl Pts',(1.21938737280852,1.,-1.38420564527715));
#32322=CARTESIAN_POINT('Ctrl Pts',(1.22752961899387,-1.,-1.39361389568796));
#32323=CARTESIAN_POINT('Ctrl Pts',(1.22752961899387,1.,-1.39361389568796));
#32324=CARTESIAN_POINT('Ctrl Pts',(1.23434087290423,-1.,-1.40164708206106));
#32325=CARTESIAN_POINT('Ctrl Pts',(1.23434087290423,1.,-1.40164708206106));
#32326=CARTESIAN_POINT('Ctrl Pts',(1.23994455029534,-1.,-1.40845295531283));
#32327=CARTESIAN_POINT('Ctrl Pts',(1.23994455029534,1.,-1.40845295531283));
#32328=CARTESIAN_POINT('Ctrl Pts',(1.24450600513056,-1.,-1.41422913175179));
#32329=CARTESIAN_POINT('Ctrl Pts',(1.24450600513056,1.,-1.41422913175179));
#32330=CARTESIAN_POINT('Ctrl Pts',(1.24824430986571,-1.,-1.41923722596025));
#32331=CARTESIAN_POINT('Ctrl Pts',(1.24824430986571,1.,-1.41923722596025));
#32332=CARTESIAN_POINT('Ctrl Pts',(1.2514145557001,-1.,-1.42378102115575));
#32333=CARTESIAN_POINT('Ctrl Pts',(1.2514145557001,1.,-1.42378102115575));
#32334=CARTESIAN_POINT('Ctrl Pts',(1.25426945222639,-1.,-1.42815938799387));
#32335=CARTESIAN_POINT('Ctrl Pts',(1.25426945222639,1.,-1.42815938799387));
#32336=CARTESIAN_POINT('Ctrl Pts',(1.25702687965755,-1.,-1.43262645609691));
#32337=CARTESIAN_POINT('Ctrl Pts',(1.25702687965755,1.,-1.43262645609691));
#32338=CARTESIAN_POINT('Ctrl Pts',(1.25983531012005,-1.,-1.43734919180848));
#32339=CARTESIAN_POINT('Ctrl Pts',(1.25983531012005,1.,-1.43734919180848));
#32340=CARTESIAN_POINT('Ctrl Pts',(1.26273903323858,-1.,-1.44236470511303));
#32341=CARTESIAN_POINT('Ctrl Pts',(1.26273903323858,1.,-1.44236470511303));
#32342=CARTESIAN_POINT('Ctrl Pts',(1.26570925118868,-1.,-1.44761985001662));
#32343=CARTESIAN_POINT('Ctrl Pts',(1.26570925118868,1.,-1.44761985001662));
#32344=CARTESIAN_POINT('Ctrl Pts',(1.2686778680489,-1.,-1.45301422764247));
#32345=CARTESIAN_POINT('Ctrl Pts',(1.2686778680489,1.,-1.45301422764247));
#32346=CARTESIAN_POINT('Ctrl Pts',(1.27156805265289,-1.,-1.45843906294697));
#32347=CARTESIAN_POINT('Ctrl Pts',(1.27156805265289,1.,-1.45843906294697));
#32348=CARTESIAN_POINT('Ctrl Pts',(1.27433119897822,-1.,-1.46382431332476));
#32349=CARTESIAN_POINT('Ctrl Pts',(1.27433119897822,1.,-1.46382431332476));
#32350=CARTESIAN_POINT('Ctrl Pts',(1.27696414831089,-1.,-1.46916035917133));
#32351=CARTESIAN_POINT('Ctrl Pts',(1.27696414831089,1.,-1.46916035917133));
#32352=CARTESIAN_POINT('Ctrl Pts',(1.2794891824849,-1.,-1.4744717526707));
#32353=CARTESIAN_POINT('Ctrl Pts',(1.2794891824849,1.,-1.4744717526707));
#32354=CARTESIAN_POINT('Ctrl Pts',(1.28194158939517,-1.,-1.47980070347096));
#32355=CARTESIAN_POINT('Ctrl Pts',(1.28194158939517,1.,-1.47980070347096));
#32356=CARTESIAN_POINT('Ctrl Pts',(1.28435533880201,-1.,-1.4851881711891));
#32357=CARTESIAN_POINT('Ctrl Pts',(1.28435533880201,1.,-1.4851881711891));
#32358=CARTESIAN_POINT('Ctrl Pts',(1.2867467611644,-1.,-1.4906522831278));
#32359=CARTESIAN_POINT('Ctrl Pts',(1.2867467611644,1.,-1.4906522831278));
#32360=CARTESIAN_POINT('Ctrl Pts',(1.28911506584254,-1.,-1.49618896881754));
#32361=CARTESIAN_POINT('Ctrl Pts',(1.28911506584254,1.,-1.49618896881754));
#32362=CARTESIAN_POINT('Ctrl Pts',(1.29145022885181,-1.,-1.50178230149776));
#32363=CARTESIAN_POINT('Ctrl Pts',(1.29145022885181,1.,-1.50178230149776));
#32364=CARTESIAN_POINT('Ctrl Pts',(1.29373841372842,-1.,-1.50741159078365));
#32365=CARTESIAN_POINT('Ctrl Pts',(1.29373841372842,1.,-1.50741159078365));
#32366=CARTESIAN_POINT('Ctrl Pts',(1.29596850710509,-1.,-1.51305994241402));
#32367=CARTESIAN_POINT('Ctrl Pts',(1.29596850710509,1.,-1.51305994241402));
#32368=CARTESIAN_POINT('Ctrl Pts',(1.29813791800747,-1.,-1.51872184912724));
#32369=CARTESIAN_POINT('Ctrl Pts',(1.29813791800747,1.,-1.51872184912724));
#32370=CARTESIAN_POINT('Ctrl Pts',(1.30024984366328,-1.,-1.52439957861062));
#32371=CARTESIAN_POINT('Ctrl Pts',(1.30024984366328,1.,-1.52439957861062));
#32372=CARTESIAN_POINT('Ctrl Pts',(1.30231064395568,-1.,-1.53009970283891));
#32373=CARTESIAN_POINT('Ctrl Pts',(1.30231064395568,1.,-1.53009970283891));
#32374=CARTESIAN_POINT('Ctrl Pts',(1.30432735639489,-1.,-1.53582981268977));
#32375=CARTESIAN_POINT('Ctrl Pts',(1.30432735639489,1.,-1.53582981268977));
#32376=CARTESIAN_POINT('Ctrl Pts',(1.30630475189556,-1.,-1.54159462645432));
#32377=CARTESIAN_POINT('Ctrl Pts',(1.30630475189556,1.,-1.54159462645432));
#32378=CARTESIAN_POINT('Ctrl Pts',(1.30824393907473,-1.,-1.54739413957185));
#32379=CARTESIAN_POINT('Ctrl Pts',(1.30824393907473,1.,-1.54739413957185));
#32380=CARTESIAN_POINT('Ctrl Pts',(1.31014393684222,-1.,-1.55322568759481));
#32381=CARTESIAN_POINT('Ctrl Pts',(1.31014393684222,1.,-1.55322568759481));
#32382=CARTESIAN_POINT('Ctrl Pts',(1.31200264341696,-1.,-1.55908521254821));
#32383=CARTESIAN_POINT('Ctrl Pts',(1.31200264341696,1.,-1.55908521254821));
#32384=CARTESIAN_POINT('Ctrl Pts',(1.31381795281002,-1.,-1.56496872402353));
#32385=CARTESIAN_POINT('Ctrl Pts',(1.31381795281002,1.,-1.56496872402353));
#32386=CARTESIAN_POINT('Ctrl Pts',(1.31558903860016,-1.,-1.57087397835723));
#32387=CARTESIAN_POINT('Ctrl Pts',(1.31558903860016,1.,-1.57087397835723));
#32388=CARTESIAN_POINT('Ctrl Pts',(1.31731642317187,-1.,-1.5768005650559));
#32389=CARTESIAN_POINT('Ctrl Pts',(1.31731642317187,1.,-1.5768005650559));
#32390=CARTESIAN_POINT('Ctrl Pts',(1.31900135021432,-1.,-1.58274907898834));
#32391=CARTESIAN_POINT('Ctrl Pts',(1.31900135021432,1.,-1.58274907898834));
#32392=CARTESIAN_POINT('Ctrl Pts',(1.32064537110892,-1.,-1.58872057258245));
#32393=CARTESIAN_POINT('Ctrl Pts',(1.32064537110892,1.,-1.58872057258245));
#32394=CARTESIAN_POINT('Ctrl Pts',(1.32224985747682,-1.,-1.59471591079403));
#32395=CARTESIAN_POINT('Ctrl Pts',(1.32224985747682,1.,-1.59471591079403));
#32396=CARTESIAN_POINT('Ctrl Pts',(1.32381550858256,-1.,-1.60073511858687));
#32397=CARTESIAN_POINT('Ctrl Pts',(1.32381550858256,1.,-1.60073511858687));
#32398=CARTESIAN_POINT('Ctrl Pts',(1.32534250785782,-1.,-1.60677758290954));
#32399=CARTESIAN_POINT('Ctrl Pts',(1.32534250785782,1.,-1.60677758290954));
#32400=CARTESIAN_POINT('Ctrl Pts',(1.32683074483356,-1.,-1.6128423401575));
#32401=CARTESIAN_POINT('Ctrl Pts',(1.32683074483356,1.,-1.6128423401575));
#32402=CARTESIAN_POINT('Ctrl Pts',(1.32828000610449,-1.,-1.61892832270724));
#32403=CARTESIAN_POINT('Ctrl Pts',(1.32828000610449,1.,-1.61892832270724));
#32404=CARTESIAN_POINT('Ctrl Pts',(1.3296901950568,-1.,-1.62503464209797));
#32405=CARTESIAN_POINT('Ctrl Pts',(1.3296901950568,1.,-1.62503464209797));
#32406=CARTESIAN_POINT('Ctrl Pts',(1.33106149345645,-1.,-1.63116079730923));
#32407=CARTESIAN_POINT('Ctrl Pts',(1.33106149345645,1.,-1.63116079730923));
#32408=CARTESIAN_POINT('Ctrl Pts',(1.33239425103724,-1.,-1.63730653475089));
#32409=CARTESIAN_POINT('Ctrl Pts',(1.33239425103724,1.,-1.63730653475089));
#32410=CARTESIAN_POINT('Ctrl Pts',(1.33368890676572,-1.,-1.6434717485603));
#32411=CARTESIAN_POINT('Ctrl Pts',(1.33368890676572,1.,-1.6434717485603));
#32412=CARTESIAN_POINT('Ctrl Pts',(1.33494590467993,-1.,-1.6496563728683));
#32413=CARTESIAN_POINT('Ctrl Pts',(1.33494590467993,1.,-1.6496563728683));
#32414=CARTESIAN_POINT('Ctrl Pts',(1.33616559745172,-1.,-1.65586025952593));
#32415=CARTESIAN_POINT('Ctrl Pts',(1.33616559745172,1.,-1.65586025952593));
#32416=CARTESIAN_POINT('Ctrl Pts',(1.33734820885262,-1.,-1.66208312541983));
#32417=CARTESIAN_POINT('Ctrl Pts',(1.33734820885262,1.,-1.66208312541983));
#32418=CARTESIAN_POINT('Ctrl Pts',(1.33849388654388,-1.,-1.66832460783989));
#32419=CARTESIAN_POINT('Ctrl Pts',(1.33849388654388,1.,-1.66832460783989));
#32420=CARTESIAN_POINT('Ctrl Pts',(1.3396027347034,-1.,-1.67458429426086));
#32421=CARTESIAN_POINT('Ctrl Pts',(1.3396027347034,1.,-1.67458429426086));
#32422=CARTESIAN_POINT('Ctrl Pts',(1.34067485185203,-1.,-1.68086176030362));
#32423=CARTESIAN_POINT('Ctrl Pts',(1.34067485185203,1.,-1.68086176030362));
#32424=CARTESIAN_POINT('Ctrl Pts',(1.341710374848,-1.,-1.68715660868764));
#32425=CARTESIAN_POINT('Ctrl Pts',(1.341710374848,1.,-1.68715660868764));
#32426=CARTESIAN_POINT('Ctrl Pts',(1.34270948206319,-1.,-1.6934684849687));
#32427=CARTESIAN_POINT('Ctrl Pts',(1.34270948206319,1.,-1.6934684849687));
#32428=CARTESIAN_POINT('Ctrl Pts',(1.34367237124483,-1.,-1.69979707754427));
#32429=CARTESIAN_POINT('Ctrl Pts',(1.34367237124483,1.,-1.69979707754427));
#32430=CARTESIAN_POINT('Ctrl Pts',(1.34459924533831,-1.,-1.70614212266738));
#32431=CARTESIAN_POINT('Ctrl Pts',(1.34459924533831,1.,-1.70614212266738));
#32432=CARTESIAN_POINT('Ctrl Pts',(1.34549029589416,-1.,-1.71250340686822));
#32433=CARTESIAN_POINT('Ctrl Pts',(1.34549029589416,1.,-1.71250340686822));
#32434=CARTESIAN_POINT('Ctrl Pts',(1.34634568653227,-1.,-1.7188807715049));
#32435=CARTESIAN_POINT('Ctrl Pts',(1.34634568653227,1.,-1.7188807715049));
#32436=CARTESIAN_POINT('Ctrl Pts',(1.34716554819527,-1.,-1.72527410680674));
#32437=CARTESIAN_POINT('Ctrl Pts',(1.34716554819527,1.,-1.72527410680674));
#32438=CARTESIAN_POINT('Ctrl Pts',(1.34779309152035,-1.,-1.7304014965394));
#32439=CARTESIAN_POINT('Ctrl Pts',(1.34779309152035,1.,-1.7304014965394));
#32440=CARTESIAN_POINT('Ctrl Pts',(1.34824783112887,-1.,-1.73425417885907));
#32441=CARTESIAN_POINT('Ctrl Pts',(1.34824783112887,1.,-1.73425417885907));
#32442=CARTESIAN_POINT('Ctrl Pts',(1.34854391898045,-1.,-1.73682580585691));
#32443=CARTESIAN_POINT('Ctrl Pts',(1.34854391898045,1.,-1.73682580585691));
#32444=CARTESIAN_POINT('Ctrl Pts',(1.34869019493419,-1.,-1.73811241238545));
#32445=CARTESIAN_POINT('Ctrl Pts',(1.34869019493419,1.,-1.73811241238545));
#32446=CARTESIAN_POINT('',(1.15624053661742,1.,-1.31362392696032));
#32447=CARTESIAN_POINT('Ctrl Pts',(1.15624053661742,1.,-1.31362392696032));
#32448=CARTESIAN_POINT('Ctrl Pts',(1.15950888730809,1.,-1.31722977216397));
#32449=CARTESIAN_POINT('Ctrl Pts',(1.16589330093588,1.,-1.32428080721772));
#32450=CARTESIAN_POINT('Ctrl Pts',(1.17501305789857,1.,-1.33437539347008));
#32451=CARTESIAN_POINT('Ctrl Pts',(1.18625865667441,1.,-1.34687054001093));
#32452=CARTESIAN_POINT('Ctrl Pts',(1.1987959077932,1.,-1.36088705043885));
#32453=CARTESIAN_POINT('Ctrl Pts',(1.20982812925645,1.,-1.37331915607905));
#32454=CARTESIAN_POINT('Ctrl Pts',(1.21938737280852,1.,-1.38420564527715));
#32455=CARTESIAN_POINT('Ctrl Pts',(1.22752961899387,1.,-1.39361389568796));
#32456=CARTESIAN_POINT('Ctrl Pts',(1.23434087290423,1.,-1.40164708206106));
#32457=CARTESIAN_POINT('Ctrl Pts',(1.23994455029534,1.,-1.40845295531283));
#32458=CARTESIAN_POINT('Ctrl Pts',(1.24450600513056,1.,-1.41422913175179));
#32459=CARTESIAN_POINT('Ctrl Pts',(1.24824430986571,1.,-1.41923722596025));
#32460=CARTESIAN_POINT('Ctrl Pts',(1.2514145557001,1.,-1.42378102115575));
#32461=CARTESIAN_POINT('Ctrl Pts',(1.25426945222639,1.,-1.42815938799387));
#32462=CARTESIAN_POINT('Ctrl Pts',(1.25702687965755,1.,-1.43262645609691));
#32463=CARTESIAN_POINT('Ctrl Pts',(1.25983531012005,1.,-1.43734919180848));
#32464=CARTESIAN_POINT('Ctrl Pts',(1.26273903323858,1.,-1.44236470511303));
#32465=CARTESIAN_POINT('Ctrl Pts',(1.26570925118868,1.,-1.44761985001662));
#32466=CARTESIAN_POINT('Ctrl Pts',(1.2686778680489,1.,-1.45301422764247));
#32467=CARTESIAN_POINT('Ctrl Pts',(1.27156805265289,1.,-1.45843906294697));
#32468=CARTESIAN_POINT('Ctrl Pts',(1.27433119897822,1.,-1.46382431332476));
#32469=CARTESIAN_POINT('Ctrl Pts',(1.27696414831089,1.,-1.46916035917133));
#32470=CARTESIAN_POINT('Ctrl Pts',(1.2794891824849,1.,-1.4744717526707));
#32471=CARTESIAN_POINT('Ctrl Pts',(1.28194158939517,1.,-1.47980070347096));
#32472=CARTESIAN_POINT('Ctrl Pts',(1.28435533880201,1.,-1.4851881711891));
#32473=CARTESIAN_POINT('Ctrl Pts',(1.2867467611644,1.,-1.4906522831278));
#32474=CARTESIAN_POINT('Ctrl Pts',(1.28911506584254,1.,-1.49618896881754));
#32475=CARTESIAN_POINT('Ctrl Pts',(1.29145022885181,1.,-1.50178230149776));
#32476=CARTESIAN_POINT('Ctrl Pts',(1.29373841372842,1.,-1.50741159078365));
#32477=CARTESIAN_POINT('Ctrl Pts',(1.29596850710509,1.,-1.51305994241402));
#32478=CARTESIAN_POINT('Ctrl Pts',(1.29813791800747,1.,-1.51872184912724));
#32479=CARTESIAN_POINT('Ctrl Pts',(1.30024984366328,1.,-1.52439957861062));
#32480=CARTESIAN_POINT('Ctrl Pts',(1.30231064395568,1.,-1.53009970283891));
#32481=CARTESIAN_POINT('Ctrl Pts',(1.30432735639489,1.,-1.53582981268977));
#32482=CARTESIAN_POINT('Ctrl Pts',(1.30630475189556,1.,-1.54159462645432));
#32483=CARTESIAN_POINT('Ctrl Pts',(1.30824393907473,1.,-1.54739413957185));
#32484=CARTESIAN_POINT('Ctrl Pts',(1.31014393684222,1.,-1.55322568759481));
#32485=CARTESIAN_POINT('Ctrl Pts',(1.31200264341696,1.,-1.55908521254821));
#32486=CARTESIAN_POINT('Ctrl Pts',(1.31381795281002,1.,-1.56496872402353));
#32487=CARTESIAN_POINT('Ctrl Pts',(1.31558903860016,1.,-1.57087397835723));
#32488=CARTESIAN_POINT('Ctrl Pts',(1.31731642317187,1.,-1.5768005650559));
#32489=CARTESIAN_POINT('Ctrl Pts',(1.31900135021432,1.,-1.58274907898834));
#32490=CARTESIAN_POINT('Ctrl Pts',(1.32064537110892,1.,-1.58872057258245));
#32491=CARTESIAN_POINT('Ctrl Pts',(1.32224985747682,1.,-1.59471591079403));
#32492=CARTESIAN_POINT('Ctrl Pts',(1.32381550858256,1.,-1.60073511858687));
#32493=CARTESIAN_POINT('Ctrl Pts',(1.32534250785782,1.,-1.60677758290954));
#32494=CARTESIAN_POINT('Ctrl Pts',(1.32683074483356,1.,-1.6128423401575));
#32495=CARTESIAN_POINT('Ctrl Pts',(1.32828000610449,1.,-1.61892832270724));
#32496=CARTESIAN_POINT('Ctrl Pts',(1.3296901950568,1.,-1.62503464209797));
#32497=CARTESIAN_POINT('Ctrl Pts',(1.33106149345645,1.,-1.63116079730923));
#32498=CARTESIAN_POINT('Ctrl Pts',(1.33239425103724,1.,-1.63730653475089));
#32499=CARTESIAN_POINT('Ctrl Pts',(1.33368890676572,1.,-1.6434717485603));
#32500=CARTESIAN_POINT('Ctrl Pts',(1.33494590467993,1.,-1.6496563728683));
#32501=CARTESIAN_POINT('Ctrl Pts',(1.33616559745172,1.,-1.65586025952593));
#32502=CARTESIAN_POINT('Ctrl Pts',(1.33734820885262,1.,-1.66208312541983));
#32503=CARTESIAN_POINT('Ctrl Pts',(1.33849388654388,1.,-1.66832460783989));
#32504=CARTESIAN_POINT('Ctrl Pts',(1.3396027347034,1.,-1.67458429426086));
#32505=CARTESIAN_POINT('Ctrl Pts',(1.34067485185203,1.,-1.68086176030362));
#32506=CARTESIAN_POINT('Ctrl Pts',(1.341710374848,1.,-1.68715660868764));
#32507=CARTESIAN_POINT('Ctrl Pts',(1.34270948206319,1.,-1.6934684849687));
#32508=CARTESIAN_POINT('Ctrl Pts',(1.34367237124483,1.,-1.69979707754427));
#32509=CARTESIAN_POINT('Ctrl Pts',(1.34459924533831,1.,-1.70614212266738));
#32510=CARTESIAN_POINT('Ctrl Pts',(1.34549029589416,1.,-1.71250340686822));
#32511=CARTESIAN_POINT('Ctrl Pts',(1.34634568653227,1.,-1.7188807715049));
#32512=CARTESIAN_POINT('Ctrl Pts',(1.34716554819527,1.,-1.72527410680674));
#32513=CARTESIAN_POINT('Ctrl Pts',(1.34779309152035,1.,-1.7304014965394));
#32514=CARTESIAN_POINT('Ctrl Pts',(1.34824783112887,1.,-1.73425417885907));
#32515=CARTESIAN_POINT('Ctrl Pts',(1.34854391898045,1.,-1.73682580585691));
#32516=CARTESIAN_POINT('Ctrl Pts',(1.34869019493419,1.,-1.73811241238545));
#32517=CARTESIAN_POINT('',(1.15624053661742,0.,-1.31362392696032));
#32518=CARTESIAN_POINT('Origin',(0.,0.,0.));
#32519=CARTESIAN_POINT('',(1.31362392696032,1.,-1.15624053661742));
#32520=CARTESIAN_POINT('Origin',(0.,1.,0.));
#32521=CARTESIAN_POINT('',(1.31362392696032,0.,-1.15624053661742));
#32522=CARTESIAN_POINT('Ctrl Pts',(1.73811241238545,-1.,-1.34869019493419));
#32523=CARTESIAN_POINT('Ctrl Pts',(1.73811241238545,1.,-1.34869019493419));
#32524=CARTESIAN_POINT('Ctrl Pts',(1.73682580585819,-1.,-1.34854391898145));
#32525=CARTESIAN_POINT('Ctrl Pts',(1.73682580585819,1.,-1.34854391898145));
#32526=CARTESIAN_POINT('Ctrl Pts',(1.73425417886254,-1.,-1.34824783113158));
#32527=CARTESIAN_POINT('Ctrl Pts',(1.73425417886254,1.,-1.34824783113158));
#32528=CARTESIAN_POINT('Ctrl Pts',(1.73040149654497,-1.,-1.3477930915247));
#32529=CARTESIAN_POINT('Ctrl Pts',(1.73040149654497,1.,-1.3477930915247));
#32530=CARTESIAN_POINT('Ctrl Pts',(1.72527410681298,-1.,-1.34716554820013));
#32531=CARTESIAN_POINT('Ctrl Pts',(1.72527410681298,1.,-1.34716554820013));
#32532=CARTESIAN_POINT('Ctrl Pts',(1.7188807715095,-1.,-1.34634568653586));
#32533=CARTESIAN_POINT('Ctrl Pts',(1.7188807715095,1.,-1.34634568653586));
#32534=CARTESIAN_POINT('Ctrl Pts',(1.71250340687011,-1.,-1.34549029589563));
#32535=CARTESIAN_POINT('Ctrl Pts',(1.71250340687011,1.,-1.34549029589563));
#32536=CARTESIAN_POINT('Ctrl Pts',(1.70614212266676,-1.,-1.34459924533783));
#32537=CARTESIAN_POINT('Ctrl Pts',(1.70614212266676,1.,-1.34459924533783));
#32538=CARTESIAN_POINT('Ctrl Pts',(1.69979707754221,-1.,-1.34367237124322));
#32539=CARTESIAN_POINT('Ctrl Pts',(1.69979707754221,1.,-1.34367237124322));
#32540=CARTESIAN_POINT('Ctrl Pts',(1.6934684849664,-1.,-1.34270948206139));
#32541=CARTESIAN_POINT('Ctrl Pts',(1.6934684849664,1.,-1.34270948206139));
#32542=CARTESIAN_POINT('Ctrl Pts',(1.68715660868602,-1.,-1.34171037484673));
#32543=CARTESIAN_POINT('Ctrl Pts',(1.68715660868602,1.,-1.34171037484673));
#32544=CARTESIAN_POINT('Ctrl Pts',(1.68086176030308,-1.,-1.3406748518516));
#32545=CARTESIAN_POINT('Ctrl Pts',(1.68086176030308,1.,-1.3406748518516));
#32546=CARTESIAN_POINT('Ctrl Pts',(1.67458429426126,-1.,-1.33960273470372));
#32547=CARTESIAN_POINT('Ctrl Pts',(1.67458429426126,1.,-1.33960273470372));
#32548=CARTESIAN_POINT('Ctrl Pts',(1.66832460784078,-1.,-1.33849388654458));
#32549=CARTESIAN_POINT('Ctrl Pts',(1.66832460784078,1.,-1.33849388654458));
#32550=CARTESIAN_POINT('Ctrl Pts',(1.66208312542073,-1.,-1.33734820885331));
#32551=CARTESIAN_POINT('Ctrl Pts',(1.66208312542073,1.,-1.33734820885331));
#32552=CARTESIAN_POINT('Ctrl Pts',(1.65586025952651,-1.,-1.33616559745217));
#32553=CARTESIAN_POINT('Ctrl Pts',(1.65586025952651,1.,-1.33616559745217));
#32554=CARTESIAN_POINT('Ctrl Pts',(1.64965637286843,-1.,-1.33494590468003));
#32555=CARTESIAN_POINT('Ctrl Pts',(1.64965637286843,1.,-1.33494590468003));
#32556=CARTESIAN_POINT('Ctrl Pts',(1.64347174856007,-1.,-1.33368890676554));
#32557=CARTESIAN_POINT('Ctrl Pts',(1.64347174856007,1.,-1.33368890676554));
#32558=CARTESIAN_POINT('Ctrl Pts',(1.63730653475049,-1.,-1.33239425103694));
#32559=CARTESIAN_POINT('Ctrl Pts',(1.63730653475049,1.,-1.33239425103694));
#32560=CARTESIAN_POINT('Ctrl Pts',(1.63116079730887,-1.,-1.33106149345618));
#32561=CARTESIAN_POINT('Ctrl Pts',(1.63116079730887,1.,-1.33106149345618));
#32562=CARTESIAN_POINT('Ctrl Pts',(1.62503464209777,-1.,-1.32969019505665));
#32563=CARTESIAN_POINT('Ctrl Pts',(1.62503464209777,1.,-1.32969019505665));
#32564=CARTESIAN_POINT('Ctrl Pts',(1.61892832270723,-1.,-1.32828000610448));
#32565=CARTESIAN_POINT('Ctrl Pts',(1.61892832270723,1.,-1.32828000610448));
#32566=CARTESIAN_POINT('Ctrl Pts',(1.61284234015762,-1.,-1.32683074483365));
#32567=CARTESIAN_POINT('Ctrl Pts',(1.61284234015762,1.,-1.32683074483365));
#32568=CARTESIAN_POINT('Ctrl Pts',(1.6067775829097,-1.,-1.32534250785794));
#32569=CARTESIAN_POINT('Ctrl Pts',(1.6067775829097,1.,-1.32534250785794));
#32570=CARTESIAN_POINT('Ctrl Pts',(1.600735118587,-1.,-1.32381550858266));
#32571=CARTESIAN_POINT('Ctrl Pts',(1.600735118587,1.,-1.32381550858266));
#32572=CARTESIAN_POINT('Ctrl Pts',(1.59471591079408,-1.,-1.32224985747686));
#32573=CARTESIAN_POINT('Ctrl Pts',(1.59471591079408,1.,-1.32224985747686));
#32574=CARTESIAN_POINT('Ctrl Pts',(1.58872057258244,-1.,-1.32064537110891));
#32575=CARTESIAN_POINT('Ctrl Pts',(1.58872057258244,1.,-1.32064537110891));
#32576=CARTESIAN_POINT('Ctrl Pts',(1.58274907898829,-1.,-1.31900135021428));
#32577=CARTESIAN_POINT('Ctrl Pts',(1.58274907898829,1.,-1.31900135021428));
#32578=CARTESIAN_POINT('Ctrl Pts',(1.57680056505585,-1.,-1.31731642317183));
#32579=CARTESIAN_POINT('Ctrl Pts',(1.57680056505585,1.,-1.31731642317183));
#32580=CARTESIAN_POINT('Ctrl Pts',(1.57087397835721,-1.,-1.31558903860015));
#32581=CARTESIAN_POINT('Ctrl Pts',(1.57087397835721,1.,-1.31558903860015));
#32582=CARTESIAN_POINT('Ctrl Pts',(1.56496872402352,-1.,-1.31381795281002));
#32583=CARTESIAN_POINT('Ctrl Pts',(1.56496872402352,1.,-1.31381795281002));
#32584=CARTESIAN_POINT('Ctrl Pts',(1.55908521254822,-1.,-1.31200264341696));
#32585=CARTESIAN_POINT('Ctrl Pts',(1.55908521254822,1.,-1.31200264341696));
#32586=CARTESIAN_POINT('Ctrl Pts',(1.55322568759481,-1.,-1.31014393684221));
#32587=CARTESIAN_POINT('Ctrl Pts',(1.55322568759481,1.,-1.31014393684221));
#32588=CARTESIAN_POINT('Ctrl Pts',(1.54739413957183,-1.,-1.30824393907471));
#32589=CARTESIAN_POINT('Ctrl Pts',(1.54739413957183,1.,-1.30824393907471));
#32590=CARTESIAN_POINT('Ctrl Pts',(1.54159462645428,-1.,-1.30630475189553));
#32591=CARTESIAN_POINT('Ctrl Pts',(1.54159462645428,1.,-1.30630475189553));
#32592=CARTESIAN_POINT('Ctrl Pts',(1.53582981268976,-1.,-1.30432735639487));
#32593=CARTESIAN_POINT('Ctrl Pts',(1.53582981268976,1.,-1.30432735639487));
#32594=CARTESIAN_POINT('Ctrl Pts',(1.53009970283893,-1.,-1.3023106439557));
#32595=CARTESIAN_POINT('Ctrl Pts',(1.53009970283893,1.,-1.3023106439557));
#32596=CARTESIAN_POINT('Ctrl Pts',(1.5243995786107,-1.,-1.30024984366334));
#32597=CARTESIAN_POINT('Ctrl Pts',(1.5243995786107,1.,-1.30024984366334));
#32598=CARTESIAN_POINT('Ctrl Pts',(1.51872184912735,-1.,-1.29813791800757));
#32599=CARTESIAN_POINT('Ctrl Pts',(1.51872184912735,1.,-1.29813791800757));
#32600=CARTESIAN_POINT('Ctrl Pts',(1.51305994241412,-1.,-1.29596850710518));
#32601=CARTESIAN_POINT('Ctrl Pts',(1.51305994241412,1.,-1.29596850710518));
#32602=CARTESIAN_POINT('Ctrl Pts',(1.50741159078367,-1.,-1.29373841372843));
#32603=CARTESIAN_POINT('Ctrl Pts',(1.50741159078367,1.,-1.29373841372843));
#32604=CARTESIAN_POINT('Ctrl Pts',(1.50178230149764,-1.,-1.29145022885171));
#32605=CARTESIAN_POINT('Ctrl Pts',(1.50178230149764,1.,-1.29145022885171));
#32606=CARTESIAN_POINT('Ctrl Pts',(1.49618896881729,-1.,-1.28911506584232));
#32607=CARTESIAN_POINT('Ctrl Pts',(1.49618896881729,1.,-1.28911506584232));
#32608=CARTESIAN_POINT('Ctrl Pts',(1.4906522831275,-1.,-1.28674676116415));
#32609=CARTESIAN_POINT('Ctrl Pts',(1.4906522831275,1.,-1.28674676116415));
#32610=CARTESIAN_POINT('Ctrl Pts',(1.48518817118891,-1.,-1.28435533880184));
#32611=CARTESIAN_POINT('Ctrl Pts',(1.48518817118891,1.,-1.28435533880184));
#32612=CARTESIAN_POINT('Ctrl Pts',(1.47980070347102,-1.,-1.28194158939522));
#32613=CARTESIAN_POINT('Ctrl Pts',(1.47980070347102,1.,-1.28194158939522));
#32614=CARTESIAN_POINT('Ctrl Pts',(1.4744717526711,-1.,-1.27948918248524));
#32615=CARTESIAN_POINT('Ctrl Pts',(1.4744717526711,1.,-1.27948918248524));
#32616=CARTESIAN_POINT('Ctrl Pts',(1.46916035917197,-1.,-1.27696414831144));
#32617=CARTESIAN_POINT('Ctrl Pts',(1.46916035917197,1.,-1.27696414831144));
#32618=CARTESIAN_POINT('Ctrl Pts',(1.4638243133254,-1.,-1.27433119897877));
#32619=CARTESIAN_POINT('Ctrl Pts',(1.4638243133254,1.,-1.27433119897877));
#32620=CARTESIAN_POINT('Ctrl Pts',(1.45843906294725,-1.,-1.27156805265312));
#32621=CARTESIAN_POINT('Ctrl Pts',(1.45843906294725,1.,-1.27156805265312));
#32622=CARTESIAN_POINT('Ctrl Pts',(1.45301422764205,-1.,-1.26867786804854));
#32623=CARTESIAN_POINT('Ctrl Pts',(1.45301422764205,1.,-1.26867786804854));
#32624=CARTESIAN_POINT('Ctrl Pts',(1.44761985001544,-1.,-1.26570925118767));
#32625=CARTESIAN_POINT('Ctrl Pts',(1.44761985001544,1.,-1.26570925118767));
#32626=CARTESIAN_POINT('Ctrl Pts',(1.44236470511145,-1.,-1.26273903323723));
#32627=CARTESIAN_POINT('Ctrl Pts',(1.44236470511145,1.,-1.26273903323723));
#32628=CARTESIAN_POINT('Ctrl Pts',(1.43734919180719,-1.,-1.25983531011894));
#32629=CARTESIAN_POINT('Ctrl Pts',(1.43734919180719,1.,-1.25983531011894));
#32630=CARTESIAN_POINT('Ctrl Pts',(1.43262645609679,-1.,-1.25702687965744));
#32631=CARTESIAN_POINT('Ctrl Pts',(1.43262645609679,1.,-1.25702687965744));
#32632=CARTESIAN_POINT('Ctrl Pts',(1.42815938799555,-1.,-1.25426945222783));
#32633=CARTESIAN_POINT('Ctrl Pts',(1.42815938799555,1.,-1.25426945222783));
#32634=CARTESIAN_POINT('Ctrl Pts',(1.42378102115911,-1.,-1.25141455570299));
#32635=CARTESIAN_POINT('Ctrl Pts',(1.42378102115911,1.,-1.25141455570299));
#32636=CARTESIAN_POINT('Ctrl Pts',(1.41923722596421,-1.,-1.24824430986911));
#32637=CARTESIAN_POINT('Ctrl Pts',(1.41923722596421,1.,-1.24824430986911));
#32638=CARTESIAN_POINT('Ctrl Pts',(1.41422913175437,-1.,-1.24450600513278));
#32639=CARTESIAN_POINT('Ctrl Pts',(1.41422913175437,1.,-1.24450600513278));
#32640=CARTESIAN_POINT('Ctrl Pts',(1.40845295531151,-1.,-1.23994455029421));
#32641=CARTESIAN_POINT('Ctrl Pts',(1.40845295531151,1.,-1.23994455029421));
#32642=CARTESIAN_POINT('Ctrl Pts',(1.40164708205345,-1.,-1.23434087289768));
#32643=CARTESIAN_POINT('Ctrl Pts',(1.40164708205345,1.,-1.23434087289768));
#32644=CARTESIAN_POINT('Ctrl Pts',(1.39361389567257,-1.,-1.22752961898063));
#32645=CARTESIAN_POINT('Ctrl Pts',(1.39361389567257,1.,-1.22752961898063));
#32646=CARTESIAN_POINT('Ctrl Pts',(1.38420564525391,-1.,-1.21938737278853));
#32647=CARTESIAN_POINT('Ctrl Pts',(1.38420564525391,1.,-1.21938737278853));
#32648=CARTESIAN_POINT('Ctrl Pts',(1.37331915604962,-1.,-1.20982812923113));
#32649=CARTESIAN_POINT('Ctrl Pts',(1.37331915604962,1.,-1.20982812923113));
#32650=CARTESIAN_POINT('Ctrl Pts',(1.36088705040677,-1.,-1.1987959077656));
#32651=CARTESIAN_POINT('Ctrl Pts',(1.36088705040677,1.,-1.1987959077656));
#32652=CARTESIAN_POINT('Ctrl Pts',(1.34687053998157,-1.,-1.18625865664915));
#32653=CARTESIAN_POINT('Ctrl Pts',(1.34687053998157,1.,-1.18625865664915));
#32654=CARTESIAN_POINT('Ctrl Pts',(1.33437539344842,-1.,-1.17501305787994));
#32655=CARTESIAN_POINT('Ctrl Pts',(1.33437539344842,1.,-1.17501305787994));
#32656=CARTESIAN_POINT('Ctrl Pts',(1.32428080720544,-1.,-1.16589330092532));
#32657=CARTESIAN_POINT('Ctrl Pts',(1.32428080720544,1.,-1.16589330092532));
#32658=CARTESIAN_POINT('Ctrl Pts',(1.3172297721596,-1.,-1.15950888730433));
#32659=CARTESIAN_POINT('Ctrl Pts',(1.3172297721596,1.,-1.15950888730433));
#32660=CARTESIAN_POINT('Ctrl Pts',(1.31362392696032,-1.,-1.15624053661742));
#32661=CARTESIAN_POINT('Ctrl Pts',(1.31362392696032,1.,-1.15624053661742));
#32662=CARTESIAN_POINT('',(1.73811241238545,1.,-1.34869019493419));
#32663=CARTESIAN_POINT('Ctrl Pts',(1.73811241238545,1.,-1.34869019493419));
#32664=CARTESIAN_POINT('Ctrl Pts',(1.73682580585819,1.,-1.34854391898145));
#32665=CARTESIAN_POINT('Ctrl Pts',(1.73425417886254,1.,-1.34824783113158));
#32666=CARTESIAN_POINT('Ctrl Pts',(1.73040149654497,1.,-1.3477930915247));
#32667=CARTESIAN_POINT('Ctrl Pts',(1.72527410681298,1.,-1.34716554820013));
#32668=CARTESIAN_POINT('Ctrl Pts',(1.7188807715095,1.,-1.34634568653586));
#32669=CARTESIAN_POINT('Ctrl Pts',(1.71250340687011,1.,-1.34549029589563));
#32670=CARTESIAN_POINT('Ctrl Pts',(1.70614212266676,1.,-1.34459924533783));
#32671=CARTESIAN_POINT('Ctrl Pts',(1.69979707754221,1.,-1.34367237124322));
#32672=CARTESIAN_POINT('Ctrl Pts',(1.6934684849664,1.,-1.34270948206139));
#32673=CARTESIAN_POINT('Ctrl Pts',(1.68715660868602,1.,-1.34171037484673));
#32674=CARTESIAN_POINT('Ctrl Pts',(1.68086176030308,1.,-1.3406748518516));
#32675=CARTESIAN_POINT('Ctrl Pts',(1.67458429426126,1.,-1.33960273470372));
#32676=CARTESIAN_POINT('Ctrl Pts',(1.66832460784078,1.,-1.33849388654458));
#32677=CARTESIAN_POINT('Ctrl Pts',(1.66208312542073,1.,-1.33734820885331));
#32678=CARTESIAN_POINT('Ctrl Pts',(1.65586025952651,1.,-1.33616559745217));
#32679=CARTESIAN_POINT('Ctrl Pts',(1.64965637286843,1.,-1.33494590468003));
#32680=CARTESIAN_POINT('Ctrl Pts',(1.64347174856007,1.,-1.33368890676554));
#32681=CARTESIAN_POINT('Ctrl Pts',(1.63730653475049,1.,-1.33239425103694));
#32682=CARTESIAN_POINT('Ctrl Pts',(1.63116079730887,1.,-1.33106149345618));
#32683=CARTESIAN_POINT('Ctrl Pts',(1.62503464209777,1.,-1.32969019505665));
#32684=CARTESIAN_POINT('Ctrl Pts',(1.61892832270723,1.,-1.32828000610448));
#32685=CARTESIAN_POINT('Ctrl Pts',(1.61284234015762,1.,-1.32683074483365));
#32686=CARTESIAN_POINT('Ctrl Pts',(1.6067775829097,1.,-1.32534250785794));
#32687=CARTESIAN_POINT('Ctrl Pts',(1.600735118587,1.,-1.32381550858266));
#32688=CARTESIAN_POINT('Ctrl Pts',(1.59471591079408,1.,-1.32224985747686));
#32689=CARTESIAN_POINT('Ctrl Pts',(1.58872057258244,1.,-1.32064537110891));
#32690=CARTESIAN_POINT('Ctrl Pts',(1.58274907898829,1.,-1.31900135021428));
#32691=CARTESIAN_POINT('Ctrl Pts',(1.57680056505585,1.,-1.31731642317183));
#32692=CARTESIAN_POINT('Ctrl Pts',(1.57087397835721,1.,-1.31558903860015));
#32693=CARTESIAN_POINT('Ctrl Pts',(1.56496872402352,1.,-1.31381795281002));
#32694=CARTESIAN_POINT('Ctrl Pts',(1.55908521254822,1.,-1.31200264341696));
#32695=CARTESIAN_POINT('Ctrl Pts',(1.55322568759481,1.,-1.31014393684221));
#32696=CARTESIAN_POINT('Ctrl Pts',(1.54739413957183,1.,-1.30824393907471));
#32697=CARTESIAN_POINT('Ctrl Pts',(1.54159462645428,1.,-1.30630475189553));
#32698=CARTESIAN_POINT('Ctrl Pts',(1.53582981268976,1.,-1.30432735639487));
#32699=CARTESIAN_POINT('Ctrl Pts',(1.53009970283893,1.,-1.3023106439557));
#32700=CARTESIAN_POINT('Ctrl Pts',(1.5243995786107,1.,-1.30024984366334));
#32701=CARTESIAN_POINT('Ctrl Pts',(1.51872184912735,1.,-1.29813791800757));
#32702=CARTESIAN_POINT('Ctrl Pts',(1.51305994241412,1.,-1.29596850710518));
#32703=CARTESIAN_POINT('Ctrl Pts',(1.50741159078367,1.,-1.29373841372843));
#32704=CARTESIAN_POINT('Ctrl Pts',(1.50178230149764,1.,-1.29145022885171));
#32705=CARTESIAN_POINT('Ctrl Pts',(1.49618896881729,1.,-1.28911506584232));
#32706=CARTESIAN_POINT('Ctrl Pts',(1.4906522831275,1.,-1.28674676116415));
#32707=CARTESIAN_POINT('Ctrl Pts',(1.48518817118891,1.,-1.28435533880184));
#32708=CARTESIAN_POINT('Ctrl Pts',(1.47980070347102,1.,-1.28194158939522));
#32709=CARTESIAN_POINT('Ctrl Pts',(1.4744717526711,1.,-1.27948918248524));
#32710=CARTESIAN_POINT('Ctrl Pts',(1.46916035917197,1.,-1.27696414831144));
#32711=CARTESIAN_POINT('Ctrl Pts',(1.4638243133254,1.,-1.27433119897877));
#32712=CARTESIAN_POINT('Ctrl Pts',(1.45843906294725,1.,-1.27156805265312));
#32713=CARTESIAN_POINT('Ctrl Pts',(1.45301422764205,1.,-1.26867786804854));
#32714=CARTESIAN_POINT('Ctrl Pts',(1.44761985001544,1.,-1.26570925118767));
#32715=CARTESIAN_POINT('Ctrl Pts',(1.44236470511145,1.,-1.26273903323723));
#32716=CARTESIAN_POINT('Ctrl Pts',(1.43734919180719,1.,-1.25983531011894));
#32717=CARTESIAN_POINT('Ctrl Pts',(1.43262645609679,1.,-1.25702687965744));
#32718=CARTESIAN_POINT('Ctrl Pts',(1.42815938799555,1.,-1.25426945222783));
#32719=CARTESIAN_POINT('Ctrl Pts',(1.42378102115911,1.,-1.25141455570299));
#32720=CARTESIAN_POINT('Ctrl Pts',(1.41923722596421,1.,-1.24824430986911));
#32721=CARTESIAN_POINT('Ctrl Pts',(1.41422913175437,1.,-1.24450600513278));
#32722=CARTESIAN_POINT('Ctrl Pts',(1.40845295531151,1.,-1.23994455029421));
#32723=CARTESIAN_POINT('Ctrl Pts',(1.40164708205345,1.,-1.23434087289768));
#32724=CARTESIAN_POINT('Ctrl Pts',(1.39361389567257,1.,-1.22752961898063));
#32725=CARTESIAN_POINT('Ctrl Pts',(1.38420564525391,1.,-1.21938737278853));
#32726=CARTESIAN_POINT('Ctrl Pts',(1.37331915604962,1.,-1.20982812923113));
#32727=CARTESIAN_POINT('Ctrl Pts',(1.36088705040677,1.,-1.1987959077656));
#32728=CARTESIAN_POINT('Ctrl Pts',(1.34687053998157,1.,-1.18625865664915));
#32729=CARTESIAN_POINT('Ctrl Pts',(1.33437539344842,1.,-1.17501305787994));
#32730=CARTESIAN_POINT('Ctrl Pts',(1.32428080720544,1.,-1.16589330092532));
#32731=CARTESIAN_POINT('Ctrl Pts',(1.3172297721596,1.,-1.15950888730433));
#32732=CARTESIAN_POINT('Ctrl Pts',(1.31362392696032,1.,-1.15624053661742));
#32733=CARTESIAN_POINT('',(1.73811241238545,0.,-1.34869019493419));
#32734=CARTESIAN_POINT('Origin',(1.81978687191668,0.,-1.23627494547115));
#32735=CARTESIAN_POINT('',(1.81978687191668,1.,-1.23627494547115));
#32736=CARTESIAN_POINT('',(1.73811241238545,1.,-1.34869019493419));
#32737=CARTESIAN_POINT('',(1.81978687191668,0.,-1.23627494547115));
#32738=CARTESIAN_POINT('Ctrl Pts',(1.5055822144029,-1.,-0.892032620296855));
#32739=CARTESIAN_POINT('Ctrl Pts',(1.5055822144029,1.,-0.892032620296855));
#32740=CARTESIAN_POINT('Ctrl Pts',(1.50980486807181,-1.,-0.894452006967538));
#32741=CARTESIAN_POINT('Ctrl Pts',(1.50980486807181,1.,-0.894452006967538));
#32742=CARTESIAN_POINT('Ctrl Pts',(1.51805569591479,-1.,-0.89918504749193));
#32743=CARTESIAN_POINT('Ctrl Pts',(1.51805569591479,1.,-0.89918504749193));
#32744=CARTESIAN_POINT('Ctrl Pts',(1.52984849890434,-1.,-0.905967409640499));
#32745=CARTESIAN_POINT('Ctrl Pts',(1.52984849890434,1.,-0.905967409640499));
#32746=CARTESIAN_POINT('Ctrl Pts',(1.54440491152807,-1.,-0.91437591904658));
#32747=CARTESIAN_POINT('Ctrl Pts',(1.54440491152807,1.,-0.91437591904658));
#32748=CARTESIAN_POINT('Ctrl Pts',(1.56065988582509,-1.,-0.923832188966322));
#32749=CARTESIAN_POINT('Ctrl Pts',(1.56065988582509,1.,-0.923832188966322));
#32750=CARTESIAN_POINT('Ctrl Pts',(1.57499388385561,-1.,-0.932246680128849));
#32751=CARTESIAN_POINT('Ctrl Pts',(1.57499388385561,1.,-0.932246680128849));
#32752=CARTESIAN_POINT('Ctrl Pts',(1.58744937489796,-1.,-0.939646377909319));
#32753=CARTESIAN_POINT('Ctrl Pts',(1.58744937489796,1.,-0.939646377909319));
#32754=CARTESIAN_POINT('Ctrl Pts',(1.59810042045408,-1.,-0.946078063325796));
#32755=CARTESIAN_POINT('Ctrl Pts',(1.59810042045408,1.,-0.946078063325796));
#32756=CARTESIAN_POINT('Ctrl Pts',(1.60706069897794,-1.,-0.951613284361248));
#32757=CARTESIAN_POINT('Ctrl Pts',(1.60706069897794,1.,-0.951613284361248));
#32758=CARTESIAN_POINT('Ctrl Pts',(1.61449324337233,-1.,-0.956354422921573));
#32759=CARTESIAN_POINT('Ctrl Pts',(1.61449324337233,1.,-0.956354422921573));
#32760=CARTESIAN_POINT('Ctrl Pts',(1.62061638139929,-1.,-0.960438326099958));
#32761=CARTESIAN_POINT('Ctrl Pts',(1.62061638139929,1.,-0.960438326099958));
#32762=CARTESIAN_POINT('Ctrl Pts',(1.6257193066974,-1.,-0.964046107037821));
#32763=CARTESIAN_POINT('Ctrl Pts',(1.6257193066974,1.,-0.964046107037821));
#32764=CARTESIAN_POINT('Ctrl Pts',(1.63013849959083,-1.,-0.967387853228041));
#32765=CARTESIAN_POINT('Ctrl Pts',(1.63013849959083,1.,-0.967387853228041));
#32766=CARTESIAN_POINT('Ctrl Pts',(1.63420665729609,-1.,-0.970669715996356));
#32767=CARTESIAN_POINT('Ctrl Pts',(1.63420665729609,1.,-0.970669715996356));
#32768=CARTESIAN_POINT('Ctrl Pts',(1.63820952658157,-1.,-0.974066058287501));
#32769=CARTESIAN_POINT('Ctrl Pts',(1.63820952658157,1.,-0.974066058287501));
#32770=CARTESIAN_POINT('Ctrl Pts',(1.64233990826831,-1.,-0.977689794120297));
#32771=CARTESIAN_POINT('Ctrl Pts',(1.64233990826831,1.,-0.977689794120297));
#32772=CARTESIAN_POINT('Ctrl Pts',(1.64665139190834,-1.,-0.981562530940574));
#32773=CARTESIAN_POINT('Ctrl Pts',(1.64665139190834,1.,-0.981562530940574));
#32774=CARTESIAN_POINT('Ctrl Pts',(1.6511001661277,-1.,-0.985642622921626));
#32775=CARTESIAN_POINT('Ctrl Pts',(1.6511001661277,1.,-0.985642622921626));
#32776=CARTESIAN_POINT('Ctrl Pts',(1.65559044289746,-1.,-0.98985562785445));
#32777=CARTESIAN_POINT('Ctrl Pts',(1.65559044289746,1.,-0.98985562785445));
#32778=CARTESIAN_POINT('Ctrl Pts',(1.66001553809916,-1.,-0.994121836661116));
#32779=CARTESIAN_POINT('Ctrl Pts',(1.66001553809916,1.,-0.994121836661116));
#32780=CARTESIAN_POINT('Ctrl Pts',(1.66430758030304,-1.,-0.998389654952317));
#32781=CARTESIAN_POINT('Ctrl Pts',(1.66430758030304,1.,-0.998389654952317));
#32782=CARTESIAN_POINT('Ctrl Pts',(1.66846059277231,-1.,-1.00265091003682));
#32783=CARTESIAN_POINT('Ctrl Pts',(1.66846059277231,1.,-1.00265091003682));
#32784=CARTESIAN_POINT('Ctrl Pts',(1.67250335383248,-1.,-1.00692206696387));
#32785=CARTESIAN_POINT('Ctrl Pts',(1.67250335383248,1.,-1.00692206696387));
#32786=CARTESIAN_POINT('Ctrl Pts',(1.67648246776457,-1.,-1.01123236493507));
#32787=CARTESIAN_POINT('Ctrl Pts',(1.67648246776457,1.,-1.01123236493507));
#32788=CARTESIAN_POINT('Ctrl Pts',(1.6804428989482,-1.,-1.01561026162787));
#32789=CARTESIAN_POINT('Ctrl Pts',(1.6804428989482,1.,-1.01561026162787));
#32790=CARTESIAN_POINT('Ctrl Pts',(1.68440578021739,-1.,-1.02006795074222));
#32791=CARTESIAN_POINT('Ctrl Pts',(1.68440578021739,1.,-1.02006795074222));
#32792=CARTESIAN_POINT('Ctrl Pts',(1.68836910178475,-1.,-1.02460180535272));
#32793=CARTESIAN_POINT('Ctrl Pts',(1.68836910178475,1.,-1.02460180535272));
#32794=CARTESIAN_POINT('Ctrl Pts',(1.69231840863471,-1.,-1.02919977579155));
#32795=CARTESIAN_POINT('Ctrl Pts',(1.69231840863471,1.,-1.02919977579155));
#32796=CARTESIAN_POINT('Ctrl Pts',(1.69623414782769,-1.,-1.03384646003587));
#32797=CARTESIAN_POINT('Ctrl Pts',(1.69623414782769,1.,-1.03384646003587));
#32798=CARTESIAN_POINT('Ctrl Pts',(1.70010052930951,-1.,-1.03852922490782));
#32799=CARTESIAN_POINT('Ctrl Pts',(1.70010052930951,1.,-1.03852922490782));
#32800=CARTESIAN_POINT('Ctrl Pts',(1.70391338707969,-1.,-1.04324363334546));
#32801=CARTESIAN_POINT('Ctrl Pts',(1.70391338707969,1.,-1.04324363334546));
#32802=CARTESIAN_POINT('Ctrl Pts',(1.70767646263641,-1.,-1.0479908540499));
#32803=CARTESIAN_POINT('Ctrl Pts',(1.70767646263641,1.,-1.0479908540499));
#32804=CARTESIAN_POINT('Ctrl Pts',(1.71139783543986,-1.,-1.05277517202854));
#32805=CARTESIAN_POINT('Ctrl Pts',(1.71139783543986,1.,-1.05277517202854));
#32806=CARTESIAN_POINT('Ctrl Pts',(1.71508654427022,-1.,-1.05760163192481));
#32807=CARTESIAN_POINT('Ctrl Pts',(1.71508654427022,1.,-1.05760163192481));
#32808=CARTESIAN_POINT('Ctrl Pts',(1.71874858456908,-1.,-1.0624732468065));
#32809=CARTESIAN_POINT('Ctrl Pts',(1.71874858456908,1.,-1.0624732468065));
#32810=CARTESIAN_POINT('Ctrl Pts',(1.72238500928456,-1.,-1.06738966975463));
#32811=CARTESIAN_POINT('Ctrl Pts',(1.72238500928456,1.,-1.06738966975463));
#32812=CARTESIAN_POINT('Ctrl Pts',(1.72599406198489,-1.,-1.07234866990252));
#32813=CARTESIAN_POINT('Ctrl Pts',(1.72599406198489,1.,-1.07234866990252));
#32814=CARTESIAN_POINT('Ctrl Pts',(1.72957248977424,-1.,-1.0773470373727));
#32815=CARTESIAN_POINT('Ctrl Pts',(1.72957248977424,1.,-1.0773470373727));
#32816=CARTESIAN_POINT('Ctrl Pts',(1.73311705663407,-1.,-1.08238162784749));
#32817=CARTESIAN_POINT('Ctrl Pts',(1.73311705663407,1.,-1.08238162784749));
#32818=CARTESIAN_POINT('Ctrl Pts',(1.73662628326093,-1.,-1.08745056285429));
#32819=CARTESIAN_POINT('Ctrl Pts',(1.73662628326093,1.,-1.08745056285429));
#32820=CARTESIAN_POINT('Ctrl Pts',(1.74010053962252,-1.,-1.09255329056496));
#32821=CARTESIAN_POINT('Ctrl Pts',(1.74010053962252,1.,-1.09255329056496));
#32822=CARTESIAN_POINT('Ctrl Pts',(1.74354119236212,-1.,-1.09768999241229));
#32823=CARTESIAN_POINT('Ctrl Pts',(1.74354119236212,1.,-1.09768999241229));
#32824=CARTESIAN_POINT('Ctrl Pts',(1.74695004214924,-1.,-1.10286118991144));
#32825=CARTESIAN_POINT('Ctrl Pts',(1.74695004214924,1.,-1.10286118991144));
#32826=CARTESIAN_POINT('Ctrl Pts',(1.75032866075914,-1.,-1.10806728183003));
#32827=CARTESIAN_POINT('Ctrl Pts',(1.75032866075914,1.,-1.10806728183003));
#32828=CARTESIAN_POINT('Ctrl Pts',(1.75367772094617,-1.,-1.11330807582542));
#32829=CARTESIAN_POINT('Ctrl Pts',(1.75367772094617,1.,-1.11330807582542));
#32830=CARTESIAN_POINT('Ctrl Pts',(1.75699720772089,-1.,-1.11858293216752));
#32831=CARTESIAN_POINT('Ctrl Pts',(1.75699720772089,1.,-1.11858293216752));
#32832=CARTESIAN_POINT('Ctrl Pts',(1.76028671825084,-1.,-1.12389096855078));
#32833=CARTESIAN_POINT('Ctrl Pts',(1.76028671825084,1.,-1.12389096855078));
#32834=CARTESIAN_POINT('Ctrl Pts',(1.76354571966171,-1.,-1.12923123555076));
#32835=CARTESIAN_POINT('Ctrl Pts',(1.76354571966171,1.,-1.12923123555076));
#32836=CARTESIAN_POINT('Ctrl Pts',(1.76677384551883,-1.,-1.13460291804635));
#32837=CARTESIAN_POINT('Ctrl Pts',(1.76677384551883,1.,-1.13460291804635));
#32838=CARTESIAN_POINT('Ctrl Pts',(1.76997111386806,-1.,-1.14000548337));
#32839=CARTESIAN_POINT('Ctrl Pts',(1.76997111386806,1.,-1.14000548337));
#32840=CARTESIAN_POINT('Ctrl Pts',(1.77313777896234,-1.,-1.14543858226948));
#32841=CARTESIAN_POINT('Ctrl Pts',(1.77313777896234,1.,-1.14543858226948));
#32842=CARTESIAN_POINT('Ctrl Pts',(1.77627422557034,-1.,-1.15090197841531));
#32843=CARTESIAN_POINT('Ctrl Pts',(1.77627422557034,1.,-1.15090197841531));
#32844=CARTESIAN_POINT('Ctrl Pts',(1.77938085564261,-1.,-1.15639547194689));
#32845=CARTESIAN_POINT('Ctrl Pts',(1.77938085564261,1.,-1.15639547194689));
#32846=CARTESIAN_POINT('Ctrl Pts',(1.78245795880949,-1.,-1.16191881298458));
#32847=CARTESIAN_POINT('Ctrl Pts',(1.78245795880949,1.,-1.16191881298458));
#32848=CARTESIAN_POINT('Ctrl Pts',(1.78550566040349,-1.,-1.16747166312239));
#32849=CARTESIAN_POINT('Ctrl Pts',(1.78550566040349,1.,-1.16747166312239));
#32850=CARTESIAN_POINT('Ctrl Pts',(1.78852398877523,-1.,-1.17305363177265));
#32851=CARTESIAN_POINT('Ctrl Pts',(1.78852398877523,1.,-1.17305363177265));
#32852=CARTESIAN_POINT('Ctrl Pts',(1.79151291552646,-1.,-1.17866429440781));
#32853=CARTESIAN_POINT('Ctrl Pts',(1.79151291552646,1.,-1.17866429440781));
#32854=CARTESIAN_POINT('Ctrl Pts',(1.79447240321572,-1.,-1.18430321697471));
#32855=CARTESIAN_POINT('Ctrl Pts',(1.79447240321572,1.,-1.18430321697471));
#32856=CARTESIAN_POINT('Ctrl Pts',(1.79740245923649,-1.,-1.1899699793456));
#32857=CARTESIAN_POINT('Ctrl Pts',(1.79740245923649,1.,-1.1899699793456));
#32858=CARTESIAN_POINT('Ctrl Pts',(1.80030314370121,-1.,-1.19566418930405));
#32859=CARTESIAN_POINT('Ctrl Pts',(1.80030314370121,1.,-1.19566418930405));
#32860=CARTESIAN_POINT('Ctrl Pts',(1.8031745483882,-1.,-1.2013854893912));
#32861=CARTESIAN_POINT('Ctrl Pts',(1.8031745483882,1.,-1.2013854893912));
#32862=CARTESIAN_POINT('Ctrl Pts',(1.80601678480772,-1.,-1.20713356605519));
#32863=CARTESIAN_POINT('Ctrl Pts',(1.80601678480772,1.,-1.20713356605519));
#32864=CARTESIAN_POINT('Ctrl Pts',(1.80882996916931,-1.,-1.2129081570818));
#32865=CARTESIAN_POINT('Ctrl Pts',(1.80882996916931,1.,-1.2129081570818));
#32866=CARTESIAN_POINT('Ctrl Pts',(1.81161420806172,-1.,-1.2187090610323));
#32867=CARTESIAN_POINT('Ctrl Pts',(1.81161420806172,1.,-1.2187090610323));
#32868=CARTESIAN_POINT('Ctrl Pts',(1.81436959209778,-1.,-1.22453613304507));
#32869=CARTESIAN_POINT('Ctrl Pts',(1.81436959209778,1.,-1.22453613304507));
#32870=CARTESIAN_POINT('Ctrl Pts',(1.81655087183054,-1.,-1.22921864890975));
#32871=CARTESIAN_POINT('Ctrl Pts',(1.81655087183054,1.,-1.22921864890975));
#32872=CARTESIAN_POINT('Ctrl Pts',(1.81817389920914,-1.,-1.23274224526804));
#32873=CARTESIAN_POINT('Ctrl Pts',(1.81817389920914,1.,-1.23274224526804));
#32874=CARTESIAN_POINT('Ctrl Pts',(1.81925017193531,-1.,-1.23509651170384));
#32875=CARTESIAN_POINT('Ctrl Pts',(1.81925017193531,1.,-1.23509651170384));
#32876=CARTESIAN_POINT('Ctrl Pts',(1.81978687191668,-1.,-1.23627494547115));
#32877=CARTESIAN_POINT('Ctrl Pts',(1.81978687191668,1.,-1.23627494547115));
#32878=CARTESIAN_POINT('',(1.5055822144029,1.,-0.892032620296855));
#32879=CARTESIAN_POINT('Ctrl Pts',(1.5055822144029,1.,-0.892032620296855));
#32880=CARTESIAN_POINT('Ctrl Pts',(1.50980486807181,1.,-0.894452006967538));
#32881=CARTESIAN_POINT('Ctrl Pts',(1.51805569591479,1.,-0.89918504749193));
#32882=CARTESIAN_POINT('Ctrl Pts',(1.52984849890434,1.,-0.905967409640499));
#32883=CARTESIAN_POINT('Ctrl Pts',(1.54440491152807,1.,-0.91437591904658));
#32884=CARTESIAN_POINT('Ctrl Pts',(1.56065988582509,1.,-0.923832188966322));
#32885=CARTESIAN_POINT('Ctrl Pts',(1.57499388385561,1.,-0.932246680128849));
#32886=CARTESIAN_POINT('Ctrl Pts',(1.58744937489796,1.,-0.939646377909319));
#32887=CARTESIAN_POINT('Ctrl Pts',(1.59810042045408,1.,-0.946078063325796));
#32888=CARTESIAN_POINT('Ctrl Pts',(1.60706069897794,1.,-0.951613284361248));
#32889=CARTESIAN_POINT('Ctrl Pts',(1.61449324337233,1.,-0.956354422921573));
#32890=CARTESIAN_POINT('Ctrl Pts',(1.62061638139929,1.,-0.960438326099958));
#32891=CARTESIAN_POINT('Ctrl Pts',(1.6257193066974,1.,-0.964046107037821));
#32892=CARTESIAN_POINT('Ctrl Pts',(1.63013849959083,1.,-0.967387853228041));
#32893=CARTESIAN_POINT('Ctrl Pts',(1.63420665729609,1.,-0.970669715996356));
#32894=CARTESIAN_POINT('Ctrl Pts',(1.63820952658157,1.,-0.974066058287501));
#32895=CARTESIAN_POINT('Ctrl Pts',(1.64233990826831,1.,-0.977689794120297));
#32896=CARTESIAN_POINT('Ctrl Pts',(1.64665139190834,1.,-0.981562530940574));
#32897=CARTESIAN_POINT('Ctrl Pts',(1.6511001661277,1.,-0.985642622921626));
#32898=CARTESIAN_POINT('Ctrl Pts',(1.65559044289746,1.,-0.98985562785445));
#32899=CARTESIAN_POINT('Ctrl Pts',(1.66001553809916,1.,-0.994121836661116));
#32900=CARTESIAN_POINT('Ctrl Pts',(1.66430758030304,1.,-0.998389654952317));
#32901=CARTESIAN_POINT('Ctrl Pts',(1.66846059277231,1.,-1.00265091003682));
#32902=CARTESIAN_POINT('Ctrl Pts',(1.67250335383248,1.,-1.00692206696387));
#32903=CARTESIAN_POINT('Ctrl Pts',(1.67648246776457,1.,-1.01123236493507));
#32904=CARTESIAN_POINT('Ctrl Pts',(1.6804428989482,1.,-1.01561026162787));
#32905=CARTESIAN_POINT('Ctrl Pts',(1.68440578021739,1.,-1.02006795074222));
#32906=CARTESIAN_POINT('Ctrl Pts',(1.68836910178475,1.,-1.02460180535272));
#32907=CARTESIAN_POINT('Ctrl Pts',(1.69231840863471,1.,-1.02919977579155));
#32908=CARTESIAN_POINT('Ctrl Pts',(1.69623414782769,1.,-1.03384646003587));
#32909=CARTESIAN_POINT('Ctrl Pts',(1.70010052930951,1.,-1.03852922490782));
#32910=CARTESIAN_POINT('Ctrl Pts',(1.70391338707969,1.,-1.04324363334546));
#32911=CARTESIAN_POINT('Ctrl Pts',(1.70767646263641,1.,-1.0479908540499));
#32912=CARTESIAN_POINT('Ctrl Pts',(1.71139783543986,1.,-1.05277517202854));
#32913=CARTESIAN_POINT('Ctrl Pts',(1.71508654427022,1.,-1.05760163192481));
#32914=CARTESIAN_POINT('Ctrl Pts',(1.71874858456908,1.,-1.0624732468065));
#32915=CARTESIAN_POINT('Ctrl Pts',(1.72238500928456,1.,-1.06738966975463));
#32916=CARTESIAN_POINT('Ctrl Pts',(1.72599406198489,1.,-1.07234866990252));
#32917=CARTESIAN_POINT('Ctrl Pts',(1.72957248977424,1.,-1.0773470373727));
#32918=CARTESIAN_POINT('Ctrl Pts',(1.73311705663407,1.,-1.08238162784749));
#32919=CARTESIAN_POINT('Ctrl Pts',(1.73662628326093,1.,-1.08745056285429));
#32920=CARTESIAN_POINT('Ctrl Pts',(1.74010053962252,1.,-1.09255329056496));
#32921=CARTESIAN_POINT('Ctrl Pts',(1.74354119236212,1.,-1.09768999241229));
#32922=CARTESIAN_POINT('Ctrl Pts',(1.74695004214924,1.,-1.10286118991144));
#32923=CARTESIAN_POINT('Ctrl Pts',(1.75032866075914,1.,-1.10806728183003));
#32924=CARTESIAN_POINT('Ctrl Pts',(1.75367772094617,1.,-1.11330807582542));
#32925=CARTESIAN_POINT('Ctrl Pts',(1.75699720772089,1.,-1.11858293216752));
#32926=CARTESIAN_POINT('Ctrl Pts',(1.76028671825084,1.,-1.12389096855078));
#32927=CARTESIAN_POINT('Ctrl Pts',(1.76354571966171,1.,-1.12923123555076));
#32928=CARTESIAN_POINT('Ctrl Pts',(1.76677384551883,1.,-1.13460291804635));
#32929=CARTESIAN_POINT('Ctrl Pts',(1.76997111386806,1.,-1.14000548337));
#32930=CARTESIAN_POINT('Ctrl Pts',(1.77313777896234,1.,-1.14543858226948));
#32931=CARTESIAN_POINT('Ctrl Pts',(1.77627422557034,1.,-1.15090197841531));
#32932=CARTESIAN_POINT('Ctrl Pts',(1.77938085564261,1.,-1.15639547194689));
#32933=CARTESIAN_POINT('Ctrl Pts',(1.78245795880949,1.,-1.16191881298458));
#32934=CARTESIAN_POINT('Ctrl Pts',(1.78550566040349,1.,-1.16747166312239));
#32935=CARTESIAN_POINT('Ctrl Pts',(1.78852398877523,1.,-1.17305363177265));
#32936=CARTESIAN_POINT('Ctrl Pts',(1.79151291552646,1.,-1.17866429440781));
#32937=CARTESIAN_POINT('Ctrl Pts',(1.79447240321572,1.,-1.18430321697471));
#32938=CARTESIAN_POINT('Ctrl Pts',(1.79740245923649,1.,-1.1899699793456));
#32939=CARTESIAN_POINT('Ctrl Pts',(1.80030314370121,1.,-1.19566418930405));
#32940=CARTESIAN_POINT('Ctrl Pts',(1.8031745483882,1.,-1.2013854893912));
#32941=CARTESIAN_POINT('Ctrl Pts',(1.80601678480772,1.,-1.20713356605519));
#32942=CARTESIAN_POINT('Ctrl Pts',(1.80882996916931,1.,-1.2129081570818));
#32943=CARTESIAN_POINT('Ctrl Pts',(1.81161420806172,1.,-1.2187090610323));
#32944=CARTESIAN_POINT('Ctrl Pts',(1.81436959209778,1.,-1.22453613304507));
#32945=CARTESIAN_POINT('Ctrl Pts',(1.81655087183054,1.,-1.22921864890975));
#32946=CARTESIAN_POINT('Ctrl Pts',(1.81817389920914,1.,-1.23274224526804));
#32947=CARTESIAN_POINT('Ctrl Pts',(1.81925017193531,1.,-1.23509651170384));
#32948=CARTESIAN_POINT('Ctrl Pts',(1.81978687191668,1.,-1.23627494547115));
#32949=CARTESIAN_POINT('',(1.5055822144029,0.,-0.892032620296855));
#32950=CARTESIAN_POINT('Origin',(0.,0.,0.));
#32951=CARTESIAN_POINT('',(1.60662857109684,1.,-0.693717979106306));
#32952=CARTESIAN_POINT('Origin',(0.,1.,0.));
#32953=CARTESIAN_POINT('',(1.60662857109684,0.,-0.693717979106308));
#32954=CARTESIAN_POINT('Ctrl Pts',(2.0698113262342,-1.,-0.745574324794401));
#32955=CARTESIAN_POINT('Ctrl Pts',(2.0698113262342,1.,-0.745574324794401));
#32956=CARTESIAN_POINT('Ctrl Pts',(2.06854248895728,-1.,-0.745832791378367));
#32957=CARTESIAN_POINT('Ctrl Pts',(2.06854248895728,1.,-0.745832791378367));
#32958=CARTESIAN_POINT('Ctrl Pts',(2.06600523016815,-1.,-0.746345871544201));
#32959=CARTESIAN_POINT('Ctrl Pts',(2.06600523016815,1.,-0.746345871544201));
#32960=CARTESIAN_POINT('Ctrl Pts',(2.06220058927826,-1.,-0.74710393278792));
#32961=CARTESIAN_POINT('Ctrl Pts',(2.06220058927826,1.,-0.74710393278792));
#32962=CARTESIAN_POINT('Ctrl Pts',(2.05713023031006,-1.,-0.748091554183803));
#32963=CARTESIAN_POINT('Ctrl Pts',(2.05713023031006,1.,-0.748091554183803));
#32964=CARTESIAN_POINT('Ctrl Pts',(2.05079645592154,-1.,-0.749287468665046));
#32965=CARTESIAN_POINT('Ctrl Pts',(2.05079645592154,1.,-0.749287468665046));
#32966=CARTESIAN_POINT('Ctrl Pts',(2.04446689147979,-1.,-0.750444657875576));
#32967=CARTESIAN_POINT('Ctrl Pts',(2.04446689147979,1.,-0.750444657875576));
#32968=CARTESIAN_POINT('Ctrl Pts',(2.03814160092099,-1.,-0.751562963361115));
#32969=CARTESIAN_POINT('Ctrl Pts',(2.03814160092099,1.,-0.751562963361115));
#32970=CARTESIAN_POINT('Ctrl Pts',(2.03182068456221,-1.,-0.752642180487211));
#32971=CARTESIAN_POINT('Ctrl Pts',(2.03182068456221,1.,-0.752642180487211));
#32972=CARTESIAN_POINT('Ctrl Pts',(2.02550428623313,-1.,-0.753682061112768));
#32973=CARTESIAN_POINT('Ctrl Pts',(2.02550428623313,1.,-0.753682061112768));
#32974=CARTESIAN_POINT('Ctrl Pts',(2.01919259405809,-1.,-0.754682330722816));
#32975=CARTESIAN_POINT('Ctrl Pts',(2.01919259405809,1.,-0.754682330722816));
#32976=CARTESIAN_POINT('Ctrl Pts',(2.01288584328084,-1.,-0.755642704957865));
#32977=CARTESIAN_POINT('Ctrl Pts',(2.01288584328084,1.,-0.755642704957865));
#32978=CARTESIAN_POINT('Ctrl Pts',(2.0065843158773,-1.,-0.756562904646671));
#32979=CARTESIAN_POINT('Ctrl Pts',(2.0065843158773,1.,-0.756562904646671));
#32980=CARTESIAN_POINT('Ctrl Pts',(2.00028834739178,-1.,-0.757442676862724));
#32981=CARTESIAN_POINT('Ctrl Pts',(2.00028834739178,1.,-0.757442676862724));
#32982=CARTESIAN_POINT('Ctrl Pts',(1.99399831098817,-1.,-0.758281796766761));
#32983=CARTESIAN_POINT('Ctrl Pts',(1.99399831098817,1.,-0.758281796766761));
#32984=CARTESIAN_POINT('Ctrl Pts',(1.98771456680874,-1.,-0.759080037802488));
#32985=CARTESIAN_POINT('Ctrl Pts',(1.98771456680874,1.,-0.759080037802488));
#32986=CARTESIAN_POINT('Ctrl Pts',(1.98143741418172,-1.,-0.75983714745219));
#32987=CARTESIAN_POINT('Ctrl Pts',(1.98143741418172,1.,-0.75983714745219));
#32988=CARTESIAN_POINT('Ctrl Pts',(1.97516705321494,-1.,-0.760552825409757));
#32989=CARTESIAN_POINT('Ctrl Pts',(1.97516705321494,1.,-0.760552825409757));
#32990=CARTESIAN_POINT('Ctrl Pts',(1.96890351582499,-1.,-0.761226690483821));
#32991=CARTESIAN_POINT('Ctrl Pts',(1.96890351582499,1.,-0.761226690483821));
#32992=CARTESIAN_POINT('Ctrl Pts',(1.96264672744186,-1.,-0.761858300014424));
#32993=CARTESIAN_POINT('Ctrl Pts',(1.96264672744186,1.,-0.761858300014424));
#32994=CARTESIAN_POINT('Ctrl Pts',(1.95639665309869,-1.,-0.762447203806179));
#32995=CARTESIAN_POINT('Ctrl Pts',(1.95639665309869,1.,-0.762447203806179));
#32996=CARTESIAN_POINT('Ctrl Pts',(1.95015342590024,-1.,-0.762992990878769));
#32997=CARTESIAN_POINT('Ctrl Pts',(1.95015342590024,1.,-0.762992990878769));
#32998=CARTESIAN_POINT('Ctrl Pts',(1.9439174661764,-1.,-0.763495333538629));
#32999=CARTESIAN_POINT('Ctrl Pts',(1.9439174661764,1.,-0.763495333538629));
#33000=CARTESIAN_POINT('Ctrl Pts',(1.93768964875886,-1.,-0.763954049121459));
#33001=CARTESIAN_POINT('Ctrl Pts',(1.93768964875886,1.,-0.763954049121459));
#33002=CARTESIAN_POINT('Ctrl Pts',(1.93147105496382,-1.,-0.764369010673941));
#33003=CARTESIAN_POINT('Ctrl Pts',(1.93147105496382,1.,-0.764369010673941));
#33004=CARTESIAN_POINT('Ctrl Pts',(1.92526263537048,-1.,-0.764740025488212));
#33005=CARTESIAN_POINT('Ctrl Pts',(1.92526263537048,1.,-0.764740025488212));
#33006=CARTESIAN_POINT('Ctrl Pts',(1.91906491634196,-1.,-0.765066729667089));
#33007=CARTESIAN_POINT('Ctrl Pts',(1.91906491634196,1.,-0.765066729667089));
#33008=CARTESIAN_POINT('Ctrl Pts',(1.91287765805169,-1.,-0.765348465884722));
#33009=CARTESIAN_POINT('Ctrl Pts',(1.91287765805169,1.,-0.765348465884722));
#33010=CARTESIAN_POINT('Ctrl Pts',(1.90669961402356,-1.,-0.765584196937919));
#33011=CARTESIAN_POINT('Ctrl Pts',(1.90669961402356,1.,-0.765584196937919));
#33012=CARTESIAN_POINT('Ctrl Pts',(1.90052930393596,-1.,-0.765772772593386));
#33013=CARTESIAN_POINT('Ctrl Pts',(1.90052930393596,1.,-0.765772772593386));
#33014=CARTESIAN_POINT('Ctrl Pts',(1.89436577771388,-1.,-0.765913193856978));
#33015=CARTESIAN_POINT('Ctrl Pts',(1.89436577771388,1.,-0.765913193856978));
#33016=CARTESIAN_POINT('Ctrl Pts',(1.88820926433409,-1.,-0.766004837062091));
#33017=CARTESIAN_POINT('Ctrl Pts',(1.88820926433409,1.,-0.766004837062091));
#33018=CARTESIAN_POINT('Ctrl Pts',(1.88206215302561,-1.,-0.766047794851865));
#33019=CARTESIAN_POINT('Ctrl Pts',(1.88206215302561,1.,-0.766047794851865));
#33020=CARTESIAN_POINT('Ctrl Pts',(1.87592888967883,-1.,-0.766042837036744));
#33021=CARTESIAN_POINT('Ctrl Pts',(1.87592888967883,1.,-0.766042837036744));
#33022=CARTESIAN_POINT('Ctrl Pts',(1.86981398314341,-1.,-0.765990708546091));
#33023=CARTESIAN_POINT('Ctrl Pts',(1.86981398314341,1.,-0.765990708546091));
#33024=CARTESIAN_POINT('Ctrl Pts',(1.86372027063312,-1.,-0.765891519092547));
#33025=CARTESIAN_POINT('Ctrl Pts',(1.86372027063312,1.,-0.765891519092547));
#33026=CARTESIAN_POINT('Ctrl Pts',(1.85764741390394,-1.,-0.765744212909319));
#33027=CARTESIAN_POINT('Ctrl Pts',(1.85764741390394,1.,-0.765744212909319));
#33028=CARTESIAN_POINT('Ctrl Pts',(1.85158945130063,-1.,-0.765545710619063));
#33029=CARTESIAN_POINT('Ctrl Pts',(1.85158945130063,1.,-0.765545710619063));
#33030=CARTESIAN_POINT('Ctrl Pts',(1.84553698875924,-1.,-0.765291664862029));
#33031=CARTESIAN_POINT('Ctrl Pts',(1.84553698875924,1.,-0.765291664862029));
#33032=CARTESIAN_POINT('Ctrl Pts',(1.83948181064835,-1.,-0.764978057881738));
#33033=CARTESIAN_POINT('Ctrl Pts',(1.83948181064835,1.,-0.764978057881738));
#33034=CARTESIAN_POINT('Ctrl Pts',(1.83342077227142,-1.,-0.764602549687853));
#33035=CARTESIAN_POINT('Ctrl Pts',(1.83342077227142,1.,-0.764602549687853));
#33036=CARTESIAN_POINT('Ctrl Pts',(1.82735991200065,-1.,-0.764165902605995));
#33037=CARTESIAN_POINT('Ctrl Pts',(1.82735991200065,1.,-0.764165902605995));
#33038=CARTESIAN_POINT('Ctrl Pts',(1.82131873145266,-1.,-0.763673465462727));
#33039=CARTESIAN_POINT('Ctrl Pts',(1.82131873145266,1.,-0.763673465462727));
#33040=CARTESIAN_POINT('Ctrl Pts',(1.8153211840553,-1.,-0.763132003836634));
#33041=CARTESIAN_POINT('Ctrl Pts',(1.8153211840553,1.,-0.763132003836634));
#33042=CARTESIAN_POINT('Ctrl Pts',(1.80938551463965,-1.,-0.762546129463938));
#33043=CARTESIAN_POINT('Ctrl Pts',(1.80938551463965,1.,-0.762546129463938));
#33044=CARTESIAN_POINT('Ctrl Pts',(1.80351583877342,-1.,-0.761915336443547));
#33045=CARTESIAN_POINT('Ctrl Pts',(1.80351583877342,1.,-0.761915336443547));
#33046=CARTESIAN_POINT('Ctrl Pts',(1.79768986997783,-1.,-0.761229695230558));
#33047=CARTESIAN_POINT('Ctrl Pts',(1.79768986997783,1.,-0.761229695230558));
#33048=CARTESIAN_POINT('Ctrl Pts',(1.7918581561088,-1.,-0.760469555880749));
#33049=CARTESIAN_POINT('Ctrl Pts',(1.7918581561088,1.,-0.760469555880749));
#33050=CARTESIAN_POINT('Ctrl Pts',(1.78596964884604,-1.,-0.75961440111019));
#33051=CARTESIAN_POINT('Ctrl Pts',(1.78596964884604,1.,-0.75961440111019));
#33052=CARTESIAN_POINT('Ctrl Pts',(1.77999411220945,-1.,-0.758650626677519));
#33053=CARTESIAN_POINT('Ctrl Pts',(1.77999411220945,1.,-0.758650626677519));
#33054=CARTESIAN_POINT('Ctrl Pts',(1.77394167108292,-1.,-0.757578264077029));
#33055=CARTESIAN_POINT('Ctrl Pts',(1.77394167108292,1.,-0.757578264077029));
#33056=CARTESIAN_POINT('Ctrl Pts',(1.76789396002998,-1.,-0.75642189602781));
#33057=CARTESIAN_POINT('Ctrl Pts',(1.76789396002998,1.,-0.75642189602781));
#33058=CARTESIAN_POINT('Ctrl Pts',(1.76197817240128,-1.,-0.755220979974462));
#33059=CARTESIAN_POINT('Ctrl Pts',(1.76197817240128,1.,-0.755220979974462));
#33060=CARTESIAN_POINT('Ctrl Pts',(1.75631083600019,-1.,-0.754009254027829));
#33061=CARTESIAN_POINT('Ctrl Pts',(1.75631083600019,1.,-0.754009254027829));
#33062=CARTESIAN_POINT('Ctrl Pts',(1.75095139468794,-1.,-0.752797683531314));
#33063=CARTESIAN_POINT('Ctrl Pts',(1.75095139468794,1.,-0.752797683531314));
#33064=CARTESIAN_POINT('Ctrl Pts',(1.74585086852502,-1.,-0.751555614164483));
#33065=CARTESIAN_POINT('Ctrl Pts',(1.74585086852502,1.,-0.751555614164483));
#33066=CARTESIAN_POINT('Ctrl Pts',(1.74080458267114,-1.,-0.75019343598125));
#33067=CARTESIAN_POINT('Ctrl Pts',(1.74080458267114,1.,-0.75019343598125));
#33068=CARTESIAN_POINT('Ctrl Pts',(1.7355035168033,-1.,-0.74858246295687));
#33069=CARTESIAN_POINT('Ctrl Pts',(1.7355035168033,1.,-0.74858246295687));
#33070=CARTESIAN_POINT('Ctrl Pts',(1.72958533647714,-1.,-0.746574710097752));
#33071=CARTESIAN_POINT('Ctrl Pts',(1.72958533647714,1.,-0.746574710097752));
#33072=CARTESIAN_POINT('Ctrl Pts',(1.72268229916769,-1.,-0.744021445433094));
#33073=CARTESIAN_POINT('Ctrl Pts',(1.72268229916769,1.,-0.744021445433094));
#33074=CARTESIAN_POINT('Ctrl Pts',(1.71447789751001,-1.,-0.74079516202821));
#33075=CARTESIAN_POINT('Ctrl Pts',(1.71447789751001,1.,-0.74079516202821));
#33076=CARTESIAN_POINT('Ctrl Pts',(1.70473309004249,-1.,-0.736799665716932));
#33077=CARTESIAN_POINT('Ctrl Pts',(1.70473309004249,1.,-0.736799665716932));
#33078=CARTESIAN_POINT('Ctrl Pts',(1.69326921972915,-1.,-0.731963238685357));
#33079=CARTESIAN_POINT('Ctrl Pts',(1.69326921972915,1.,-0.731963238685357));
#33080=CARTESIAN_POINT('Ctrl Pts',(1.67996158451922,-1.,-0.726235967982445));
#33081=CARTESIAN_POINT('Ctrl Pts',(1.67996158451922,1.,-0.726235967982445));
#33082=CARTESIAN_POINT('Ctrl Pts',(1.66472880551777,-1.,-0.71958543378795));
#33083=CARTESIAN_POINT('Ctrl Pts',(1.66472880551777,1.,-0.71958543378795));
#33084=CARTESIAN_POINT('Ctrl Pts',(1.64752408828442,-1.,-0.711993139340448));
#33085=CARTESIAN_POINT('Ctrl Pts',(1.64752408828442,1.,-0.711993139340448));
#33086=CARTESIAN_POINT('Ctrl Pts',(1.6321654166204,-1.,-0.705159151977294));
#33087=CARTESIAN_POINT('Ctrl Pts',(1.6321654166204,1.,-0.705159151977294));
#33088=CARTESIAN_POINT('Ctrl Pts',(1.61974673471117,-1.,-0.699605146398837));
#33089=CARTESIAN_POINT('Ctrl Pts',(1.61974673471117,1.,-0.699605146398837));
#33090=CARTESIAN_POINT('Ctrl Pts',(1.61106790957619,-1.,-0.69571209787897));
#33091=CARTESIAN_POINT('Ctrl Pts',(1.61106790957619,1.,-0.69571209787897));
#33092=CARTESIAN_POINT('Ctrl Pts',(1.60662857109684,-1.,-0.693717979106306));
#33093=CARTESIAN_POINT('Ctrl Pts',(1.60662857109684,1.,-0.693717979106306));
#33094=CARTESIAN_POINT('',(2.0698113262342,1.,-0.745574324794401));
#33095=CARTESIAN_POINT('Ctrl Pts',(2.0698113262342,1.,-0.745574324794401));
#33096=CARTESIAN_POINT('Ctrl Pts',(2.06854248895728,1.,-0.745832791378367));
#33097=CARTESIAN_POINT('Ctrl Pts',(2.06600523016815,1.,-0.746345871544201));
#33098=CARTESIAN_POINT('Ctrl Pts',(2.06220058927826,1.,-0.74710393278792));
#33099=CARTESIAN_POINT('Ctrl Pts',(2.05713023031006,1.,-0.748091554183803));
#33100=CARTESIAN_POINT('Ctrl Pts',(2.05079645592154,1.,-0.749287468665046));
#33101=CARTESIAN_POINT('Ctrl Pts',(2.04446689147979,1.,-0.750444657875576));
#33102=CARTESIAN_POINT('Ctrl Pts',(2.03814160092099,1.,-0.751562963361115));
#33103=CARTESIAN_POINT('Ctrl Pts',(2.03182068456221,1.,-0.752642180487211));
#33104=CARTESIAN_POINT('Ctrl Pts',(2.02550428623313,1.,-0.753682061112768));
#33105=CARTESIAN_POINT('Ctrl Pts',(2.01919259405809,1.,-0.754682330722816));
#33106=CARTESIAN_POINT('Ctrl Pts',(2.01288584328084,1.,-0.755642704957865));
#33107=CARTESIAN_POINT('Ctrl Pts',(2.0065843158773,1.,-0.756562904646671));
#33108=CARTESIAN_POINT('Ctrl Pts',(2.00028834739178,1.,-0.757442676862724));
#33109=CARTESIAN_POINT('Ctrl Pts',(1.99399831098817,1.,-0.758281796766761));
#33110=CARTESIAN_POINT('Ctrl Pts',(1.98771456680874,1.,-0.759080037802488));
#33111=CARTESIAN_POINT('Ctrl Pts',(1.98143741418172,1.,-0.75983714745219));
#33112=CARTESIAN_POINT('Ctrl Pts',(1.97516705321494,1.,-0.760552825409757));
#33113=CARTESIAN_POINT('Ctrl Pts',(1.96890351582499,1.,-0.761226690483821));
#33114=CARTESIAN_POINT('Ctrl Pts',(1.96264672744186,1.,-0.761858300014424));
#33115=CARTESIAN_POINT('Ctrl Pts',(1.95639665309869,1.,-0.762447203806179));
#33116=CARTESIAN_POINT('Ctrl Pts',(1.95015342590024,1.,-0.762992990878769));
#33117=CARTESIAN_POINT('Ctrl Pts',(1.9439174661764,1.,-0.763495333538629));
#33118=CARTESIAN_POINT('Ctrl Pts',(1.93768964875886,1.,-0.763954049121459));
#33119=CARTESIAN_POINT('Ctrl Pts',(1.93147105496382,1.,-0.764369010673941));
#33120=CARTESIAN_POINT('Ctrl Pts',(1.92526263537048,1.,-0.764740025488212));
#33121=CARTESIAN_POINT('Ctrl Pts',(1.91906491634196,1.,-0.765066729667089));
#33122=CARTESIAN_POINT('Ctrl Pts',(1.91287765805169,1.,-0.765348465884722));
#33123=CARTESIAN_POINT('Ctrl Pts',(1.90669961402356,1.,-0.765584196937919));
#33124=CARTESIAN_POINT('Ctrl Pts',(1.90052930393596,1.,-0.765772772593386));
#33125=CARTESIAN_POINT('Ctrl Pts',(1.89436577771388,1.,-0.765913193856978));
#33126=CARTESIAN_POINT('Ctrl Pts',(1.88820926433409,1.,-0.766004837062091));
#33127=CARTESIAN_POINT('Ctrl Pts',(1.88206215302561,1.,-0.766047794851865));
#33128=CARTESIAN_POINT('Ctrl Pts',(1.87592888967883,1.,-0.766042837036744));
#33129=CARTESIAN_POINT('Ctrl Pts',(1.86981398314341,1.,-0.765990708546091));
#33130=CARTESIAN_POINT('Ctrl Pts',(1.86372027063312,1.,-0.765891519092547));
#33131=CARTESIAN_POINT('Ctrl Pts',(1.85764741390394,1.,-0.765744212909319));
#33132=CARTESIAN_POINT('Ctrl Pts',(1.85158945130063,1.,-0.765545710619063));
#33133=CARTESIAN_POINT('Ctrl Pts',(1.84553698875924,1.,-0.765291664862029));
#33134=CARTESIAN_POINT('Ctrl Pts',(1.83948181064835,1.,-0.764978057881738));
#33135=CARTESIAN_POINT('Ctrl Pts',(1.83342077227142,1.,-0.764602549687853));
#33136=CARTESIAN_POINT('Ctrl Pts',(1.82735991200065,1.,-0.764165902605995));
#33137=CARTESIAN_POINT('Ctrl Pts',(1.82131873145266,1.,-0.763673465462727));
#33138=CARTESIAN_POINT('Ctrl Pts',(1.8153211840553,1.,-0.763132003836634));
#33139=CARTESIAN_POINT('Ctrl Pts',(1.80938551463965,1.,-0.762546129463938));
#33140=CARTESIAN_POINT('Ctrl Pts',(1.80351583877342,1.,-0.761915336443547));
#33141=CARTESIAN_POINT('Ctrl Pts',(1.79768986997783,1.,-0.761229695230558));
#33142=CARTESIAN_POINT('Ctrl Pts',(1.7918581561088,1.,-0.760469555880749));
#33143=CARTESIAN_POINT('Ctrl Pts',(1.78596964884604,1.,-0.75961440111019));
#33144=CARTESIAN_POINT('Ctrl Pts',(1.77999411220945,1.,-0.758650626677519));
#33145=CARTESIAN_POINT('Ctrl Pts',(1.77394167108292,1.,-0.757578264077029));
#33146=CARTESIAN_POINT('Ctrl Pts',(1.76789396002998,1.,-0.75642189602781));
#33147=CARTESIAN_POINT('Ctrl Pts',(1.76197817240128,1.,-0.755220979974462));
#33148=CARTESIAN_POINT('Ctrl Pts',(1.75631083600019,1.,-0.754009254027829));
#33149=CARTESIAN_POINT('Ctrl Pts',(1.75095139468794,1.,-0.752797683531314));
#33150=CARTESIAN_POINT('Ctrl Pts',(1.74585086852502,1.,-0.751555614164483));
#33151=CARTESIAN_POINT('Ctrl Pts',(1.74080458267114,1.,-0.75019343598125));
#33152=CARTESIAN_POINT('Ctrl Pts',(1.7355035168033,1.,-0.74858246295687));
#33153=CARTESIAN_POINT('Ctrl Pts',(1.72958533647714,1.,-0.746574710097752));
#33154=CARTESIAN_POINT('Ctrl Pts',(1.72268229916769,1.,-0.744021445433094));
#33155=CARTESIAN_POINT('Ctrl Pts',(1.71447789751001,1.,-0.74079516202821));
#33156=CARTESIAN_POINT('Ctrl Pts',(1.70473309004249,1.,-0.736799665716932));
#33157=CARTESIAN_POINT('Ctrl Pts',(1.69326921972915,1.,-0.731963238685357));
#33158=CARTESIAN_POINT('Ctrl Pts',(1.67996158451922,1.,-0.726235967982445));
#33159=CARTESIAN_POINT('Ctrl Pts',(1.66472880551777,1.,-0.71958543378795));
#33160=CARTESIAN_POINT('Ctrl Pts',(1.64752408828442,1.,-0.711993139340448));
#33161=CARTESIAN_POINT('Ctrl Pts',(1.6321654166204,1.,-0.705159151977294));
#33162=CARTESIAN_POINT('Ctrl Pts',(1.61974673471117,1.,-0.699605146398837));
#33163=CARTESIAN_POINT('Ctrl Pts',(1.61106790957619,1.,-0.69571209787897));
#33164=CARTESIAN_POINT('Ctrl Pts',(1.60662857109684,1.,-0.693717979106306));
#33165=CARTESIAN_POINT('',(2.0698113262342,0.,-0.745574324794401));
#33166=CARTESIAN_POINT('Origin',(2.11275013067528,0.,-0.61342227326009));
#33167=CARTESIAN_POINT('',(2.11275013067528,1.,-0.61342227326009));
#33168=CARTESIAN_POINT('',(2.0698113262342,1.,-0.745574324794401));
#33169=CARTESIAN_POINT('',(2.11275013067528,0.,-0.61342227326009));
#33170=CARTESIAN_POINT('Ctrl Pts',(1.7075470150345,-1.,-0.383122945602004));
#33171=CARTESIAN_POINT('Ctrl Pts',(1.7075470150345,1.,-0.383122945602004));
#33172=CARTESIAN_POINT('Ctrl Pts',(1.71231062891958,-1.,-0.384119047315542));
#33173=CARTESIAN_POINT('Ctrl Pts',(1.71231062891958,1.,-0.384119047315542));
#33174=CARTESIAN_POINT('Ctrl Pts',(1.72162022246158,-1.,-0.38607079032701));
#33175=CARTESIAN_POINT('Ctrl Pts',(1.72162022246158,1.,-0.38607079032701));
#33176=CARTESIAN_POINT('Ctrl Pts',(1.7349317097561,-1.,-0.388877023509192));
#33177=CARTESIAN_POINT('Ctrl Pts',(1.7349317097561,1.,-0.388877023509192));
#33178=CARTESIAN_POINT('Ctrl Pts',(1.75137405313962,-1.,-0.392375812294307));
#33179=CARTESIAN_POINT('Ctrl Pts',(1.75137405313962,1.,-0.392375812294307));
#33180=CARTESIAN_POINT('Ctrl Pts',(1.7697556004756,-1.,-0.39634619612042));
#33181=CARTESIAN_POINT('Ctrl Pts',(1.7697556004756,1.,-0.39634619612042));
#33182=CARTESIAN_POINT('Ctrl Pts',(1.78598826347533,-1.,-0.399919403783081));
#33183=CARTESIAN_POINT('Ctrl Pts',(1.78598826347533,1.,-0.399919403783081));
#33184=CARTESIAN_POINT('Ctrl Pts',(1.80012077176221,-1.,-0.403107976170441));
#33185=CARTESIAN_POINT('Ctrl Pts',(1.80012077176221,1.,-0.403107976170441));
#33186=CARTESIAN_POINT('Ctrl Pts',(1.81223801813988,-1.,-0.405933518411838));
#33187=CARTESIAN_POINT('Ctrl Pts',(1.81223801813988,1.,-0.405933518411838));
#33188=CARTESIAN_POINT('Ctrl Pts',(1.8224702267854,-1.,-0.408428948108534));
#33189=CARTESIAN_POINT('Ctrl Pts',(1.8224702267854,1.,-0.408428948108534));
#33190=CARTESIAN_POINT('Ctrl Pts',(1.83100408895216,-1.,-0.410641256301675));
#33191=CARTESIAN_POINT('Ctrl Pts',(1.83100408895216,1.,-0.410641256301675));
#33192=CARTESIAN_POINT('Ctrl Pts',(1.83808953475839,-1.,-0.412633125322162));
#33193=CARTESIAN_POINT('Ctrl Pts',(1.83808953475839,1.,-0.412633125322162));
#33194=CARTESIAN_POINT('Ctrl Pts',(1.8440575707371,-1.,-0.41448743825434));
#33195=CARTESIAN_POINT('Ctrl Pts',(1.8440575707371,1.,-0.41448743825434));
#33196=CARTESIAN_POINT('Ctrl Pts',(1.84929312929882,-1.,-0.416300022038864));
#33197=CARTESIAN_POINT('Ctrl Pts',(1.84929312929882,1.,-0.416300022038864));
#33198=CARTESIAN_POINT('Ctrl Pts',(1.85417632856234,-1.,-0.418164129143534));
#33199=CARTESIAN_POINT('Ctrl Pts',(1.85417632856234,1.,-0.418164129143534));
#33200=CARTESIAN_POINT('Ctrl Pts',(1.85903281096686,-1.,-0.42015728797562));
#33201=CARTESIAN_POINT('Ctrl Pts',(1.85903281096686,1.,-0.42015728797562));
#33202=CARTESIAN_POINT('Ctrl Pts',(1.86408083334028,-1.,-0.422327307418275));
#33203=CARTESIAN_POINT('Ctrl Pts',(1.86408083334028,1.,-0.422327307418275));
#33204=CARTESIAN_POINT('Ctrl Pts',(1.86937803944323,-1.,-0.424678177291359));
#33205=CARTESIAN_POINT('Ctrl Pts',(1.86937803944323,1.,-0.424678177291359));
#33206=CARTESIAN_POINT('Ctrl Pts',(1.87486989291484,-1.,-0.427183828519102));
#33207=CARTESIAN_POINT('Ctrl Pts',(1.87486989291484,1.,-0.427183828519102));
#33208=CARTESIAN_POINT('Ctrl Pts',(1.88044229001832,-1.,-0.429803062482345));
#33209=CARTESIAN_POINT('Ctrl Pts',(1.88044229001832,1.,-0.429803062482345));
#33210=CARTESIAN_POINT('Ctrl Pts',(1.88596913666793,-1.,-0.432493038548748));
#33211=CARTESIAN_POINT('Ctrl Pts',(1.88596913666793,1.,-0.432493038548748));
#33212=CARTESIAN_POINT('Ctrl Pts',(1.89136993975504,-1.,-0.435225660963383));
#33213=CARTESIAN_POINT('Ctrl Pts',(1.89136993975504,1.,-0.435225660963383));
#33214=CARTESIAN_POINT('Ctrl Pts',(1.89663648956466,-1.,-0.437995003948244));
#33215=CARTESIAN_POINT('Ctrl Pts',(1.89663648956466,1.,-0.437995003948244));
#33216=CARTESIAN_POINT('Ctrl Pts',(1.90180124389086,-1.,-0.440807833704038));
#33217=CARTESIAN_POINT('Ctrl Pts',(1.90180124389086,1.,-0.440807833704038));
#33218=CARTESIAN_POINT('Ctrl Pts',(1.90691756144898,-1.,-0.443677556849151));
#33219=CARTESIAN_POINT('Ctrl Pts',(1.90691756144898,1.,-0.443677556849151));
#33220=CARTESIAN_POINT('Ctrl Pts',(1.9120369998112,-1.,-0.446617343485711));
#33221=CARTESIAN_POINT('Ctrl Pts',(1.9120369998112,1.,-0.446617343485711));
#33222=CARTESIAN_POINT('Ctrl Pts',(1.91718342555755,-1.,-0.449632260106662));
#33223=CARTESIAN_POINT('Ctrl Pts',(1.91718342555755,1.,-0.449632260106662));
#33224=CARTESIAN_POINT('Ctrl Pts',(1.92235380648502,-1.,-0.452719478359433));
#33225=CARTESIAN_POINT('Ctrl Pts',(1.92235380648502,1.,-0.452719478359433));
#33226=CARTESIAN_POINT('Ctrl Pts',(1.92753067150476,-1.,-0.455872005174371));
#33227=CARTESIAN_POINT('Ctrl Pts',(1.92753067150476,1.,-0.455872005174371));
#33228=CARTESIAN_POINT('Ctrl Pts',(1.93269066517934,-1.,-0.459081234547926));
#33229=CARTESIAN_POINT('Ctrl Pts',(1.93269066517934,1.,-0.459081234547926));
#33230=CARTESIAN_POINT('Ctrl Pts',(1.93781486640821,-1.,-0.462340031009057));
#33231=CARTESIAN_POINT('Ctrl Pts',(1.93781486640821,1.,-0.462340031009057));
#33232=CARTESIAN_POINT('Ctrl Pts',(1.9428979419619,-1.,-0.46564546202603));
#33233=CARTESIAN_POINT('Ctrl Pts',(1.9428979419619,1.,-0.46564546202603));
#33234=CARTESIAN_POINT('Ctrl Pts',(1.94794381136514,-1.,-0.468997482913135));
#33235=CARTESIAN_POINT('Ctrl Pts',(1.94794381136514,1.,-0.468997482913135));
#33236=CARTESIAN_POINT('Ctrl Pts',(1.95296148278133,-1.,-0.472397672264072));
#33237=CARTESIAN_POINT('Ctrl Pts',(1.95296148278133,1.,-0.472397672264072));
#33238=CARTESIAN_POINT('Ctrl Pts',(1.95796111148177,-1.,-0.475848034683176));
#33239=CARTESIAN_POINT('Ctrl Pts',(1.95796111148177,1.,-0.475848034683176));
#33240=CARTESIAN_POINT('Ctrl Pts',(1.96294933055943,-1.,-0.479349583074855));
#33241=CARTESIAN_POINT('Ctrl Pts',(1.96294933055943,1.,-0.479349583074855));
#33242=CARTESIAN_POINT('Ctrl Pts',(1.96792703422362,-1.,-0.482901662120691));
#33243=CARTESIAN_POINT('Ctrl Pts',(1.96792703422362,1.,-0.482901662120691));
#33244=CARTESIAN_POINT('Ctrl Pts',(1.97289186263272,-1.,-0.486502692907659));
#33245=CARTESIAN_POINT('Ctrl Pts',(1.97289186263272,1.,-0.486502692907659));
#33246=CARTESIAN_POINT('Ctrl Pts',(1.97783973019229,-1.,-0.490150627860953));
#33247=CARTESIAN_POINT('Ctrl Pts',(1.97783973019229,1.,-0.490150627860953));
#33248=CARTESIAN_POINT('Ctrl Pts',(1.98276658761821,-1.,-0.493843476541495));
#33249=CARTESIAN_POINT('Ctrl Pts',(1.98276658761821,1.,-0.493843476541495));
#33250=CARTESIAN_POINT('Ctrl Pts',(1.98767044752932,-1.,-0.497579909545574));
#33251=CARTESIAN_POINT('Ctrl Pts',(1.98767044752932,1.,-0.497579909545574));
#33252=CARTESIAN_POINT('Ctrl Pts',(1.99255149126155,-1.,-0.501359287727146));
#33253=CARTESIAN_POINT('Ctrl Pts',(1.99255149126155,1.,-0.501359287727146));
#33254=CARTESIAN_POINT('Ctrl Pts',(1.99741107463572,-1.,-0.505181361323026));
#33255=CARTESIAN_POINT('Ctrl Pts',(1.99741107463572,1.,-0.505181361323026));
#33256=CARTESIAN_POINT('Ctrl Pts',(2.00225107134734,-1.,-0.509046069886157));
#33257=CARTESIAN_POINT('Ctrl Pts',(2.00225107134734,1.,-0.509046069886157));
#33258=CARTESIAN_POINT('Ctrl Pts',(2.00707309946949,-1.,-0.512953306961793));
#33259=CARTESIAN_POINT('Ctrl Pts',(2.00707309946949,1.,-0.512953306961793));
#33260=CARTESIAN_POINT('Ctrl Pts',(2.01187773939242,-1.,-0.516902681728687));
#33261=CARTESIAN_POINT('Ctrl Pts',(2.01187773939242,1.,-0.516902681728687));
#33262=CARTESIAN_POINT('Ctrl Pts',(2.01666477917286,-1.,-0.520893590399371));
#33263=CARTESIAN_POINT('Ctrl Pts',(2.01666477917286,1.,-0.520893590399371));
#33264=CARTESIAN_POINT('Ctrl Pts',(2.02143356304698,-1.,-0.524925318333476));
#33265=CARTESIAN_POINT('Ctrl Pts',(2.02143356304698,1.,-0.524925318333476));
#33266=CARTESIAN_POINT('Ctrl Pts',(2.0261832908329,-1.,-0.528997127241914));
#33267=CARTESIAN_POINT('Ctrl Pts',(2.0261832908329,1.,-0.528997127241914));
#33268=CARTESIAN_POINT('Ctrl Pts',(2.03091336214426,-1.,-0.533108355132977));
#33269=CARTESIAN_POINT('Ctrl Pts',(2.03091336214426,1.,-0.533108355132977));
#33270=CARTESIAN_POINT('Ctrl Pts',(2.03562362954037,-1.,-0.537258489833262));
#33271=CARTESIAN_POINT('Ctrl Pts',(2.03562362954037,1.,-0.537258489833262));
#33272=CARTESIAN_POINT('Ctrl Pts',(2.04031422690527,-1.,-0.541447120615659));
#33273=CARTESIAN_POINT('Ctrl Pts',(2.04031422690527,1.,-0.541447120615659));
#33274=CARTESIAN_POINT('Ctrl Pts',(2.04498544714588,-1.,-0.54567390381743));
#33275=CARTESIAN_POINT('Ctrl Pts',(2.04498544714588,1.,-0.54567390381743));
#33276=CARTESIAN_POINT('Ctrl Pts',(2.04963761077958,-1.,-0.549938525150295));
#33277=CARTESIAN_POINT('Ctrl Pts',(2.04963761077958,1.,-0.549938525150295));
#33278=CARTESIAN_POINT('Ctrl Pts',(2.05427091604413,-1.,-0.554240657463906));
#33279=CARTESIAN_POINT('Ctrl Pts',(2.05427091604413,1.,-0.554240657463906));
#33280=CARTESIAN_POINT('Ctrl Pts',(2.05888537756462,-1.,-0.558579940185152));
#33281=CARTESIAN_POINT('Ctrl Pts',(2.05888537756462,1.,-0.558579940185152));
#33282=CARTESIAN_POINT('Ctrl Pts',(2.06348090160589,-1.,-0.562955993082262));
#33283=CARTESIAN_POINT('Ctrl Pts',(2.06348090160589,1.,-0.562955993082262));
#33284=CARTESIAN_POINT('Ctrl Pts',(2.06805732997334,-1.,-0.567368421181087));
#33285=CARTESIAN_POINT('Ctrl Pts',(2.06805732997334,1.,-0.567368421181087));
#33286=CARTESIAN_POINT('Ctrl Pts',(2.07261449292824,-1.,-0.571816823242603));
#33287=CARTESIAN_POINT('Ctrl Pts',(2.07261449292824,1.,-0.571816823242603));
#33288=CARTESIAN_POINT('Ctrl Pts',(2.07715226767559,-1.,-0.576300797416845));
#33289=CARTESIAN_POINT('Ctrl Pts',(2.07715226767559,1.,-0.576300797416845));
#33290=CARTESIAN_POINT('Ctrl Pts',(2.08167059018418,-1.,-0.580819952108064));
#33291=CARTESIAN_POINT('Ctrl Pts',(2.08167059018418,1.,-0.580819952108064));
#33292=CARTESIAN_POINT('Ctrl Pts',(2.08616943727951,-1.,-0.585373918991617));
#33293=CARTESIAN_POINT('Ctrl Pts',(2.08616943727951,1.,-0.585373918991617));
#33294=CARTESIAN_POINT('Ctrl Pts',(2.09064881812129,-1.,-0.589962365403406));
#33295=CARTESIAN_POINT('Ctrl Pts',(2.09064881812129,1.,-0.589962365403406));
#33296=CARTESIAN_POINT('Ctrl Pts',(2.0951087622027,-1.,-0.594585006052162));
#33297=CARTESIAN_POINT('Ctrl Pts',(2.0951087622027,1.,-0.594585006052162));
#33298=CARTESIAN_POINT('Ctrl Pts',(2.0995493086477,-1.,-0.599241616420534));
#33299=CARTESIAN_POINT('Ctrl Pts',(2.0995493086477,1.,-0.599241616420534));
#33300=CARTESIAN_POINT('Ctrl Pts',(2.10397049886949,-1.,-0.60393203073603));
#33301=CARTESIAN_POINT('Ctrl Pts',(2.10397049886949,1.,-0.60393203073603));
#33302=CARTESIAN_POINT('Ctrl Pts',(2.1074919961518,-1.,-0.607711315454876));
#33303=CARTESIAN_POINT('Ctrl Pts',(2.1074919961518,1.,-0.607711315454876));
#33304=CARTESIAN_POINT('Ctrl Pts',(2.11012443807238,-1.,-0.610560911689899));
#33305=CARTESIAN_POINT('Ctrl Pts',(2.11012443807238,1.,-0.610560911689899));
#33306=CARTESIAN_POINT('Ctrl Pts',(2.11187554259986,-1.,-0.6124673655618));
#33307=CARTESIAN_POINT('Ctrl Pts',(2.11187554259986,1.,-0.6124673655618));
#33308=CARTESIAN_POINT('Ctrl Pts',(2.11275013067528,-1.,-0.61342227326009));
#33309=CARTESIAN_POINT('Ctrl Pts',(2.11275013067528,1.,-0.61342227326009));
#33310=CARTESIAN_POINT('',(1.7075470150345,1.,-0.383122945602004));
#33311=CARTESIAN_POINT('Ctrl Pts',(1.7075470150345,1.,-0.383122945602004));
#33312=CARTESIAN_POINT('Ctrl Pts',(1.71231062891958,1.,-0.384119047315542));
#33313=CARTESIAN_POINT('Ctrl Pts',(1.72162022246158,1.,-0.38607079032701));
#33314=CARTESIAN_POINT('Ctrl Pts',(1.7349317097561,1.,-0.388877023509192));
#33315=CARTESIAN_POINT('Ctrl Pts',(1.75137405313962,1.,-0.392375812294307));
#33316=CARTESIAN_POINT('Ctrl Pts',(1.7697556004756,1.,-0.39634619612042));
#33317=CARTESIAN_POINT('Ctrl Pts',(1.78598826347533,1.,-0.399919403783081));
#33318=CARTESIAN_POINT('Ctrl Pts',(1.80012077176221,1.,-0.403107976170441));
#33319=CARTESIAN_POINT('Ctrl Pts',(1.81223801813988,1.,-0.405933518411838));
#33320=CARTESIAN_POINT('Ctrl Pts',(1.8224702267854,1.,-0.408428948108534));
#33321=CARTESIAN_POINT('Ctrl Pts',(1.83100408895216,1.,-0.410641256301675));
#33322=CARTESIAN_POINT('Ctrl Pts',(1.83808953475839,1.,-0.412633125322162));
#33323=CARTESIAN_POINT('Ctrl Pts',(1.8440575707371,1.,-0.41448743825434));
#33324=CARTESIAN_POINT('Ctrl Pts',(1.84929312929882,1.,-0.416300022038864));
#33325=CARTESIAN_POINT('Ctrl Pts',(1.85417632856234,1.,-0.418164129143534));
#33326=CARTESIAN_POINT('Ctrl Pts',(1.85903281096686,1.,-0.42015728797562));
#33327=CARTESIAN_POINT('Ctrl Pts',(1.86408083334028,1.,-0.422327307418275));
#33328=CARTESIAN_POINT('Ctrl Pts',(1.86937803944323,1.,-0.424678177291359));
#33329=CARTESIAN_POINT('Ctrl Pts',(1.87486989291484,1.,-0.427183828519102));
#33330=CARTESIAN_POINT('Ctrl Pts',(1.88044229001832,1.,-0.429803062482345));
#33331=CARTESIAN_POINT('Ctrl Pts',(1.88596913666793,1.,-0.432493038548748));
#33332=CARTESIAN_POINT('Ctrl Pts',(1.89136993975504,1.,-0.435225660963383));
#33333=CARTESIAN_POINT('Ctrl Pts',(1.89663648956466,1.,-0.437995003948244));
#33334=CARTESIAN_POINT('Ctrl Pts',(1.90180124389086,1.,-0.440807833704038));
#33335=CARTESIAN_POINT('Ctrl Pts',(1.90691756144898,1.,-0.443677556849151));
#33336=CARTESIAN_POINT('Ctrl Pts',(1.9120369998112,1.,-0.446617343485711));
#33337=CARTESIAN_POINT('Ctrl Pts',(1.91718342555755,1.,-0.449632260106662));
#33338=CARTESIAN_POINT('Ctrl Pts',(1.92235380648502,1.,-0.452719478359433));
#33339=CARTESIAN_POINT('Ctrl Pts',(1.92753067150476,1.,-0.455872005174371));
#33340=CARTESIAN_POINT('Ctrl Pts',(1.93269066517934,1.,-0.459081234547926));
#33341=CARTESIAN_POINT('Ctrl Pts',(1.93781486640821,1.,-0.462340031009057));
#33342=CARTESIAN_POINT('Ctrl Pts',(1.9428979419619,1.,-0.46564546202603));
#33343=CARTESIAN_POINT('Ctrl Pts',(1.94794381136514,1.,-0.468997482913135));
#33344=CARTESIAN_POINT('Ctrl Pts',(1.95296148278133,1.,-0.472397672264072));
#33345=CARTESIAN_POINT('Ctrl Pts',(1.95796111148177,1.,-0.475848034683176));
#33346=CARTESIAN_POINT('Ctrl Pts',(1.96294933055943,1.,-0.479349583074855));
#33347=CARTESIAN_POINT('Ctrl Pts',(1.96792703422362,1.,-0.482901662120691));
#33348=CARTESIAN_POINT('Ctrl Pts',(1.97289186263272,1.,-0.486502692907659));
#33349=CARTESIAN_POINT('Ctrl Pts',(1.97783973019229,1.,-0.490150627860953));
#33350=CARTESIAN_POINT('Ctrl Pts',(1.98276658761821,1.,-0.493843476541495));
#33351=CARTESIAN_POINT('Ctrl Pts',(1.98767044752932,1.,-0.497579909545574));
#33352=CARTESIAN_POINT('Ctrl Pts',(1.99255149126155,1.,-0.501359287727146));
#33353=CARTESIAN_POINT('Ctrl Pts',(1.99741107463572,1.,-0.505181361323026));
#33354=CARTESIAN_POINT('Ctrl Pts',(2.00225107134734,1.,-0.509046069886157));
#33355=CARTESIAN_POINT('Ctrl Pts',(2.00707309946949,1.,-0.512953306961793));
#33356=CARTESIAN_POINT('Ctrl Pts',(2.01187773939242,1.,-0.516902681728687));
#33357=CARTESIAN_POINT('Ctrl Pts',(2.01666477917286,1.,-0.520893590399371));
#33358=CARTESIAN_POINT('Ctrl Pts',(2.02143356304698,1.,-0.524925318333476));
#33359=CARTESIAN_POINT('Ctrl Pts',(2.0261832908329,1.,-0.528997127241914));
#33360=CARTESIAN_POINT('Ctrl Pts',(2.03091336214426,1.,-0.533108355132977));
#33361=CARTESIAN_POINT('Ctrl Pts',(2.03562362954037,1.,-0.537258489833262));
#33362=CARTESIAN_POINT('Ctrl Pts',(2.04031422690527,1.,-0.541447120615659));
#33363=CARTESIAN_POINT('Ctrl Pts',(2.04498544714588,1.,-0.54567390381743));
#33364=CARTESIAN_POINT('Ctrl Pts',(2.04963761077958,1.,-0.549938525150295));
#33365=CARTESIAN_POINT('Ctrl Pts',(2.05427091604413,1.,-0.554240657463906));
#33366=CARTESIAN_POINT('Ctrl Pts',(2.05888537756462,1.,-0.558579940185152));
#33367=CARTESIAN_POINT('Ctrl Pts',(2.06348090160589,1.,-0.562955993082262));
#33368=CARTESIAN_POINT('Ctrl Pts',(2.06805732997334,1.,-0.567368421181087));
#33369=CARTESIAN_POINT('Ctrl Pts',(2.07261449292824,1.,-0.571816823242603));
#33370=CARTESIAN_POINT('Ctrl Pts',(2.07715226767559,1.,-0.576300797416845));
#33371=CARTESIAN_POINT('Ctrl Pts',(2.08167059018418,1.,-0.580819952108064));
#33372=CARTESIAN_POINT('Ctrl Pts',(2.08616943727951,1.,-0.585373918991617));
#33373=CARTESIAN_POINT('Ctrl Pts',(2.09064881812129,1.,-0.589962365403406));
#33374=CARTESIAN_POINT('Ctrl Pts',(2.0951087622027,1.,-0.594585006052162));
#33375=CARTESIAN_POINT('Ctrl Pts',(2.0995493086477,1.,-0.599241616420534));
#33376=CARTESIAN_POINT('Ctrl Pts',(2.10397049886949,1.,-0.60393203073603));
#33377=CARTESIAN_POINT('Ctrl Pts',(2.1074919961518,1.,-0.607711315454876));
#33378=CARTESIAN_POINT('Ctrl Pts',(2.11012443807238,1.,-0.610560911689899));
#33379=CARTESIAN_POINT('Ctrl Pts',(2.11187554259986,1.,-0.6124673655618));
#33380=CARTESIAN_POINT('Ctrl Pts',(2.11275013067528,1.,-0.61342227326009));
#33381=CARTESIAN_POINT('',(1.7075470150345,0.,-0.383122945602001));
#33382=CARTESIAN_POINT('Origin',(0.,0.,0.));
#33383=CARTESIAN_POINT('',(1.74236521665491,1.,-0.163289472382896));
#33384=CARTESIAN_POINT('Origin',(0.,1.,0.));
#33385=CARTESIAN_POINT('',(1.74236521665491,0.,-0.163289472382896));
#33386=CARTESIAN_POINT('Ctrl Pts',(2.19890268624765,-1.,-0.0694764450219582));
#33387=CARTESIAN_POINT('Ctrl Pts',(2.19890268624765,1.,-0.0694764450219582));
#33388=CARTESIAN_POINT('Ctrl Pts',(2.19777582085423,-1.,-0.0701143536325491));
#33389=CARTESIAN_POINT('Ctrl Pts',(2.19777582085423,1.,-0.0701143536325491));
#33390=CARTESIAN_POINT('Ctrl Pts',(2.19552129484002,-1.,-0.0713863779526155));
#33391=CARTESIAN_POINT('Ctrl Pts',(2.19552129484002,1.,-0.0713863779526155));
#33392=CARTESIAN_POINT('Ctrl Pts',(2.19213712013662,-1.,-0.0732830357306726));
#33393=CARTESIAN_POINT('Ctrl Pts',(2.19213712013662,1.,-0.0732830357306726));
#33394=CARTESIAN_POINT('Ctrl Pts',(2.1876201139953,-1.,-0.0757891465836149));
#33395=CARTESIAN_POINT('Ctrl Pts',(2.1876201139953,1.,-0.0757891465836149));
#33396=CARTESIAN_POINT('Ctrl Pts',(2.18196589448887,-1.,-0.0788837727685244));
#33397=CARTESIAN_POINT('Ctrl Pts',(2.18196589448887,1.,-0.0788837727685244));
#33398=CARTESIAN_POINT('Ctrl Pts',(2.176303712113,-1.,-0.0819402680872767));
#33399=CARTESIAN_POINT('Ctrl Pts',(2.176303712113,1.,-0.0819402680872767));
#33400=CARTESIAN_POINT('Ctrl Pts',(2.17063357870952,-1.,-0.0849584620835374));
#33401=CARTESIAN_POINT('Ctrl Pts',(2.17063357870952,1.,-0.0849584620835374));
#33402=CARTESIAN_POINT('Ctrl Pts',(2.16495552645014,-1.,-0.0879381291386924));
#33403=CARTESIAN_POINT('Ctrl Pts',(2.16495552645014,1.,-0.0879381291386924));
#33404=CARTESIAN_POINT('Ctrl Pts',(2.15926961544516,-1.,-0.0908789888107267));
#33405=CARTESIAN_POINT('Ctrl Pts',(2.15926961544516,1.,-0.0908789888107267));
#33406=CARTESIAN_POINT('Ctrl Pts',(2.1535759397817,-1.,-0.0937807218867645));
#33407=CARTESIAN_POINT('Ctrl Pts',(2.1535759397817,1.,-0.0937807218867645));
#33408=CARTESIAN_POINT('Ctrl Pts',(2.14787463531795,-1.,-0.096642985230546));
#33409=CARTESIAN_POINT('Ctrl Pts',(2.14787463531795,1.,-0.096642985230546));
#33410=CARTESIAN_POINT('Ctrl Pts',(2.14216588396025,-1.,-0.0994654261990917));
#33411=CARTESIAN_POINT('Ctrl Pts',(2.14216588396025,1.,-0.0994654261990917));
#33412=CARTESIAN_POINT('Ctrl Pts',(2.13644992667165,-1.,-0.102247700556101));
#33413=CARTESIAN_POINT('Ctrl Pts',(2.13644992667165,1.,-0.102247700556101));
#33414=CARTESIAN_POINT('Ctrl Pts',(2.13072704887293,-1.,-0.10498947915274));
#33415=CARTESIAN_POINT('Ctrl Pts',(2.13072704887293,1.,-0.10498947915274));
#33416=CARTESIAN_POINT('Ctrl Pts',(2.12499752307,-1.,-0.10769043523109));
#33417=CARTESIAN_POINT('Ctrl Pts',(2.12499752307,1.,-0.10769043523109));
#33418=CARTESIAN_POINT('Ctrl Pts',(2.11926155590865,-1.,-0.110350236135025));
#33419=CARTESIAN_POINT('Ctrl Pts',(2.11926155590865,1.,-0.110350236135025));
#33420=CARTESIAN_POINT('Ctrl Pts',(2.11351924490306,-1.,-0.112968534419737));
#33421=CARTESIAN_POINT('Ctrl Pts',(2.11351924490306,1.,-0.112968534419737));
#33422=CARTESIAN_POINT('Ctrl Pts',(2.10777050261309,-1.,-0.115544957687927));
#33423=CARTESIAN_POINT('Ctrl Pts',(2.10777050261309,1.,-0.115544957687927));
#33424=CARTESIAN_POINT('Ctrl Pts',(2.102015121329,-1.,-0.118079107988356));
#33425=CARTESIAN_POINT('Ctrl Pts',(2.102015121329,1.,-0.118079107988356));
#33426=CARTESIAN_POINT('Ctrl Pts',(2.0962529286773,-1.,-0.120570567965122));
#33427=CARTESIAN_POINT('Ctrl Pts',(2.0962529286773,1.,-0.120570567965122));
#33428=CARTESIAN_POINT('Ctrl Pts',(2.09048392424825,-1.,-0.123018905621083));
#33429=CARTESIAN_POINT('Ctrl Pts',(2.09048392424825,1.,-0.123018905621083));
#33430=CARTESIAN_POINT('Ctrl Pts',(2.08470840653643,-1.,-0.125423679412062));
#33431=CARTESIAN_POINT('Ctrl Pts',(2.08470840653643,1.,-0.125423679412062));
#33432=CARTESIAN_POINT('Ctrl Pts',(2.07892715110987,-1.,-0.12778444527612));
#33433=CARTESIAN_POINT('Ctrl Pts',(2.07892715110987,1.,-0.12778444527612));
#33434=CARTESIAN_POINT('Ctrl Pts',(2.07314114713063,-1.,-0.130100748328404));
#33435=CARTESIAN_POINT('Ctrl Pts',(2.07314114713063,1.,-0.130100748328404));
#33436=CARTESIAN_POINT('Ctrl Pts',(2.06735123910326,-1.,-0.132372111547711));
#33437=CARTESIAN_POINT('Ctrl Pts',(2.06735123910326,1.,-0.132372111547711));
#33438=CARTESIAN_POINT('Ctrl Pts',(2.06155781517842,-1.,-0.134598026192106));
#33439=CARTESIAN_POINT('Ctrl Pts',(2.06155781517842,1.,-0.134598026192106));
#33440=CARTESIAN_POINT('Ctrl Pts',(2.05576044414264,-1.,-0.136777941218044));
#33441=CARTESIAN_POINT('Ctrl Pts',(2.05576044414264,1.,-0.136777941218044));
#33442=CARTESIAN_POINT('Ctrl Pts',(2.04995762001328,-1.,-0.138911255368966));
#33443=CARTESIAN_POINT('Ctrl Pts',(2.04995762001328,1.,-0.138911255368966));
#33444=CARTESIAN_POINT('Ctrl Pts',(2.04414757947916,-1.,-0.140997332152546));
#33445=CARTESIAN_POINT('Ctrl Pts',(2.04414757947916,1.,-0.140997332152546));
#33446=CARTESIAN_POINT('Ctrl Pts',(2.03832911025912,-1.,-0.143035515058209));
#33447=CARTESIAN_POINT('Ctrl Pts',(2.03832911025912,1.,-0.143035515058209));
#33448=CARTESIAN_POINT('Ctrl Pts',(2.03250223739942,-1.,-0.145025140186058));
#33449=CARTESIAN_POINT('Ctrl Pts',(2.03250223739942,1.,-0.145025140186058));
#33450=CARTESIAN_POINT('Ctrl Pts',(2.02666926182017,-1.,-0.146965557332583));
#33451=CARTESIAN_POINT('Ctrl Pts',(2.02666926182017,1.,-0.146965557332583));
#33452=CARTESIAN_POINT('Ctrl Pts',(2.02083464969894,-1.,-0.148856124775337));
#33453=CARTESIAN_POINT('Ctrl Pts',(2.02083464969894,1.,-0.148856124775337));
#33454=CARTESIAN_POINT('Ctrl Pts',(2.01500291940238,-1.,-0.150696157673078));
#33455=CARTESIAN_POINT('Ctrl Pts',(2.01500291940238,1.,-0.150696157673078));
#33456=CARTESIAN_POINT('Ctrl Pts',(2.00917680318424,-1.,-0.15248488362145));
#33457=CARTESIAN_POINT('Ctrl Pts',(2.00917680318424,1.,-0.15248488362145));
#33458=CARTESIAN_POINT('Ctrl Pts',(2.00335565310543,-1.,-0.154221403049722));
#33459=CARTESIAN_POINT('Ctrl Pts',(2.00335565310543,1.,-0.154221403049722));
#33460=CARTESIAN_POINT('Ctrl Pts',(1.99753284771497,-1.,-0.155904629548784));
#33461=CARTESIAN_POINT('Ctrl Pts',(1.99753284771497,1.,-0.155904629548784));
#33462=CARTESIAN_POINT('Ctrl Pts',(1.99169810931908,-1.,-0.157533331459227));
#33463=CARTESIAN_POINT('Ctrl Pts',(1.99169810931908,1.,-0.157533331459227));
#33464=CARTESIAN_POINT('Ctrl Pts',(1.98584238283292,-1.,-0.159106226437299));
#33465=CARTESIAN_POINT('Ctrl Pts',(1.98584238283292,1.,-0.159106226437299));
#33466=CARTESIAN_POINT('Ctrl Pts',(1.97996195437559,-1.,-0.160622060784611));
#33467=CARTESIAN_POINT('Ctrl Pts',(1.97996195437559,1.,-0.160622060784611));
#33468=CARTESIAN_POINT('Ctrl Pts',(1.97406280235188,-1.,-0.162079693556289));
#33469=CARTESIAN_POINT('Ctrl Pts',(1.97406280235188,1.,-0.162079693556289));
#33470=CARTESIAN_POINT('Ctrl Pts',(1.96816512677967,-1.,-0.163478185457734));
#33471=CARTESIAN_POINT('Ctrl Pts',(1.96816512677967,1.,-0.163478185457734));
#33472=CARTESIAN_POINT('Ctrl Pts',(1.96229379940136,-1.,-0.164816568920269));
#33473=CARTESIAN_POINT('Ctrl Pts',(1.96229379940136,1.,-0.164816568920269));
#33474=CARTESIAN_POINT('Ctrl Pts',(1.9564675971873,-1.,-0.166093592002813));
#33475=CARTESIAN_POINT('Ctrl Pts',(1.9564675971873,1.,-0.166093592002813));
#33476=CARTESIAN_POINT('Ctrl Pts',(1.95069027794294,-1.,-0.167307501784476));
#33477=CARTESIAN_POINT('Ctrl Pts',(1.95069027794294,1.,-0.167307501784476));
#33478=CARTESIAN_POINT('Ctrl Pts',(1.94493757756931,-1.,-0.168455741607556));
#33479=CARTESIAN_POINT('Ctrl Pts',(1.94493757756931,1.,-0.168455741607556));
#33480=CARTESIAN_POINT('Ctrl Pts',(1.93915639211581,-1.,-0.169534904817491));
#33481=CARTESIAN_POINT('Ctrl Pts',(1.93915639211581,1.,-0.169534904817491));
#33482=CARTESIAN_POINT('Ctrl Pts',(1.93329183155539,-1.,-0.170541253116202));
#33483=CARTESIAN_POINT('Ctrl Pts',(1.93329183155539,1.,-0.170541253116202));
#33484=CARTESIAN_POINT('Ctrl Pts',(1.92731093582036,-1.,-0.171471191532988));
#33485=CARTESIAN_POINT('Ctrl Pts',(1.92731093582036,1.,-0.171471191532988));
#33486=CARTESIAN_POINT('Ctrl Pts',(1.9212233439798,-1.,-0.172321621259514));
#33487=CARTESIAN_POINT('Ctrl Pts',(1.9212233439798,1.,-0.172321621259514));
#33488=CARTESIAN_POINT('Ctrl Pts',(1.91511429159527,-1.,-0.173090695383496));
#33489=CARTESIAN_POINT('Ctrl Pts',(1.91511429159527,1.,-0.173090695383496));
#33490=CARTESIAN_POINT('Ctrl Pts',(1.90911693975267,-1.,-0.173776635257817));
#33491=CARTESIAN_POINT('Ctrl Pts',(1.90911693975267,1.,-0.173776635257817));
#33492=CARTESIAN_POINT('Ctrl Pts',(1.90335253862834,-1.,-0.174375518661085));
#33493=CARTESIAN_POINT('Ctrl Pts',(1.90335253862834,1.,-0.174375518661085));
#33494=CARTESIAN_POINT('Ctrl Pts',(1.89788101117132,-1.,-0.174879405091263));
#33495=CARTESIAN_POINT('Ctrl Pts',(1.89788101117132,1.,-0.174879405091263));
#33496=CARTESIAN_POINT('Ctrl Pts',(1.892646301985,-1.,-0.175274276190844));
#33497=CARTESIAN_POINT('Ctrl Pts',(1.892646301985,1.,-0.175274276190844));
#33498=CARTESIAN_POINT('Ctrl Pts',(1.88742606273259,-1.,-0.175538155840648));
#33499=CARTESIAN_POINT('Ctrl Pts',(1.88742606273259,1.,-0.175538155840648));
#33500=CARTESIAN_POINT('Ctrl Pts',(1.88188663145367,-1.,-0.175644148889699));
#33501=CARTESIAN_POINT('Ctrl Pts',(1.88188663145367,1.,-0.175644148889699));
#33502=CARTESIAN_POINT('Ctrl Pts',(1.87563767773588,-1.,-0.175563480746485));
#33503=CARTESIAN_POINT('Ctrl Pts',(1.87563767773588,1.,-0.175563480746485));
#33504=CARTESIAN_POINT('Ctrl Pts',(1.86828349694799,-1.,-0.175268337590758));
#33505=CARTESIAN_POINT('Ctrl Pts',(1.86828349694799,1.,-0.175268337590758));
#33506=CARTESIAN_POINT('Ctrl Pts',(1.85948367088837,-1.,-0.17473525927603));
#33507=CARTESIAN_POINT('Ctrl Pts',(1.85948367088837,1.,-0.17473525927603));
#33508=CARTESIAN_POINT('Ctrl Pts',(1.8489811319852,-1.,-0.173946627587732));
#33509=CARTESIAN_POINT('Ctrl Pts',(1.8489811319852,1.,-0.173946627587732));
#33510=CARTESIAN_POINT('Ctrl Pts',(1.83658380527692,-1.,-0.1728894428919));
#33511=CARTESIAN_POINT('Ctrl Pts',(1.83658380527692,1.,-0.1728894428919));
#33512=CARTESIAN_POINT('Ctrl Pts',(1.82215766811545,-1.,-0.171554770204119));
#33513=CARTESIAN_POINT('Ctrl Pts',(1.82215766811545,1.,-0.171554770204119));
#33514=CARTESIAN_POINT('Ctrl Pts',(1.80561530629706,-1.,-0.169936923904608));
#33515=CARTESIAN_POINT('Ctrl Pts',(1.80561530629706,1.,-0.169936923904608));
#33516=CARTESIAN_POINT('Ctrl Pts',(1.7869064998507,-1.,-0.168032772805197));
#33517=CARTESIAN_POINT('Ctrl Pts',(1.7869064998507,1.,-0.168032772805197));
#33518=CARTESIAN_POINT('Ctrl Pts',(1.77018771684844,-1.,-0.1662793551464));
#33519=CARTESIAN_POINT('Ctrl Pts',(1.77018771684844,1.,-0.1662793551464));
#33520=CARTESIAN_POINT('Ctrl Pts',(1.75666056638427,-1.,-0.164834765707159));
#33521=CARTESIAN_POINT('Ctrl Pts',(1.75666056638427,1.,-0.164834765707159));
#33522=CARTESIAN_POINT('Ctrl Pts',(1.7472034950333,-1.,-0.163814161002002));
#33523=CARTESIAN_POINT('Ctrl Pts',(1.7472034950333,1.,-0.163814161002002));
#33524=CARTESIAN_POINT('Ctrl Pts',(1.74236521665491,-1.,-0.163289472382896));
#33525=CARTESIAN_POINT('Ctrl Pts',(1.74236521665491,1.,-0.163289472382896));
#33526=CARTESIAN_POINT('',(2.19890268624765,1.,-0.0694764450219582));
#33527=CARTESIAN_POINT('Ctrl Pts',(2.19890268624765,1.,-0.0694764450219582));
#33528=CARTESIAN_POINT('Ctrl Pts',(2.19777582085423,1.,-0.0701143536325491));
#33529=CARTESIAN_POINT('Ctrl Pts',(2.19552129484002,1.,-0.0713863779526155));
#33530=CARTESIAN_POINT('Ctrl Pts',(2.19213712013662,1.,-0.0732830357306726));
#33531=CARTESIAN_POINT('Ctrl Pts',(2.1876201139953,1.,-0.0757891465836149));
#33532=CARTESIAN_POINT('Ctrl Pts',(2.18196589448887,1.,-0.0788837727685244));
#33533=CARTESIAN_POINT('Ctrl Pts',(2.176303712113,1.,-0.0819402680872767));
#33534=CARTESIAN_POINT('Ctrl Pts',(2.17063357870952,1.,-0.0849584620835374));
#33535=CARTESIAN_POINT('Ctrl Pts',(2.16495552645014,1.,-0.0879381291386924));
#33536=CARTESIAN_POINT('Ctrl Pts',(2.15926961544516,1.,-0.0908789888107267));
#33537=CARTESIAN_POINT('Ctrl Pts',(2.1535759397817,1.,-0.0937807218867645));
#33538=CARTESIAN_POINT('Ctrl Pts',(2.14787463531795,1.,-0.096642985230546));
#33539=CARTESIAN_POINT('Ctrl Pts',(2.14216588396025,1.,-0.0994654261990917));
#33540=CARTESIAN_POINT('Ctrl Pts',(2.13644992667165,1.,-0.102247700556101));
#33541=CARTESIAN_POINT('Ctrl Pts',(2.13072704887293,1.,-0.10498947915274));
#33542=CARTESIAN_POINT('Ctrl Pts',(2.12499752307,1.,-0.10769043523109));
#33543=CARTESIAN_POINT('Ctrl Pts',(2.11926155590865,1.,-0.110350236135025));
#33544=CARTESIAN_POINT('Ctrl Pts',(2.11351924490306,1.,-0.112968534419737));
#33545=CARTESIAN_POINT('Ctrl Pts',(2.10777050261309,1.,-0.115544957687927));
#33546=CARTESIAN_POINT('Ctrl Pts',(2.102015121329,1.,-0.118079107988356));
#33547=CARTESIAN_POINT('Ctrl Pts',(2.0962529286773,1.,-0.120570567965122));
#33548=CARTESIAN_POINT('Ctrl Pts',(2.09048392424825,1.,-0.123018905621083));
#33549=CARTESIAN_POINT('Ctrl Pts',(2.08470840653643,1.,-0.125423679412062));
#33550=CARTESIAN_POINT('Ctrl Pts',(2.07892715110987,1.,-0.12778444527612));
#33551=CARTESIAN_POINT('Ctrl Pts',(2.07314114713063,1.,-0.130100748328404));
#33552=CARTESIAN_POINT('Ctrl Pts',(2.06735123910326,1.,-0.132372111547711));
#33553=CARTESIAN_POINT('Ctrl Pts',(2.06155781517842,1.,-0.134598026192106));
#33554=CARTESIAN_POINT('Ctrl Pts',(2.05576044414264,1.,-0.136777941218044));
#33555=CARTESIAN_POINT('Ctrl Pts',(2.04995762001328,1.,-0.138911255368966));
#33556=CARTESIAN_POINT('Ctrl Pts',(2.04414757947916,1.,-0.140997332152546));
#33557=CARTESIAN_POINT('Ctrl Pts',(2.03832911025912,1.,-0.143035515058209));
#33558=CARTESIAN_POINT('Ctrl Pts',(2.03250223739942,1.,-0.145025140186058));
#33559=CARTESIAN_POINT('Ctrl Pts',(2.02666926182017,1.,-0.146965557332583));
#33560=CARTESIAN_POINT('Ctrl Pts',(2.02083464969894,1.,-0.148856124775337));
#33561=CARTESIAN_POINT('Ctrl Pts',(2.01500291940238,1.,-0.150696157673078));
#33562=CARTESIAN_POINT('Ctrl Pts',(2.00917680318424,1.,-0.15248488362145));
#33563=CARTESIAN_POINT('Ctrl Pts',(2.00335565310543,1.,-0.154221403049722));
#33564=CARTESIAN_POINT('Ctrl Pts',(1.99753284771497,1.,-0.155904629548784));
#33565=CARTESIAN_POINT('Ctrl Pts',(1.99169810931908,1.,-0.157533331459227));
#33566=CARTESIAN_POINT('Ctrl Pts',(1.98584238283292,1.,-0.159106226437299));
#33567=CARTESIAN_POINT('Ctrl Pts',(1.97996195437559,1.,-0.160622060784611));
#33568=CARTESIAN_POINT('Ctrl Pts',(1.97406280235188,1.,-0.162079693556289));
#33569=CARTESIAN_POINT('Ctrl Pts',(1.96816512677967,1.,-0.163478185457734));
#33570=CARTESIAN_POINT('Ctrl Pts',(1.96229379940136,1.,-0.164816568920269));
#33571=CARTESIAN_POINT('Ctrl Pts',(1.9564675971873,1.,-0.166093592002813));
#33572=CARTESIAN_POINT('Ctrl Pts',(1.95069027794294,1.,-0.167307501784476));
#33573=CARTESIAN_POINT('Ctrl Pts',(1.94493757756931,1.,-0.168455741607556));
#33574=CARTESIAN_POINT('Ctrl Pts',(1.93915639211581,1.,-0.169534904817491));
#33575=CARTESIAN_POINT('Ctrl Pts',(1.93329183155539,1.,-0.170541253116202));
#33576=CARTESIAN_POINT('Ctrl Pts',(1.92731093582036,1.,-0.171471191532988));
#33577=CARTESIAN_POINT('Ctrl Pts',(1.9212233439798,1.,-0.172321621259514));
#33578=CARTESIAN_POINT('Ctrl Pts',(1.91511429159527,1.,-0.173090695383496));
#33579=CARTESIAN_POINT('Ctrl Pts',(1.90911693975267,1.,-0.173776635257817));
#33580=CARTESIAN_POINT('Ctrl Pts',(1.90335253862834,1.,-0.174375518661085));
#33581=CARTESIAN_POINT('Ctrl Pts',(1.89788101117132,1.,-0.174879405091263));
#33582=CARTESIAN_POINT('Ctrl Pts',(1.892646301985,1.,-0.175274276190844));
#33583=CARTESIAN_POINT('Ctrl Pts',(1.88742606273259,1.,-0.175538155840648));
#33584=CARTESIAN_POINT('Ctrl Pts',(1.88188663145367,1.,-0.175644148889699));
#33585=CARTESIAN_POINT('Ctrl Pts',(1.87563767773588,1.,-0.175563480746485));
#33586=CARTESIAN_POINT('Ctrl Pts',(1.86828349694799,1.,-0.175268337590758));
#33587=CARTESIAN_POINT('Ctrl Pts',(1.85948367088837,1.,-0.17473525927603));
#33588=CARTESIAN_POINT('Ctrl Pts',(1.8489811319852,1.,-0.173946627587732));
#33589=CARTESIAN_POINT('Ctrl Pts',(1.83658380527692,1.,-0.1728894428919));
#33590=CARTESIAN_POINT('Ctrl Pts',(1.82215766811545,1.,-0.171554770204119));
#33591=CARTESIAN_POINT('Ctrl Pts',(1.80561530629706,1.,-0.169936923904608));
#33592=CARTESIAN_POINT('Ctrl Pts',(1.7869064998507,1.,-0.168032772805197));
#33593=CARTESIAN_POINT('Ctrl Pts',(1.77018771684844,1.,-0.1662793551464));
#33594=CARTESIAN_POINT('Ctrl Pts',(1.75666056638427,1.,-0.164834765707159));
#33595=CARTESIAN_POINT('Ctrl Pts',(1.7472034950333,1.,-0.163814161002002));
#33596=CARTESIAN_POINT('Ctrl Pts',(1.74236521665491,1.,-0.163289472382896));
#33597=CARTESIAN_POINT('',(2.19890268624765,0.,-0.0694764450219582));
#33598=CARTESIAN_POINT('Origin',(2.19890268624765,0.,0.0694764450219582));
#33599=CARTESIAN_POINT('',(2.19890268624765,1.,0.0694764450219582));
#33600=CARTESIAN_POINT('',(2.19890268624765,1.,-0.0694764450219582));
#33601=CARTESIAN_POINT('',(2.19890268624765,0.,0.0694764450219582));
#33602=CARTESIAN_POINT('Ctrl Pts',(1.74236521665491,-1.,0.163289472382896));
#33603=CARTESIAN_POINT('Ctrl Pts',(1.74236521665491,1.,0.163289472382896));
#33604=CARTESIAN_POINT('Ctrl Pts',(1.74720349503904,-1.,0.163814161002474));
#33605=CARTESIAN_POINT('Ctrl Pts',(1.74720349503904,1.,0.163814161002474));
#33606=CARTESIAN_POINT('Ctrl Pts',(1.75666056640041,-1.,0.164834765708484));
#33607=CARTESIAN_POINT('Ctrl Pts',(1.75666056640041,1.,0.164834765708484));
#33608=CARTESIAN_POINT('Ctrl Pts',(1.77018771687692,-1.,0.166279355148738));
#33609=CARTESIAN_POINT('Ctrl Pts',(1.77018771687692,1.,0.166279355148738));
#33610=CARTESIAN_POINT('Ctrl Pts',(1.78690649988931,-1.,0.16803277280837));
#33611=CARTESIAN_POINT('Ctrl Pts',(1.78690649988931,1.,0.16803277280837));
#33612=CARTESIAN_POINT('Ctrl Pts',(1.80561530633924,-1.,0.169936923908078));
#33613=CARTESIAN_POINT('Ctrl Pts',(1.80561530633924,1.,0.169936923908078));
#33614=CARTESIAN_POINT('Ctrl Pts',(1.82215766815414,-1.,0.171554770207306));
#33615=CARTESIAN_POINT('Ctrl Pts',(1.82215766815414,1.,0.171554770207306));
#33616=CARTESIAN_POINT('Ctrl Pts',(1.83658380530747,-1.,0.17288944289442));
#33617=CARTESIAN_POINT('Ctrl Pts',(1.83658380530747,1.,0.17288944289442));
#33618=CARTESIAN_POINT('Ctrl Pts',(1.84898113200543,-1.,0.173946627589401));
#33619=CARTESIAN_POINT('Ctrl Pts',(1.84898113200543,1.,0.173946627589401));
#33620=CARTESIAN_POINT('Ctrl Pts',(1.85948367089838,-1.,0.174735259276856));
#33621=CARTESIAN_POINT('Ctrl Pts',(1.85948367089838,1.,0.174735259276856));
#33622=CARTESIAN_POINT('Ctrl Pts',(1.86828349694972,-1.,0.1752683375909));
#33623=CARTESIAN_POINT('Ctrl Pts',(1.86828349694972,1.,0.1752683375909));
#33624=CARTESIAN_POINT('Ctrl Pts',(1.87563767773249,-1.,0.175563480746205));
#33625=CARTESIAN_POINT('Ctrl Pts',(1.87563767773249,1.,0.175563480746205));
#33626=CARTESIAN_POINT('Ctrl Pts',(1.88188663144846,-1.,0.175644148889271));
#33627=CARTESIAN_POINT('Ctrl Pts',(1.88188663144846,1.,0.175644148889271));
#33628=CARTESIAN_POINT('Ctrl Pts',(1.88742606272818,-1.,0.175538155840286));
#33629=CARTESIAN_POINT('Ctrl Pts',(1.88742606272818,1.,0.175538155840286));
#33630=CARTESIAN_POINT('Ctrl Pts',(1.89264630198279,-1.,0.175274276190664));
#33631=CARTESIAN_POINT('Ctrl Pts',(1.89264630198279,1.,0.175274276190664));
#33632=CARTESIAN_POINT('Ctrl Pts',(1.89788101117148,-1.,0.174879405091277));
#33633=CARTESIAN_POINT('Ctrl Pts',(1.89788101117148,1.,0.174879405091277));
#33634=CARTESIAN_POINT('Ctrl Pts',(1.90335253863003,-1.,0.174375518661222));
#33635=CARTESIAN_POINT('Ctrl Pts',(1.90335253863003,1.,0.174375518661222));
#33636=CARTESIAN_POINT('Ctrl Pts',(1.90911693975475,-1.,0.173776635257983));
#33637=CARTESIAN_POINT('Ctrl Pts',(1.90911693975475,1.,0.173776635257983));
#33638=CARTESIAN_POINT('Ctrl Pts',(1.91511429159681,-1.,0.173090695383619));
#33639=CARTESIAN_POINT('Ctrl Pts',(1.91511429159681,1.,0.173090695383619));
#33640=CARTESIAN_POINT('Ctrl Pts',(1.92122334398034,-1.,0.172321621259556));
#33641=CARTESIAN_POINT('Ctrl Pts',(1.92122334398034,1.,0.172321621259556));
#33642=CARTESIAN_POINT('Ctrl Pts',(1.92731093582,-1.,0.17147119153296));
#33643=CARTESIAN_POINT('Ctrl Pts',(1.92731093582,1.,0.17147119153296));
#33644=CARTESIAN_POINT('Ctrl Pts',(1.93329183155455,-1.,0.170541253116136));
#33645=CARTESIAN_POINT('Ctrl Pts',(1.93329183155455,1.,0.170541253116136));
#33646=CARTESIAN_POINT('Ctrl Pts',(1.93915639211497,-1.,0.169534904817425));
#33647=CARTESIAN_POINT('Ctrl Pts',(1.93915639211497,1.,0.169534904817425));
#33648=CARTESIAN_POINT('Ctrl Pts',(1.94493757756879,-1.,0.168455741607515));
#33649=CARTESIAN_POINT('Ctrl Pts',(1.94493757756879,1.,0.168455741607515));
#33650=CARTESIAN_POINT('Ctrl Pts',(1.95069027794286,-1.,0.167307501784469));
#33651=CARTESIAN_POINT('Ctrl Pts',(1.95069027794286,1.,0.167307501784469));
#33652=CARTESIAN_POINT('Ctrl Pts',(1.95646759718755,-1.,0.166093592002832));
#33653=CARTESIAN_POINT('Ctrl Pts',(1.95646759718755,1.,0.166093592002832));
#33654=CARTESIAN_POINT('Ctrl Pts',(1.96229379940174,-1.,0.1648165689203));
#33655=CARTESIAN_POINT('Ctrl Pts',(1.96229379940174,1.,0.1648165689203));
#33656=CARTESIAN_POINT('Ctrl Pts',(1.96816512678,-1.,0.16347818545776));
#33657=CARTESIAN_POINT('Ctrl Pts',(1.96816512678,1.,0.16347818545776));
#33658=CARTESIAN_POINT('Ctrl Pts',(1.97406280235204,-1.,0.162079693556302));
#33659=CARTESIAN_POINT('Ctrl Pts',(1.97406280235204,1.,0.162079693556302));
#33660=CARTESIAN_POINT('Ctrl Pts',(1.97996195437557,-1.,0.16062206078461));
#33661=CARTESIAN_POINT('Ctrl Pts',(1.97996195437557,1.,0.16062206078461));
#33662=CARTESIAN_POINT('Ctrl Pts',(1.98584238283279,-1.,0.159106226437288));
#33663=CARTESIAN_POINT('Ctrl Pts',(1.98584238283279,1.,0.159106226437288));
#33664=CARTESIAN_POINT('Ctrl Pts',(1.99169810931893,-1.,0.157533331459215));
#33665=CARTESIAN_POINT('Ctrl Pts',(1.99169810931893,1.,0.157533331459215));
#33666=CARTESIAN_POINT('Ctrl Pts',(1.99753284771487,-1.,0.155904629548774));
#33667=CARTESIAN_POINT('Ctrl Pts',(1.99753284771487,1.,0.155904629548774));
#33668=CARTESIAN_POINT('Ctrl Pts',(2.00335565310539,-1.,0.154221403049719));
#33669=CARTESIAN_POINT('Ctrl Pts',(2.00335565310539,1.,0.154221403049719));
#33670=CARTESIAN_POINT('Ctrl Pts',(2.00917680318426,-1.,0.152484883621452));
#33671=CARTESIAN_POINT('Ctrl Pts',(2.00917680318426,1.,0.152484883621452));
#33672=CARTESIAN_POINT('Ctrl Pts',(2.01500291940243,-1.,0.150696157673084));
#33673=CARTESIAN_POINT('Ctrl Pts',(2.01500291940243,1.,0.150696157673084));
#33674=CARTESIAN_POINT('Ctrl Pts',(2.02083464969897,-1.,0.148856124775342));
#33675=CARTESIAN_POINT('Ctrl Pts',(2.02083464969897,1.,0.148856124775342));
#33676=CARTESIAN_POINT('Ctrl Pts',(2.02666926182017,-1.,0.146965557332586));
#33677=CARTESIAN_POINT('Ctrl Pts',(2.02666926182017,1.,0.146965557332586));
#33678=CARTESIAN_POINT('Ctrl Pts',(2.03250223739941,-1.,0.145025140186058));
#33679=CARTESIAN_POINT('Ctrl Pts',(2.03250223739941,1.,0.145025140186058));
#33680=CARTESIAN_POINT('Ctrl Pts',(2.03832911025913,-1.,0.143035515058208));
#33681=CARTESIAN_POINT('Ctrl Pts',(2.03832911025913,1.,0.143035515058208));
#33682=CARTESIAN_POINT('Ctrl Pts',(2.04414757947919,-1.,0.140997332152545));
#33683=CARTESIAN_POINT('Ctrl Pts',(2.04414757947919,1.,0.140997332152545));
#33684=CARTESIAN_POINT('Ctrl Pts',(2.04995762001333,-1.,0.138911255368966));
#33685=CARTESIAN_POINT('Ctrl Pts',(2.04995762001333,1.,0.138911255368966));
#33686=CARTESIAN_POINT('Ctrl Pts',(2.0557604441427,-1.,0.136777941218044));
#33687=CARTESIAN_POINT('Ctrl Pts',(2.0557604441427,1.,0.136777941218044));
#33688=CARTESIAN_POINT('Ctrl Pts',(2.06155781517844,-1.,0.134598026192107));
#33689=CARTESIAN_POINT('Ctrl Pts',(2.06155781517844,1.,0.134598026192107));
#33690=CARTESIAN_POINT('Ctrl Pts',(2.06735123910319,-1.,0.132372111547709));
#33691=CARTESIAN_POINT('Ctrl Pts',(2.06735123910319,1.,0.132372111547709));
#33692=CARTESIAN_POINT('Ctrl Pts',(2.07314114713047,-1.,0.1301007483284));
#33693=CARTESIAN_POINT('Ctrl Pts',(2.07314114713047,1.,0.1301007483284));
#33694=CARTESIAN_POINT('Ctrl Pts',(2.07892715110967,-1.,0.127784445276116));
#33695=CARTESIAN_POINT('Ctrl Pts',(2.07892715110967,1.,0.127784445276116));
#33696=CARTESIAN_POINT('Ctrl Pts',(2.08470840653628,-1.,0.125423679412058));
#33697=CARTESIAN_POINT('Ctrl Pts',(2.08470840653628,1.,0.125423679412058));
#33698=CARTESIAN_POINT('Ctrl Pts',(2.09048392424826,-1.,0.123018905621083));
#33699=CARTESIAN_POINT('Ctrl Pts',(2.09048392424826,1.,0.123018905621083));
#33700=CARTESIAN_POINT('Ctrl Pts',(2.09625292867756,-1.,0.120570567965129));
#33701=CARTESIAN_POINT('Ctrl Pts',(2.09625292867756,1.,0.120570567965129));
#33702=CARTESIAN_POINT('Ctrl Pts',(2.10201512132945,-1.,0.118079107988368));
#33703=CARTESIAN_POINT('Ctrl Pts',(2.10201512132945,1.,0.118079107988368));
#33704=CARTESIAN_POINT('Ctrl Pts',(2.10777050261359,-1.,0.11554495768794));
#33705=CARTESIAN_POINT('Ctrl Pts',(2.10777050261359,1.,0.11554495768794));
#33706=CARTESIAN_POINT('Ctrl Pts',(2.11351924490335,-1.,0.112968534419746));
#33707=CARTESIAN_POINT('Ctrl Pts',(2.11351924490335,1.,0.112968534419746));
#33708=CARTESIAN_POINT('Ctrl Pts',(2.11926155590849,-1.,0.11035023613502));
#33709=CARTESIAN_POINT('Ctrl Pts',(2.11926155590849,1.,0.11035023613502));
#33710=CARTESIAN_POINT('Ctrl Pts',(2.12499752306927,-1.,0.107690435231068));
#33711=CARTESIAN_POINT('Ctrl Pts',(2.12499752306927,1.,0.107690435231068));
#33712=CARTESIAN_POINT('Ctrl Pts',(2.1307270488718,-1.,0.104989479152703));
#33713=CARTESIAN_POINT('Ctrl Pts',(2.1307270488718,1.,0.104989479152703));
#33714=CARTESIAN_POINT('Ctrl Pts',(2.13644992667052,-1.,0.102247700556063));
#33715=CARTESIAN_POINT('Ctrl Pts',(2.13644992667052,1.,0.102247700556063));
#33716=CARTESIAN_POINT('Ctrl Pts',(2.14216588395974,-1.,0.0994654261990741));
#33717=CARTESIAN_POINT('Ctrl Pts',(2.14216588395974,1.,0.0994654261990741));
#33718=CARTESIAN_POINT('Ctrl Pts',(2.14787463531864,-1.,0.0966429852305688));
#33719=CARTESIAN_POINT('Ctrl Pts',(2.14787463531864,1.,0.0966429852305688));
#33720=CARTESIAN_POINT('Ctrl Pts',(2.15357593978377,-1.,0.0937807218868344));
#33721=CARTESIAN_POINT('Ctrl Pts',(2.15357593978377,1.,0.0937807218868344));
#33722=CARTESIAN_POINT('Ctrl Pts',(2.15926961544808,-1.,0.0908789888108265));
#33723=CARTESIAN_POINT('Ctrl Pts',(2.15926961544808,1.,0.0908789888108265));
#33724=CARTESIAN_POINT('Ctrl Pts',(2.16495552645275,-1.,0.0879381291387821));
#33725=CARTESIAN_POINT('Ctrl Pts',(2.16495552645275,1.,0.0879381291387821));
#33726=CARTESIAN_POINT('Ctrl Pts',(2.17063357871031,-1.,0.0849584620835642));
#33727=CARTESIAN_POINT('Ctrl Pts',(2.17063357871031,1.,0.0849584620835642));
#33728=CARTESIAN_POINT('Ctrl Pts',(2.1763037121106,-1.,0.0819402680871938));
#33729=CARTESIAN_POINT('Ctrl Pts',(2.1763037121106,1.,0.0819402680871938));
#33730=CARTESIAN_POINT('Ctrl Pts',(2.18196589448304,-1.,0.0788837727683226));
#33731=CARTESIAN_POINT('Ctrl Pts',(2.18196589448304,1.,0.0788837727683226));
#33732=CARTESIAN_POINT('Ctrl Pts',(2.1876201139874,-1.,0.075789146583341));
#33733=CARTESIAN_POINT('Ctrl Pts',(2.1876201139874,1.,0.075789146583341));
#33734=CARTESIAN_POINT('Ctrl Pts',(2.19213712012956,-1.,0.0732830357304275));
#33735=CARTESIAN_POINT('Ctrl Pts',(2.19213712012956,1.,0.0732830357304275));
#33736=CARTESIAN_POINT('Ctrl Pts',(2.19552129483562,-1.,0.0713863779524626));
#33737=CARTESIAN_POINT('Ctrl Pts',(2.19552129483562,1.,0.0713863779524626));
#33738=CARTESIAN_POINT('Ctrl Pts',(2.19777582085261,-1.,0.0701143536324925));
#33739=CARTESIAN_POINT('Ctrl Pts',(2.19777582085261,1.,0.0701143536324925));
#33740=CARTESIAN_POINT('Ctrl Pts',(2.19890268624765,-1.,0.0694764450219582));
#33741=CARTESIAN_POINT('Ctrl Pts',(2.19890268624765,1.,0.0694764450219582));
#33742=CARTESIAN_POINT('',(1.74236521665491,1.,0.163289472382896));
#33743=CARTESIAN_POINT('Ctrl Pts',(1.74236521665491,1.,0.163289472382896));
#33744=CARTESIAN_POINT('Ctrl Pts',(1.74720349503904,1.,0.163814161002474));
#33745=CARTESIAN_POINT('Ctrl Pts',(1.75666056640041,1.,0.164834765708484));
#33746=CARTESIAN_POINT('Ctrl Pts',(1.77018771687692,1.,0.166279355148738));
#33747=CARTESIAN_POINT('Ctrl Pts',(1.78690649988931,1.,0.16803277280837));
#33748=CARTESIAN_POINT('Ctrl Pts',(1.80561530633924,1.,0.169936923908078));
#33749=CARTESIAN_POINT('Ctrl Pts',(1.82215766815414,1.,0.171554770207306));
#33750=CARTESIAN_POINT('Ctrl Pts',(1.83658380530747,1.,0.17288944289442));
#33751=CARTESIAN_POINT('Ctrl Pts',(1.84898113200543,1.,0.173946627589401));
#33752=CARTESIAN_POINT('Ctrl Pts',(1.85948367089838,1.,0.174735259276856));
#33753=CARTESIAN_POINT('Ctrl Pts',(1.86828349694972,1.,0.1752683375909));
#33754=CARTESIAN_POINT('Ctrl Pts',(1.87563767773249,1.,0.175563480746205));
#33755=CARTESIAN_POINT('Ctrl Pts',(1.88188663144846,1.,0.175644148889271));
#33756=CARTESIAN_POINT('Ctrl Pts',(1.88742606272818,1.,0.175538155840286));
#33757=CARTESIAN_POINT('Ctrl Pts',(1.89264630198279,1.,0.175274276190664));
#33758=CARTESIAN_POINT('Ctrl Pts',(1.89788101117148,1.,0.174879405091277));
#33759=CARTESIAN_POINT('Ctrl Pts',(1.90335253863003,1.,0.174375518661222));
#33760=CARTESIAN_POINT('Ctrl Pts',(1.90911693975475,1.,0.173776635257983));
#33761=CARTESIAN_POINT('Ctrl Pts',(1.91511429159681,1.,0.173090695383619));
#33762=CARTESIAN_POINT('Ctrl Pts',(1.92122334398034,1.,0.172321621259556));
#33763=CARTESIAN_POINT('Ctrl Pts',(1.92731093582,1.,0.17147119153296));
#33764=CARTESIAN_POINT('Ctrl Pts',(1.93329183155455,1.,0.170541253116136));
#33765=CARTESIAN_POINT('Ctrl Pts',(1.93915639211497,1.,0.169534904817425));
#33766=CARTESIAN_POINT('Ctrl Pts',(1.94493757756879,1.,0.168455741607515));
#33767=CARTESIAN_POINT('Ctrl Pts',(1.95069027794286,1.,0.167307501784469));
#33768=CARTESIAN_POINT('Ctrl Pts',(1.95646759718755,1.,0.166093592002832));
#33769=CARTESIAN_POINT('Ctrl Pts',(1.96229379940174,1.,0.1648165689203));
#33770=CARTESIAN_POINT('Ctrl Pts',(1.96816512678,1.,0.16347818545776));
#33771=CARTESIAN_POINT('Ctrl Pts',(1.97406280235204,1.,0.162079693556302));
#33772=CARTESIAN_POINT('Ctrl Pts',(1.97996195437557,1.,0.16062206078461));
#33773=CARTESIAN_POINT('Ctrl Pts',(1.98584238283279,1.,0.159106226437288));
#33774=CARTESIAN_POINT('Ctrl Pts',(1.99169810931893,1.,0.157533331459215));
#33775=CARTESIAN_POINT('Ctrl Pts',(1.99753284771487,1.,0.155904629548774));
#33776=CARTESIAN_POINT('Ctrl Pts',(2.00335565310539,1.,0.154221403049719));
#33777=CARTESIAN_POINT('Ctrl Pts',(2.00917680318426,1.,0.152484883621452));
#33778=CARTESIAN_POINT('Ctrl Pts',(2.01500291940243,1.,0.150696157673084));
#33779=CARTESIAN_POINT('Ctrl Pts',(2.02083464969897,1.,0.148856124775342));
#33780=CARTESIAN_POINT('Ctrl Pts',(2.02666926182017,1.,0.146965557332586));
#33781=CARTESIAN_POINT('Ctrl Pts',(2.03250223739941,1.,0.145025140186058));
#33782=CARTESIAN_POINT('Ctrl Pts',(2.03832911025913,1.,0.143035515058208));
#33783=CARTESIAN_POINT('Ctrl Pts',(2.04414757947919,1.,0.140997332152545));
#33784=CARTESIAN_POINT('Ctrl Pts',(2.04995762001333,1.,0.138911255368966));
#33785=CARTESIAN_POINT('Ctrl Pts',(2.0557604441427,1.,0.136777941218044));
#33786=CARTESIAN_POINT('Ctrl Pts',(2.06155781517844,1.,0.134598026192107));
#33787=CARTESIAN_POINT('Ctrl Pts',(2.06735123910319,1.,0.132372111547709));
#33788=CARTESIAN_POINT('Ctrl Pts',(2.07314114713047,1.,0.1301007483284));
#33789=CARTESIAN_POINT('Ctrl Pts',(2.07892715110967,1.,0.127784445276116));
#33790=CARTESIAN_POINT('Ctrl Pts',(2.08470840653628,1.,0.125423679412058));
#33791=CARTESIAN_POINT('Ctrl Pts',(2.09048392424826,1.,0.123018905621083));
#33792=CARTESIAN_POINT('Ctrl Pts',(2.09625292867756,1.,0.120570567965129));
#33793=CARTESIAN_POINT('Ctrl Pts',(2.10201512132945,1.,0.118079107988368));
#33794=CARTESIAN_POINT('Ctrl Pts',(2.10777050261359,1.,0.11554495768794));
#33795=CARTESIAN_POINT('Ctrl Pts',(2.11351924490335,1.,0.112968534419746));
#33796=CARTESIAN_POINT('Ctrl Pts',(2.11926155590849,1.,0.11035023613502));
#33797=CARTESIAN_POINT('Ctrl Pts',(2.12499752306927,1.,0.107690435231068));
#33798=CARTESIAN_POINT('Ctrl Pts',(2.1307270488718,1.,0.104989479152703));
#33799=CARTESIAN_POINT('Ctrl Pts',(2.13644992667052,1.,0.102247700556063));
#33800=CARTESIAN_POINT('Ctrl Pts',(2.14216588395974,1.,0.0994654261990741));
#33801=CARTESIAN_POINT('Ctrl Pts',(2.14787463531864,1.,0.0966429852305688));
#33802=CARTESIAN_POINT('Ctrl Pts',(2.15357593978377,1.,0.0937807218868344));
#33803=CARTESIAN_POINT('Ctrl Pts',(2.15926961544808,1.,0.0908789888108265));
#33804=CARTESIAN_POINT('Ctrl Pts',(2.16495552645275,1.,0.0879381291387821));
#33805=CARTESIAN_POINT('Ctrl Pts',(2.17063357871031,1.,0.0849584620835642));
#33806=CARTESIAN_POINT('Ctrl Pts',(2.1763037121106,1.,0.0819402680871938));
#33807=CARTESIAN_POINT('Ctrl Pts',(2.18196589448304,1.,0.0788837727683226));
#33808=CARTESIAN_POINT('Ctrl Pts',(2.1876201139874,1.,0.075789146583341));
#33809=CARTESIAN_POINT('Ctrl Pts',(2.19213712012956,1.,0.0732830357304275));
#33810=CARTESIAN_POINT('Ctrl Pts',(2.19552129483562,1.,0.0713863779524626));
#33811=CARTESIAN_POINT('Ctrl Pts',(2.19777582085261,1.,0.0701143536324925));
#33812=CARTESIAN_POINT('Ctrl Pts',(2.19890268624765,1.,0.0694764450219582));
#33813=CARTESIAN_POINT('',(1.74236521665491,0.,0.163289472382896));
#33814=CARTESIAN_POINT('Origin',(0.,1.,0.));
#33815=CARTESIAN_POINT('Origin',(0.,1.,0.));
#33816=CARTESIAN_POINT('Origin',(0.,0.,0.));
#57830=UNCERTAINTY_MEASURE_WITH_UNIT(LENGTH_MEASURE(0.001),#57901,
'DISTANCE_ACCURACY_VALUE',
'Maximum model space distance between geometric entities at asserted c
onnectivities');
#57841=UNCERTAINTY_MEASURE_WITH_UNIT(LENGTH_MEASURE(0.001),#57901,
'DISTANCE_ACCURACY_VALUE',
'Maximum model space distance between geometric entities at asserted c
onnectivities');
#57889=(
GEOMETRIC_REPRESENTATION_CONTEXT(3)
GLOBAL_UNCERTAINTY_ASSIGNED_CONTEXT((#57830))
GLOBAL_UNIT_ASSIGNED_CONTEXT((#57901,#57903,#57904))
REPRESENTATION_CONTEXT('','3D')
);
#57900=(
GEOMETRIC_REPRESENTATION_CONTEXT(3)
GLOBAL_UNCERTAINTY_ASSIGNED_CONTEXT((#57841))
GLOBAL_UNIT_ASSIGNED_CONTEXT((#57901,#57903,#57904))
REPRESENTATION_CONTEXT('','3D')
);
#57901=(
LENGTH_UNIT()
NAMED_UNIT(*)
SI_UNIT(.CENTI.,.METRE.)
);
#57903=(
NAMED_UNIT(*)
PLANE_ANGLE_UNIT()
SI_UNIT($,.RADIAN.)
);
#57904=(
NAMED_UNIT(*)
SI_UNIT($,.STERADIAN.)
SOLID_ANGLE_UNIT()
);
#57952=SHAPE_DEFINITION_REPRESENTATION(#58023,#58156);
#58023=PRODUCT_DEFINITION_SHAPE('',$,#58215);
#58156=SHAPE_REPRESENTATION('',(#15128),#57889);
#58167=PRODUCT_DEFINITION_CONTEXT('part definition',#58343,'design');
#58215=PRODUCT_DEFINITION('Spur Gear - Module 2, 20 Teeth, 12 mm Bore',
'Spur Gear - Module 2, 20 Teeth, 12 mm Bore',#58273,#58167);
#58273=PRODUCT_DEFINITION_FORMATION('',$,#58392);
#58343=APPLICATION_CONTEXT(
'Core Data for Automotive Mechanical Design Process');
#58344=PRODUCT_CONTEXT('part definition',#58343,'mechanical');
#58392=PRODUCT('Spur Gear - Module 2, 20 Teeth, 12 mm Bore',
'Spur Gear - Module 2, 20 Teeth, 12 mm Bore',
'Spur Gear - Module 2, 20 Teeth, 12 mm Bore',(#58344));
#58473=COLOUR_RGB('Off White',0.89,0.88,0.83);
#58474=FILL_AREA_STYLE_COLOUR('',#58473);
#58475=FILL_AREA_STYLE('',(#58474));
#58476=SURFACE_STYLE_FILL_AREA(#58475);
#58477=SURFACE_SIDE_STYLE('',(#58476));
#58478=SURFACE_STYLE_USAGE(.BOTH.,#58477);
#58479=PRESENTATION_STYLE_ASSIGNMENT((#58478));
ENDSEC;
END-ISO-10303-21;
